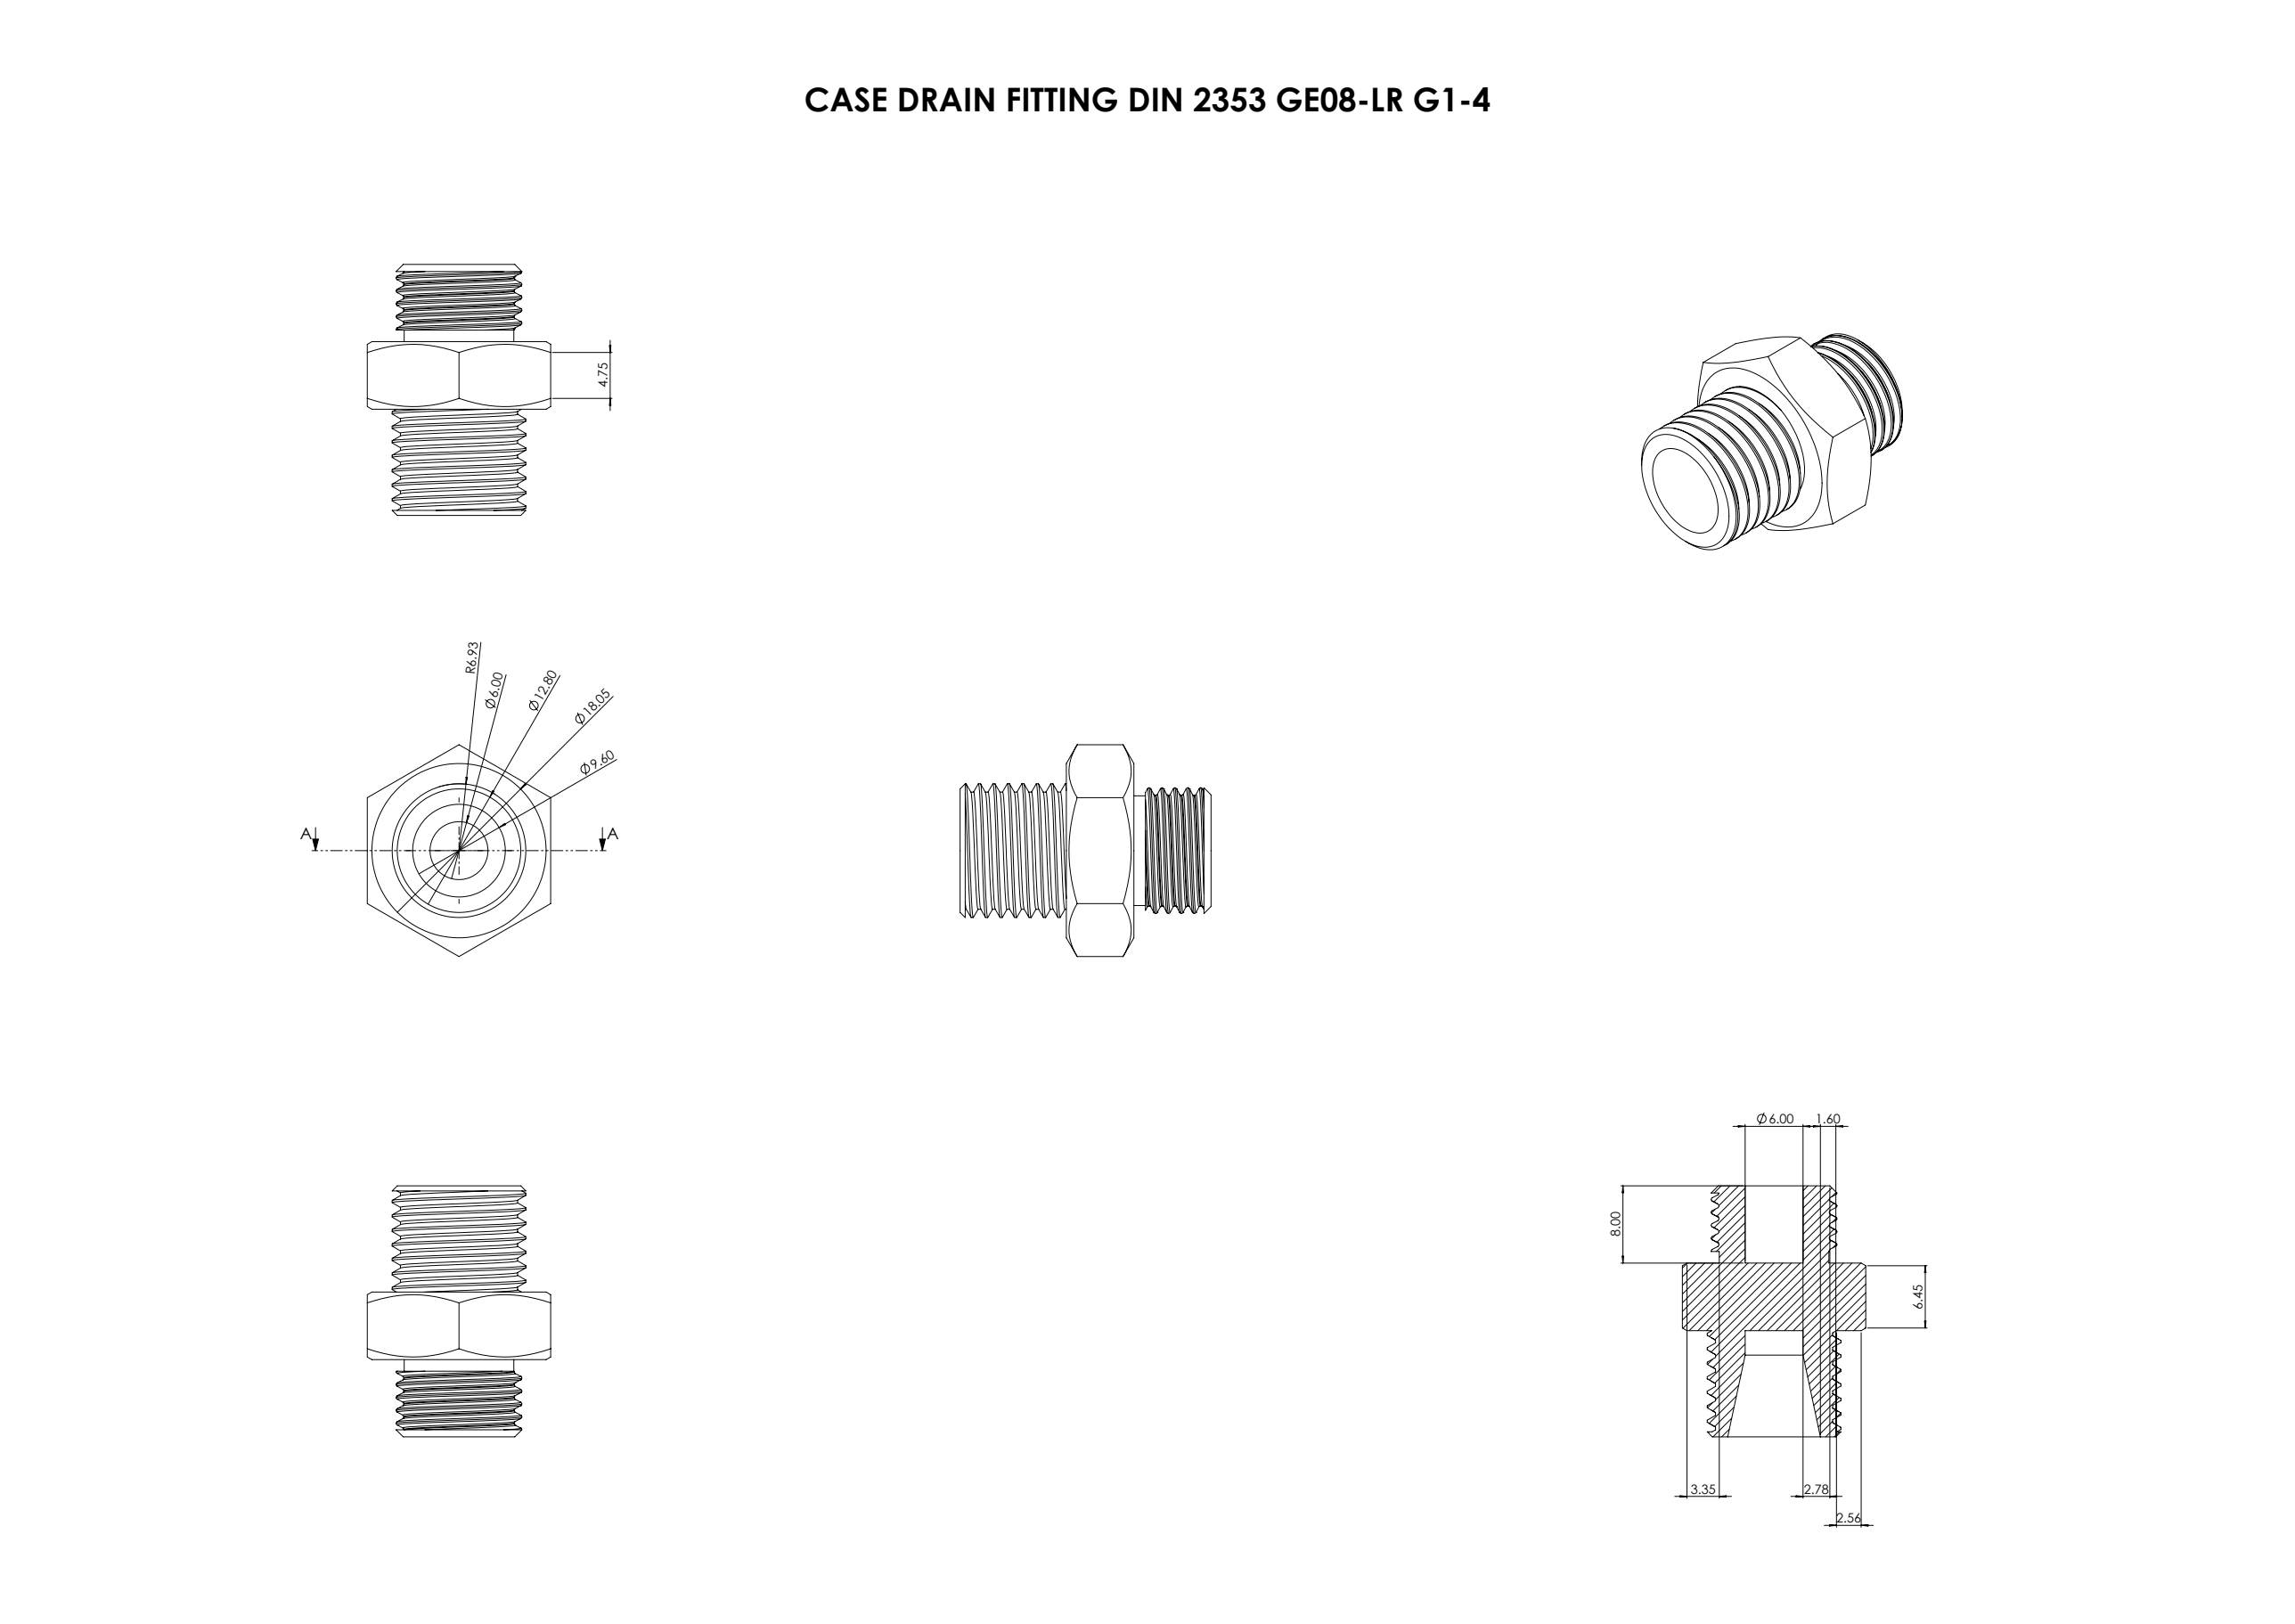
ISO-10303-21;
HEADER;
/* Generated by software containing ST-Developer
 * from STEP Tools, Inc. (www.steptools.com) 
 */

FILE_DESCRIPTION(
/* description */ (''),
/* implementation_level */ '2;1');

FILE_NAME(
/* name */ '19_Case_Drain_Fitting_DIN_2353_GE08-LR_G1-4.step',
/* time_stamp */ '2026-10-23T00:52:27+05:00',
/* author */ (''),
/* organization */ (''),
/* preprocessor_version */ 'ST-DEVELOPER v20.2',
/* originating_system */ 'Autodesk Translation Framework v15.15.0.0',
/* authorisation */ '');

FILE_SCHEMA (('AUTOMOTIVE_DESIGN { 1 0 10303 214 3 1 1 }'));
ENDSEC;

DATA;
#10=MECHANICAL_DESIGN_GEOMETRIC_PRESENTATION_REPRESENTATION('',(#1555),#59204);
#324=B_SPLINE_SURFACE_WITH_KNOTS('',3,3,((#38272,#38273,#38274,#38275,#38276,
#38277,#38278,#38279,#38280,#38281,#38282,#38283,#38284,#38285,#38286,#38287,
#38288,#38289,#38290,#38291,#38292,#38293,#38294,#38295,#38296,#38297,#38298,
#38299,#38300,#38301,#38302,#38303,#38304,#38305,#38306,#38307,#38308,#38309,
#38310,#38311,#38312,#38313,#38314,#38315,#38316,#38317,#38318,#38319,#38320,
#38321,#38322,#38323,#38324,#38325,#38326,#38327,#38328,#38329,#38330,#38331,
#38332,#38333,#38334,#38335,#38336,#38337,#38338,#38339,#38340,#38341,#38342,
#38343,#38344,#38345,#38346,#38347,#38348,#38349,#38350,#38351,#38352,#38353,
#38354,#38355,#38356,#38357,#38358,#38359,#38360,#38361,#38362,#38363,#38364,
#38365,#38366),(#38367,#38368,#38369,#38370,#38371,#38372,#38373,#38374,
#38375,#38376,#38377,#38378,#38379,#38380,#38381,#38382,#38383,#38384,#38385,
#38386,#38387,#38388,#38389,#38390,#38391,#38392,#38393,#38394,#38395,#38396,
#38397,#38398,#38399,#38400,#38401,#38402,#38403,#38404,#38405,#38406,#38407,
#38408,#38409,#38410,#38411,#38412,#38413,#38414,#38415,#38416,#38417,#38418,
#38419,#38420,#38421,#38422,#38423,#38424,#38425,#38426,#38427,#38428,#38429,
#38430,#38431,#38432,#38433,#38434,#38435,#38436,#38437,#38438,#38439,#38440,
#38441,#38442,#38443,#38444,#38445,#38446,#38447,#38448,#38449,#38450,#38451,
#38452,#38453,#38454,#38455,#38456,#38457,#38458,#38459,#38460,#38461),
(#38462,#38463,#38464,#38465,#38466,#38467,#38468,#38469,#38470,#38471,
#38472,#38473,#38474,#38475,#38476,#38477,#38478,#38479,#38480,#38481,#38482,
#38483,#38484,#38485,#38486,#38487,#38488,#38489,#38490,#38491,#38492,#38493,
#38494,#38495,#38496,#38497,#38498,#38499,#38500,#38501,#38502,#38503,#38504,
#38505,#38506,#38507,#38508,#38509,#38510,#38511,#38512,#38513,#38514,#38515,
#38516,#38517,#38518,#38519,#38520,#38521,#38522,#38523,#38524,#38525,#38526,
#38527,#38528,#38529,#38530,#38531,#38532,#38533,#38534,#38535,#38536,#38537,
#38538,#38539,#38540,#38541,#38542,#38543,#38544,#38545,#38546,#38547,#38548,
#38549,#38550,#38551,#38552,#38553,#38554,#38555,#38556),(#38557,#38558,
#38559,#38560,#38561,#38562,#38563,#38564,#38565,#38566,#38567,#38568,#38569,
#38570,#38571,#38572,#38573,#38574,#38575,#38576,#38577,#38578,#38579,#38580,
#38581,#38582,#38583,#38584,#38585,#38586,#38587,#38588,#38589,#38590,#38591,
#38592,#38593,#38594,#38595,#38596,#38597,#38598,#38599,#38600,#38601,#38602,
#38603,#38604,#38605,#38606,#38607,#38608,#38609,#38610,#38611,#38612,#38613,
#38614,#38615,#38616,#38617,#38618,#38619,#38620,#38621,#38622,#38623,#38624,
#38625,#38626,#38627,#38628,#38629,#38630,#38631,#38632,#38633,#38634,#38635,
#38636,#38637,#38638,#38639,#38640,#38641,#38642,#38643,#38644,#38645,#38646,
#38647,#38648,#38649,#38650,#38651)),.UNSPECIFIED.,.F.,.F.,.F.,(4,4),(4,
1,1,1,1,1,1,1,1,1,1,1,1,1,1,1,1,1,1,1,1,1,1,1,1,1,1,1,1,1,1,1,1,1,1,1,1,
1,1,1,1,1,1,1,1,1,1,1,1,1,1,1,1,1,1,1,1,1,1,1,1,1,1,1,1,1,1,1,1,1,1,1,1,
1,1,1,1,1,1,1,1,1,1,1,1,1,1,1,1,1,1,1,4),(0.,0.0989001011121828),(8.30505915324877,
8.80450411269543,9.30394907214209,9.80339403158876,10.3028389910354,10.8022839504821,
11.3017289099287,11.8011738693754,12.3006188288221,12.8000637882687,13.2995087477154,
13.7989537071621,14.2983986666087,14.7978436260554,15.297288585502,15.7967335449487,
16.2961785043954,16.795623463842,17.2950684232887,17.7945133827353,18.293958342182,
18.7934033016287,19.2928482610753,19.792293220522,20.2917381799687,20.7911831394153,
21.290628098862,21.7900730583086,22.2895180177553,22.788962977202,23.2884079366486,
23.7878528960953,24.287297855542,24.7867428149886,25.2861877744353,25.7856327338819,
26.2850776933286,26.7845226527753,27.2839676122219,27.7834125716686,28.2828575311152,
28.7823024905619,29.2817474500086,29.7811924094552,30.2806373689019,30.7800823283486,
31.2795272877952,31.7789722472419,32.2784172066885,32.7778621661352,33.2773071255819,
33.7767520850285,34.2761970444752,34.7756420039219,35.2750869633685,35.7745319228152,
36.2739768822618,36.7734218417085,37.2728668011552,37.7723117606018,38.2717567200485,
38.7712016794951,39.2706466389418,39.7700915983885,40.2695365578351,40.7689815172818,
41.2684264767285,41.7678714361751,42.2673163956218,42.7667613550684,43.2662063145151,
43.7656512739618,44.2650962334084,44.7645411928551,45.2639861523018,45.7634311117484,
46.2628760711951,46.7623210306417,47.2617659900884,47.7612109495351,48.2606559089817,
48.7601008684284,49.2595458278751,49.7589907873217,50.2584357467684,50.757880706215,
51.2573256656617,51.7567706251084,52.256215584555,52.7556605440017,53.2551055034483,
53.754550462895,54.2539954223417),.UNSPECIFIED.);
#325=B_SPLINE_SURFACE_WITH_KNOTS('',3,3,((#38789,#38790,#38791,#38792,#38793,
#38794,#38795,#38796,#38797,#38798,#38799,#38800,#38801,#38802,#38803,#38804,
#38805,#38806,#38807,#38808,#38809,#38810,#38811,#38812,#38813,#38814,#38815,
#38816,#38817,#38818,#38819,#38820,#38821,#38822,#38823,#38824,#38825,#38826,
#38827,#38828,#38829,#38830,#38831,#38832,#38833,#38834,#38835,#38836,#38837,
#38838,#38839,#38840,#38841,#38842,#38843,#38844,#38845,#38846,#38847,#38848,
#38849,#38850,#38851,#38852,#38853,#38854,#38855,#38856,#38857,#38858,#38859,
#38860,#38861,#38862,#38863,#38864,#38865,#38866,#38867,#38868,#38869,#38870,
#38871,#38872,#38873,#38874,#38875,#38876,#38877,#38878,#38879,#38880,#38881,
#38882,#38883),(#38884,#38885,#38886,#38887,#38888,#38889,#38890,#38891,
#38892,#38893,#38894,#38895,#38896,#38897,#38898,#38899,#38900,#38901,#38902,
#38903,#38904,#38905,#38906,#38907,#38908,#38909,#38910,#38911,#38912,#38913,
#38914,#38915,#38916,#38917,#38918,#38919,#38920,#38921,#38922,#38923,#38924,
#38925,#38926,#38927,#38928,#38929,#38930,#38931,#38932,#38933,#38934,#38935,
#38936,#38937,#38938,#38939,#38940,#38941,#38942,#38943,#38944,#38945,#38946,
#38947,#38948,#38949,#38950,#38951,#38952,#38953,#38954,#38955,#38956,#38957,
#38958,#38959,#38960,#38961,#38962,#38963,#38964,#38965,#38966,#38967,#38968,
#38969,#38970,#38971,#38972,#38973,#38974,#38975,#38976,#38977,#38978),
(#38979,#38980,#38981,#38982,#38983,#38984,#38985,#38986,#38987,#38988,
#38989,#38990,#38991,#38992,#38993,#38994,#38995,#38996,#38997,#38998,#38999,
#39000,#39001,#39002,#39003,#39004,#39005,#39006,#39007,#39008,#39009,#39010,
#39011,#39012,#39013,#39014,#39015,#39016,#39017,#39018,#39019,#39020,#39021,
#39022,#39023,#39024,#39025,#39026,#39027,#39028,#39029,#39030,#39031,#39032,
#39033,#39034,#39035,#39036,#39037,#39038,#39039,#39040,#39041,#39042,#39043,
#39044,#39045,#39046,#39047,#39048,#39049,#39050,#39051,#39052,#39053,#39054,
#39055,#39056,#39057,#39058,#39059,#39060,#39061,#39062,#39063,#39064,#39065,
#39066,#39067,#39068,#39069,#39070,#39071,#39072,#39073),(#39074,#39075,
#39076,#39077,#39078,#39079,#39080,#39081,#39082,#39083,#39084,#39085,#39086,
#39087,#39088,#39089,#39090,#39091,#39092,#39093,#39094,#39095,#39096,#39097,
#39098,#39099,#39100,#39101,#39102,#39103,#39104,#39105,#39106,#39107,#39108,
#39109,#39110,#39111,#39112,#39113,#39114,#39115,#39116,#39117,#39118,#39119,
#39120,#39121,#39122,#39123,#39124,#39125,#39126,#39127,#39128,#39129,#39130,
#39131,#39132,#39133,#39134,#39135,#39136,#39137,#39138,#39139,#39140,#39141,
#39142,#39143,#39144,#39145,#39146,#39147,#39148,#39149,#39150,#39151,#39152,
#39153,#39154,#39155,#39156,#39157,#39158,#39159,#39160,#39161,#39162,#39163,
#39164,#39165,#39166,#39167,#39168)),.UNSPECIFIED.,.F.,.F.,.F.,(4,4),(4,
1,1,1,1,1,1,1,1,1,1,1,1,1,1,1,1,1,1,1,1,1,1,1,1,1,1,1,1,1,1,1,1,1,1,1,1,
1,1,1,1,1,1,1,1,1,1,1,1,1,1,1,1,1,1,1,1,1,1,1,1,1,1,1,1,1,1,1,1,1,1,1,1,
1,1,1,1,1,1,1,1,1,1,1,1,1,1,1,1,1,1,1,4),(0.,0.0989001011121828),(11.6147305479243,
12.1141755073709,12.6136204668176,13.1130654262643,13.6125103857109,14.1119553451576,
14.6114003046042,15.1108452640509,15.6102902234976,16.1097351829442,16.6091801423909,
17.1086251018376,17.6080700612842,18.1075150207309,18.6069599801775,19.1064049396242,
19.6058498990709,20.1052948585175,20.6047398179642,21.1041847774109,21.6036297368575,
22.1030746963042,22.6025196557508,23.1019646151975,23.6014095746442,24.1008545340908,
24.6002994935375,25.0997444529841,25.5991894124308,26.0986343718775,26.5980793313241,
27.0975242907708,27.5969692502175,28.0964142096641,28.5958591691108,29.0953041285574,
29.5947490880041,30.0941940474508,30.5936390068974,31.0930839663441,31.5925289257907,
32.0919738852374,32.5914188446841,33.0908638041307,33.5903087635774,34.0897537230241,
34.5891986824707,35.0886436419174,35.588088601364,36.0875335608107,36.5869785202574,
37.086423479704,37.5858684391507,38.0853133985973,38.584758358044,39.0842033174907,
39.5836482769373,40.083093236384,40.5825381958307,41.0819831552773,41.581428114724,
42.0808730741707,42.5803180336173,43.079762993064,43.5792079525106,44.0786529119573,
44.578097871404,45.0775428308506,45.5769877902973,46.0764327497439,46.5758777091906,
47.0753226686373,47.5747676280839,48.0742125875306,48.5736575469773,49.0731025064239,
49.5725474658706,50.0719924253172,50.5714373847639,51.0708823442106,51.5703273036572,
52.0697722631039,52.5692172225505,53.0686621819972,53.5681071414439,54.0675521008905,
54.5669970603372,55.0664420197839,55.5658869792305,56.0653319386772,56.5647768981239,
57.0642218575705,57.5636668170172),.UNSPECIFIED.);
#326=B_SPLINE_SURFACE_WITH_KNOTS('',3,3,((#39272,#39273,#39274,#39275,#39276,
#39277,#39278,#39279,#39280,#39281,#39282,#39283,#39284,#39285,#39286,#39287,
#39288,#39289,#39290,#39291,#39292,#39293,#39294,#39295,#39296,#39297,#39298,
#39299,#39300,#39301,#39302,#39303,#39304,#39305,#39306,#39307,#39308,#39309,
#39310,#39311,#39312,#39313,#39314,#39315,#39316,#39317,#39318,#39319,#39320,
#39321,#39322,#39323,#39324,#39325,#39326,#39327,#39328,#39329,#39330,#39331,
#39332,#39333,#39334),(#39335,#39336,#39337,#39338,#39339,#39340,#39341,
#39342,#39343,#39344,#39345,#39346,#39347,#39348,#39349,#39350,#39351,#39352,
#39353,#39354,#39355,#39356,#39357,#39358,#39359,#39360,#39361,#39362,#39363,
#39364,#39365,#39366,#39367,#39368,#39369,#39370,#39371,#39372,#39373,#39374,
#39375,#39376,#39377,#39378,#39379,#39380,#39381,#39382,#39383,#39384,#39385,
#39386,#39387,#39388,#39389,#39390,#39391,#39392,#39393,#39394,#39395,#39396,
#39397),(#39398,#39399,#39400,#39401,#39402,#39403,#39404,#39405,#39406,
#39407,#39408,#39409,#39410,#39411,#39412,#39413,#39414,#39415,#39416,#39417,
#39418,#39419,#39420,#39421,#39422,#39423,#39424,#39425,#39426,#39427,#39428,
#39429,#39430,#39431,#39432,#39433,#39434,#39435,#39436,#39437,#39438,#39439,
#39440,#39441,#39442,#39443,#39444,#39445,#39446,#39447,#39448,#39449,#39450,
#39451,#39452,#39453,#39454,#39455,#39456,#39457,#39458,#39459,#39460),
(#39461,#39462,#39463,#39464,#39465,#39466,#39467,#39468,#39469,#39470,
#39471,#39472,#39473,#39474,#39475,#39476,#39477,#39478,#39479,#39480,#39481,
#39482,#39483,#39484,#39485,#39486,#39487,#39488,#39489,#39490,#39491,#39492,
#39493,#39494,#39495,#39496,#39497,#39498,#39499,#39500,#39501,#39502,#39503,
#39504,#39505,#39506,#39507,#39508,#39509,#39510,#39511,#39512,#39513,#39514,
#39515,#39516,#39517,#39518,#39519,#39520,#39521,#39522,#39523),(#39524,
#39525,#39526,#39527,#39528,#39529,#39530,#39531,#39532,#39533,#39534,#39535,
#39536,#39537,#39538,#39539,#39540,#39541,#39542,#39543,#39544,#39545,#39546,
#39547,#39548,#39549,#39550,#39551,#39552,#39553,#39554,#39555,#39556,#39557,
#39558,#39559,#39560,#39561,#39562,#39563,#39564,#39565,#39566,#39567,#39568,
#39569,#39570,#39571,#39572,#39573,#39574,#39575,#39576,#39577,#39578,#39579,
#39580,#39581,#39582,#39583,#39584,#39585,#39586)),.UNSPECIFIED.,.F.,.F.,
 .F.,(4,1,4),(4,1,1,1,1,1,1,1,1,1,1,1,1,1,1,1,1,1,1,1,1,1,1,1,1,1,1,1,1,
1,1,1,1,1,1,1,1,1,1,1,1,1,1,1,1,1,1,1,1,1,1,1,1,1,1,1,1,1,1,1,4),(0.,0.467498906784196,
1.09083078249646),(6.2831853071796,6.77083463049239,7.25848395380519,7.74613327711798,
8.23378260043077,8.72143192374356,9.20908124705636,9.69673057036915,10.1843798936819,
10.6720292169947,11.1596785403075,11.6473278636203,12.1349771869331,12.6226265102459,
13.1102758335587,13.5979251568715,14.0855744801843,14.5732238034971,15.0608731268099,
15.5485224501227,16.0361717734355,16.5238210967483,17.011470420061,17.4991197433738,
17.9867690666866,18.4744183899994,18.9620677133122,19.449717036625,19.9373663599378,
20.4250156832506,20.9126650065634,21.4003143298762,21.887963653189,22.3756129765018,
22.8632622998146,23.3509116231274,23.8385609464401,24.3262102697529,24.8138595930657,
25.3015089163785,25.7891582396913,26.2768075630041,26.7644568863169,27.2521062096297,
27.7397555329425,28.2274048562553,28.7150541795681,29.2027035028809,29.6903528261937,
30.1780021495065,30.6656514728192,31.153300796132,31.6409501194448,32.1285994427576,
32.6162487660704,33.1038980893832,33.591547412696,34.0791967360088,34.5668460593216,
35.0544953826344,35.5421447059472),.UNSPECIFIED.);
#327=B_SPLINE_SURFACE_WITH_KNOTS('',3,3,((#39847,#39848,#39849,#39850,#39851,
#39852,#39853,#39854,#39855,#39856,#39857,#39858,#39859,#39860,#39861,#39862,
#39863,#39864,#39865,#39866,#39867,#39868,#39869,#39870,#39871,#39872,#39873,
#39874,#39875,#39876,#39877,#39878,#39879,#39880,#39881,#39882,#39883,#39884,
#39885,#39886,#39887,#39888,#39889,#39890,#39891,#39892,#39893,#39894,#39895,
#39896,#39897,#39898,#39899,#39900,#39901,#39902,#39903,#39904,#39905,#39906,
#39907,#39908,#39909),(#39910,#39911,#39912,#39913,#39914,#39915,#39916,
#39917,#39918,#39919,#39920,#39921,#39922,#39923,#39924,#39925,#39926,#39927,
#39928,#39929,#39930,#39931,#39932,#39933,#39934,#39935,#39936,#39937,#39938,
#39939,#39940,#39941,#39942,#39943,#39944,#39945,#39946,#39947,#39948,#39949,
#39950,#39951,#39952,#39953,#39954,#39955,#39956,#39957,#39958,#39959,#39960,
#39961,#39962,#39963,#39964,#39965,#39966,#39967,#39968,#39969,#39970,#39971,
#39972),(#39973,#39974,#39975,#39976,#39977,#39978,#39979,#39980,#39981,
#39982,#39983,#39984,#39985,#39986,#39987,#39988,#39989,#39990,#39991,#39992,
#39993,#39994,#39995,#39996,#39997,#39998,#39999,#40000,#40001,#40002,#40003,
#40004,#40005,#40006,#40007,#40008,#40009,#40010,#40011,#40012,#40013,#40014,
#40015,#40016,#40017,#40018,#40019,#40020,#40021,#40022,#40023,#40024,#40025,
#40026,#40027,#40028,#40029,#40030,#40031,#40032,#40033,#40034,#40035),
(#40036,#40037,#40038,#40039,#40040,#40041,#40042,#40043,#40044,#40045,
#40046,#40047,#40048,#40049,#40050,#40051,#40052,#40053,#40054,#40055,#40056,
#40057,#40058,#40059,#40060,#40061,#40062,#40063,#40064,#40065,#40066,#40067,
#40068,#40069,#40070,#40071,#40072,#40073,#40074,#40075,#40076,#40077,#40078,
#40079,#40080,#40081,#40082,#40083,#40084,#40085,#40086,#40087,#40088,#40089,
#40090,#40091,#40092,#40093,#40094,#40095,#40096,#40097,#40098)),
 .UNSPECIFIED.,.F.,.F.,.F.,(4,4),(4,1,1,1,1,1,1,1,1,1,1,1,1,1,1,1,1,1,1,
1,1,1,1,1,1,1,1,1,1,1,1,1,1,1,1,1,1,1,1,1,1,1,1,1,1,1,1,1,1,1,1,1,1,1,1,
1,1,1,1,1,4),(0.,0.0671853436149874),(7.04827039213817,7.54746954913154,
8.0466687061249,8.54586786311827,9.04506702011163,9.54426617710499,10.0434653340984,
10.5426644910917,11.0418636480851,11.5410628050784,12.0402619620718,12.5394611190652,
13.0386602760585,13.5378594330519,14.0370585900453,14.5362577470386,15.035456904032,
15.5346560610254,16.0338552180187,16.5330543750121,17.0322535320054,17.5314526889988,
18.0306518459922,18.5298510029855,19.0290501599789,19.5282493169723,20.0274484739656,
20.526647630959,21.0258467879524,21.5250459449457,22.0242451019391,22.5234442589325,
23.0226434159258,23.5218425729192,24.0210417299125,24.5202408869059,25.0194400438993,
25.5186392008926,26.017838357886,26.5170375148794,27.0162366718727,27.5154358288661,
28.0146349858595,28.5138341428528,29.0130332998462,29.5122324568395,30.0114316138329,
30.5106307708263,31.0098299278196,31.509029084813,32.0082282418064,32.5074273987997,
33.0066265557931,33.5058257127865,34.0050248697798,34.5042240267732,35.0034231837665,
35.5026223407599,36.0018214977533,36.5010206547466,37.00021981174),
 .UNSPECIFIED.);
#328=B_SPLINE_SURFACE_WITH_KNOTS('',3,3,((#40257,#40258,#40259,#40260,#40261,
#40262,#40263,#40264,#40265,#40266,#40267,#40268,#40269,#40270,#40271,#40272,
#40273,#40274,#40275,#40276,#40277,#40278,#40279,#40280,#40281,#40282,#40283,
#40284,#40285,#40286,#40287,#40288,#40289,#40290,#40291,#40292,#40293,#40294,
#40295,#40296,#40297,#40298,#40299,#40300,#40301,#40302,#40303,#40304,#40305,
#40306,#40307,#40308,#40309,#40310,#40311,#40312,#40313,#40314,#40315,#40316,
#40317,#40318,#40319),(#40320,#40321,#40322,#40323,#40324,#40325,#40326,
#40327,#40328,#40329,#40330,#40331,#40332,#40333,#40334,#40335,#40336,#40337,
#40338,#40339,#40340,#40341,#40342,#40343,#40344,#40345,#40346,#40347,#40348,
#40349,#40350,#40351,#40352,#40353,#40354,#40355,#40356,#40357,#40358,#40359,
#40360,#40361,#40362,#40363,#40364,#40365,#40366,#40367,#40368,#40369,#40370,
#40371,#40372,#40373,#40374,#40375,#40376,#40377,#40378,#40379,#40380,#40381,
#40382),(#40383,#40384,#40385,#40386,#40387,#40388,#40389,#40390,#40391,
#40392,#40393,#40394,#40395,#40396,#40397,#40398,#40399,#40400,#40401,#40402,
#40403,#40404,#40405,#40406,#40407,#40408,#40409,#40410,#40411,#40412,#40413,
#40414,#40415,#40416,#40417,#40418,#40419,#40420,#40421,#40422,#40423,#40424,
#40425,#40426,#40427,#40428,#40429,#40430,#40431,#40432,#40433,#40434,#40435,
#40436,#40437,#40438,#40439,#40440,#40441,#40442,#40443,#40444,#40445),
(#40446,#40447,#40448,#40449,#40450,#40451,#40452,#40453,#40454,#40455,
#40456,#40457,#40458,#40459,#40460,#40461,#40462,#40463,#40464,#40465,#40466,
#40467,#40468,#40469,#40470,#40471,#40472,#40473,#40474,#40475,#40476,#40477,
#40478,#40479,#40480,#40481,#40482,#40483,#40484,#40485,#40486,#40487,#40488,
#40489,#40490,#40491,#40492,#40493,#40494,#40495,#40496,#40497,#40498,#40499,
#40500,#40501,#40502,#40503,#40504,#40505,#40506,#40507,#40508),(#40509,
#40510,#40511,#40512,#40513,#40514,#40515,#40516,#40517,#40518,#40519,#40520,
#40521,#40522,#40523,#40524,#40525,#40526,#40527,#40528,#40529,#40530,#40531,
#40532,#40533,#40534,#40535,#40536,#40537,#40538,#40539,#40540,#40541,#40542,
#40543,#40544,#40545,#40546,#40547,#40548,#40549,#40550,#40551,#40552,#40553,
#40554,#40555,#40556,#40557,#40558,#40559,#40560,#40561,#40562,#40563,#40564,
#40565,#40566,#40567,#40568,#40569,#40570,#40571)),.UNSPECIFIED.,.F.,.F.,
 .F.,(4,1,4),(4,1,1,1,1,1,1,1,1,1,1,1,1,1,1,1,1,1,1,1,1,1,1,1,1,1,1,1,1,
1,1,1,1,1,1,1,1,1,1,1,1,1,1,1,1,1,1,1,1,1,1,1,1,1,1,1,1,1,1,1,4),(0.,0.467498906784196,
1.09083078249646),(8.50634549793098,8.99399482124377,9.48164414455657,9.96929346786936,
10.4569427911822,10.9445921144949,11.4322414378077,11.9198907611205,12.4075400844333,
12.8951894077461,13.3828387310589,13.8704880543717,14.3581373776845,14.8457867009973,
15.3334360243101,15.8210853476229,16.3087346709357,16.7963839942485,17.2840333175613,
17.771682640874,18.2593319641868,18.7469812874996,19.2346306108124,19.7222799341252,
20.209929257438,20.6975785807508,21.1852279040636,21.6728772273764,22.1605265506892,
22.648175874002,23.1358251973148,23.6234745206276,24.1111238439404,24.5987731672532,
25.0864224905659,25.5740718138787,26.0617211371915,26.5493704605043,27.0370197838171,
27.5246691071299,28.0123184304427,28.4999677537555,28.9876170770683,29.4752664003811,
29.9629157236939,30.4505650470067,30.9382143703195,31.4258636936323,31.913513016945,
32.4011623402578,32.8888116635706,33.3764609868834,33.8641103101962,34.351759633509,
34.8394089568218,35.3270582801346,35.8147076034474,36.3023569267602,36.790006250073,
37.2776555733858,37.7653048966986),.UNSPECIFIED.);
#329=B_SPLINE_SURFACE_WITH_KNOTS('',3,3,((#40664,#40665,#40666,#40667,#40668,
#40669,#40670,#40671,#40672,#40673,#40674,#40675,#40676,#40677,#40678,#40679,
#40680,#40681,#40682,#40683,#40684,#40685,#40686,#40687,#40688,#40689,#40690,
#40691,#40692,#40693,#40694,#40695,#40696,#40697,#40698,#40699,#40700,#40701,
#40702,#40703,#40704,#40705,#40706,#40707,#40708,#40709,#40710,#40711,#40712,
#40713,#40714,#40715,#40716,#40717,#40718,#40719,#40720,#40721,#40722,#40723,
#40724,#40725,#40726),(#40727,#40728,#40729,#40730,#40731,#40732,#40733,
#40734,#40735,#40736,#40737,#40738,#40739,#40740,#40741,#40742,#40743,#40744,
#40745,#40746,#40747,#40748,#40749,#40750,#40751,#40752,#40753,#40754,#40755,
#40756,#40757,#40758,#40759,#40760,#40761,#40762,#40763,#40764,#40765,#40766,
#40767,#40768,#40769,#40770,#40771,#40772,#40773,#40774,#40775,#40776,#40777,
#40778,#40779,#40780,#40781,#40782,#40783,#40784,#40785,#40786,#40787,#40788,
#40789),(#40790,#40791,#40792,#40793,#40794,#40795,#40796,#40797,#40798,
#40799,#40800,#40801,#40802,#40803,#40804,#40805,#40806,#40807,#40808,#40809,
#40810,#40811,#40812,#40813,#40814,#40815,#40816,#40817,#40818,#40819,#40820,
#40821,#40822,#40823,#40824,#40825,#40826,#40827,#40828,#40829,#40830,#40831,
#40832,#40833,#40834,#40835,#40836,#40837,#40838,#40839,#40840,#40841,#40842,
#40843,#40844,#40845,#40846,#40847,#40848,#40849,#40850,#40851,#40852),
(#40853,#40854,#40855,#40856,#40857,#40858,#40859,#40860,#40861,#40862,
#40863,#40864,#40865,#40866,#40867,#40868,#40869,#40870,#40871,#40872,#40873,
#40874,#40875,#40876,#40877,#40878,#40879,#40880,#40881,#40882,#40883,#40884,
#40885,#40886,#40887,#40888,#40889,#40890,#40891,#40892,#40893,#40894,#40895,
#40896,#40897,#40898,#40899,#40900,#40901,#40902,#40903,#40904,#40905,#40906,
#40907,#40908,#40909,#40910,#40911,#40912,#40913,#40914,#40915),(#40916,
#40917,#40918,#40919,#40920,#40921,#40922,#40923,#40924,#40925,#40926,#40927,
#40928,#40929,#40930,#40931,#40932,#40933,#40934,#40935,#40936,#40937,#40938,
#40939,#40940,#40941,#40942,#40943,#40944,#40945,#40946,#40947,#40948,#40949,
#40950,#40951,#40952,#40953,#40954,#40955,#40956,#40957,#40958,#40959,#40960,
#40961,#40962,#40963,#40964,#40965,#40966,#40967,#40968,#40969,#40970,#40971,
#40972,#40973,#40974,#40975,#40976,#40977,#40978)),.UNSPECIFIED.,.F.,.F.,
 .F.,(4,1,4),(4,1,1,1,1,1,1,1,1,1,1,1,1,1,1,1,1,1,1,1,1,1,1,1,1,1,1,1,1,
1,1,1,1,1,1,1,1,1,1,1,1,1,1,1,1,1,1,1,1,1,1,1,1,1,1,1,1,1,1,1,4),(-1.09083078249646,
-0.623331875712262,0.),(9.57812533864923,10.065774661962,10.5534239852748,
11.0410733085876,11.5287226319004,12.0163719552132,12.504021278526,12.9916706018388,
13.4793199251516,13.9669692484644,14.4546185717772,14.94226789509,15.4299172184027,
15.9175665417155,16.4052158650283,16.8928651883411,17.3805145116539,17.8681638349667,
18.3558131582795,18.8434624815923,19.3311118049051,19.8187611282179,20.3064104515307,
20.7940597748435,21.2817090981563,21.7693584214691,22.2570077447818,22.7446570680946,
23.2323063914074,23.7199557147202,24.207605038033,24.6952543613458,25.1829036846586,
25.6705530079714,26.1582023312842,26.645851654597,27.1335009779098,27.6211503012226,
28.1087996245354,28.5964489478482,29.0840982711609,29.5717475944737,30.0593969177865,
30.5470462410993,31.0346955644121,31.5223448877249,32.0099942110377,32.4976435343505,
32.9852928576633,33.4729421809761,33.9605915042889,34.4482408276017,34.9358901509145,
35.4235394742273,35.91118879754,36.3988381208528,36.8864874441656,37.3741367674784,
37.8617860907912,38.349435414104,38.8370847374168),.UNSPECIFIED.);
#330=B_SPLINE_SURFACE_WITH_KNOTS('',3,3,((#41048,#41049,#41050,#41051,#41052,
#41053,#41054,#41055,#41056,#41057,#41058,#41059,#41060,#41061,#41062,#41063,
#41064,#41065,#41066,#41067,#41068,#41069,#41070,#41071,#41072,#41073,#41074,
#41075,#41076,#41077,#41078,#41079,#41080,#41081,#41082,#41083,#41084,#41085,
#41086,#41087,#41088,#41089,#41090,#41091,#41092,#41093,#41094,#41095,#41096,
#41097,#41098,#41099,#41100,#41101,#41102,#41103,#41104,#41105,#41106,#41107,
#41108,#41109,#41110),(#41111,#41112,#41113,#41114,#41115,#41116,#41117,
#41118,#41119,#41120,#41121,#41122,#41123,#41124,#41125,#41126,#41127,#41128,
#41129,#41130,#41131,#41132,#41133,#41134,#41135,#41136,#41137,#41138,#41139,
#41140,#41141,#41142,#41143,#41144,#41145,#41146,#41147,#41148,#41149,#41150,
#41151,#41152,#41153,#41154,#41155,#41156,#41157,#41158,#41159,#41160,#41161,
#41162,#41163,#41164,#41165,#41166,#41167,#41168,#41169,#41170,#41171,#41172,
#41173),(#41174,#41175,#41176,#41177,#41178,#41179,#41180,#41181,#41182,
#41183,#41184,#41185,#41186,#41187,#41188,#41189,#41190,#41191,#41192,#41193,
#41194,#41195,#41196,#41197,#41198,#41199,#41200,#41201,#41202,#41203,#41204,
#41205,#41206,#41207,#41208,#41209,#41210,#41211,#41212,#41213,#41214,#41215,
#41216,#41217,#41218,#41219,#41220,#41221,#41222,#41223,#41224,#41225,#41226,
#41227,#41228,#41229,#41230,#41231,#41232,#41233,#41234,#41235,#41236),
(#41237,#41238,#41239,#41240,#41241,#41242,#41243,#41244,#41245,#41246,
#41247,#41248,#41249,#41250,#41251,#41252,#41253,#41254,#41255,#41256,#41257,
#41258,#41259,#41260,#41261,#41262,#41263,#41264,#41265,#41266,#41267,#41268,
#41269,#41270,#41271,#41272,#41273,#41274,#41275,#41276,#41277,#41278,#41279,
#41280,#41281,#41282,#41283,#41284,#41285,#41286,#41287,#41288,#41289,#41290,
#41291,#41292,#41293,#41294,#41295,#41296,#41297,#41298,#41299)),
 .UNSPECIFIED.,.F.,.F.,.F.,(4,4),(4,1,1,1,1,1,1,1,1,1,1,1,1,1,1,1,1,1,1,
1,1,1,1,1,1,1,1,1,1,1,1,1,1,1,1,1,1,1,1,1,1,1,1,1,1,1,1,1,1,1,1,1,1,1,1,
1,1,1,1,1,4),(0.,0.0671853436149874),(10.3432104236078,10.8424095806012,
11.3416087375945,11.8408078945879,12.3400070515813,12.8392062085746,13.338405365568,
13.8376045225613,14.3368036795547,14.8360028365481,15.3352019935414,15.8344011505348,
16.3336003075282,16.8327994645215,17.3319986215149,17.8311977785083,18.3303969355016,
18.829596092495,19.3287952494883,19.8279944064817,20.3271935634751,20.8263927204684,
21.3255918774618,21.8247910344552,22.3239901914485,22.8231893484419,23.3223885054353,
23.8215876624286,24.320786819422,24.8199859764153,25.3191851334087,25.8183842904021,
26.3175834473954,26.8167826043888,27.3159817613822,27.8151809183755,28.3143800753689,
28.8135792323623,29.3127783893556,29.811977546349,30.3111767033423,30.8103758603357,
31.3095750173291,31.8087741743224,32.3079733313158,32.8071724883092,33.3063716453025,
33.8055708022959,34.3047699592893,34.8039691162826,35.303168273276,35.8023674302693,
36.3015665872627,36.8007657442561,37.2999649012494,37.7991640582428,38.2983632152362,
38.7975623722295,39.2967615292229,39.7959606862163,40.2951598432096),
 .UNSPECIFIED.);
#331=B_SPLINE_SURFACE_WITH_KNOTS('',3,3,((#41411,#41412,#41413,#41414,#41415,
#41416,#41417,#41418,#41419,#41420,#41421,#41422,#41423,#41424,#41425,#41426,
#41427,#41428,#41429,#41430,#41431,#41432,#41433,#41434,#41435,#41436,#41437,
#41438,#41439,#41440,#41441,#41442,#41443,#41444,#41445,#41446,#41447,#41448,
#41449,#41450,#41451,#41452,#41453,#41454,#41455,#41456,#41457,#41458,#41459,
#41460,#41461,#41462,#41463,#41464,#41465,#41466,#41467,#41468,#41469,#41470,
#41471,#41472,#41473),(#41474,#41475,#41476,#41477,#41478,#41479,#41480,
#41481,#41482,#41483,#41484,#41485,#41486,#41487,#41488,#41489,#41490,#41491,
#41492,#41493,#41494,#41495,#41496,#41497,#41498,#41499,#41500,#41501,#41502,
#41503,#41504,#41505,#41506,#41507,#41508,#41509,#41510,#41511,#41512,#41513,
#41514,#41515,#41516,#41517,#41518,#41519,#41520,#41521,#41522,#41523,#41524,
#41525,#41526,#41527,#41528,#41529,#41530,#41531,#41532,#41533,#41534,#41535,
#41536),(#41537,#41538,#41539,#41540,#41541,#41542,#41543,#41544,#41545,
#41546,#41547,#41548,#41549,#41550,#41551,#41552,#41553,#41554,#41555,#41556,
#41557,#41558,#41559,#41560,#41561,#41562,#41563,#41564,#41565,#41566,#41567,
#41568,#41569,#41570,#41571,#41572,#41573,#41574,#41575,#41576,#41577,#41578,
#41579,#41580,#41581,#41582,#41583,#41584,#41585,#41586,#41587,#41588,#41589,
#41590,#41591,#41592,#41593,#41594,#41595,#41596,#41597,#41598,#41599),
(#41600,#41601,#41602,#41603,#41604,#41605,#41606,#41607,#41608,#41609,
#41610,#41611,#41612,#41613,#41614,#41615,#41616,#41617,#41618,#41619,#41620,
#41621,#41622,#41623,#41624,#41625,#41626,#41627,#41628,#41629,#41630,#41631,
#41632,#41633,#41634,#41635,#41636,#41637,#41638,#41639,#41640,#41641,#41642,
#41643,#41644,#41645,#41646,#41647,#41648,#41649,#41650,#41651,#41652,#41653,
#41654,#41655,#41656,#41657,#41658,#41659,#41660,#41661,#41662),(#41663,
#41664,#41665,#41666,#41667,#41668,#41669,#41670,#41671,#41672,#41673,#41674,
#41675,#41676,#41677,#41678,#41679,#41680,#41681,#41682,#41683,#41684,#41685,
#41686,#41687,#41688,#41689,#41690,#41691,#41692,#41693,#41694,#41695,#41696,
#41697,#41698,#41699,#41700,#41701,#41702,#41703,#41704,#41705,#41706,#41707,
#41708,#41709,#41710,#41711,#41712,#41713,#41714,#41715,#41716,#41717,#41718,
#41719,#41720,#41721,#41722,#41723,#41724,#41725)),.UNSPECIFIED.,.F.,.F.,
 .F.,(4,1,4),(4,1,1,1,1,1,1,1,1,1,1,1,1,1,1,1,1,1,1,1,1,1,1,1,1,1,1,1,1,
1,1,1,1,1,1,1,1,1,1,1,1,1,1,1,1,1,1,1,1,1,1,1,1,1,1,1,1,1,1,1,4),(-1.09083078249646,
-0.623331875712262,0.),(11.8012855294006,12.2889348527134,12.7765841760262,
13.264233499339,13.7518828226518,14.2395321459646,14.7271814692774,15.2148307925902,
15.702480115903,16.1901294392157,16.6777787625285,17.1654280858413,17.6530774091541,
18.1407267324669,18.6283760557797,19.1160253790925,19.6036747024053,20.0913240257181,
20.5789733490309,21.0666226723437,21.5542719956565,22.0419213189693,22.5295706422821,
23.0172199655949,23.5048692889076,23.9925186122204,24.4801679355332,24.967817258846,
25.4554665821588,25.9431159054716,26.4307652287844,26.9184145520972,27.40606387541,
27.8937131987228,28.3813625220356,28.8690118453484,29.3566611686612,29.844310491974,
30.3319598152868,30.8196091385995,31.3072584619123,31.7949077852251,32.2825571085379,
32.7702064318507,33.2578557551635,33.7455050784763,34.2331544017891,34.7208037251019,
35.2084530484147,35.6961023717275,36.1837516950403,36.6714010183531,37.1590503416659,
37.6466996649787,38.1343489882914,38.6219983116042,39.109647634917,39.5972969582298,
40.0849462815426,40.5725956048554,41.0602449281682),.UNSPECIFIED.);
#615=B_SPLINE_CURVE_WITH_KNOTS('',3,(#37146,#37147,#37148,#37149,#37150,
#37151,#37152,#37153,#37154,#37155,#37156),.UNSPECIFIED.,.F.,.F.,(4,1,1,
1,1,1,1,1,4),(34.5575191894877,34.9358901509145,35.4235394742273,35.91118879754,
36.3988381208528,36.8864874441656,37.3741367674784,37.8617860907912,38.0719996524582),
 .UNSPECIFIED.);
#616=B_SPLINE_CURVE_WITH_KNOTS('',3,(#37159,#37160,#37161,#37162,#37163,
#37164,#37165,#37166,#37167,#37168),.UNSPECIFIED.,.F.,.F.,(4,1,1,1,1,1,
1,4),(34.5575191894877,34.8394089568218,35.3270582801346,35.8147076034474,
36.3023569267602,36.790006250073,37.2776555733858,37.7653048966986),
 .UNSPECIFIED.);
#617=B_SPLINE_CURVE_WITH_KNOTS('',3,(#37173,#37174,#37175,#37176,#37177,
#37178,#37179,#37180,#37181,#37182,#37183,#37184,#37185,#37186,#37187,#37188,
#37189),.UNSPECIFIED.,.F.,.F.,(4,1,1,1,1,1,1,1,1,1,1,1,1,1,4),(28.2743338823081,
28.5964489478482,29.0840982711609,29.5717475944737,30.0593969177865,30.5470462410993,
31.0346955644121,31.5223448877249,32.0099942110377,32.4976435343505,32.9852928576633,
33.4729421809761,33.9605915042889,34.4482408276017,34.5575191894877),
 .UNSPECIFIED.);
#618=B_SPLINE_CURVE_WITH_KNOTS('',3,(#37190,#37191,#37192,#37193,#37194,
#37195,#37196,#37197,#37198,#37199,#37200,#37201,#37202,#37203,#37204,#37205,
#37206),.UNSPECIFIED.,.F.,.F.,(4,1,1,1,1,1,1,1,1,1,1,1,1,1,4),(28.2743338823081,
28.4999677537555,28.9876170770683,29.4752664003811,29.9629157236939,30.4505650470067,
30.9382143703195,31.4258636936323,31.913513016945,32.4011623402578,32.8888116635706,
33.3764609868834,33.8641103101962,34.351759633509,34.5575191894877),
 .UNSPECIFIED.);
#619=B_SPLINE_CURVE_WITH_KNOTS('',3,(#37211,#37212,#37213,#37214,#37215,
#37216,#37217,#37218,#37219,#37220,#37221,#37222,#37223,#37224,#37225,#37226,
#37227),.UNSPECIFIED.,.F.,.F.,(4,1,1,1,1,1,1,1,1,1,1,1,1,1,4),(21.9911485751285,
22.2570077447818,22.7446570680946,23.2323063914074,23.7199557147202,24.207605038033,
24.6952543613458,25.1829036846586,25.6705530079714,26.1582023312842,26.645851654597,
27.1335009779098,27.6211503012226,28.1087996245354,28.2743338823081),
 .UNSPECIFIED.);
#620=B_SPLINE_CURVE_WITH_KNOTS('',3,(#37228,#37229,#37230,#37231,#37232,
#37233,#37234,#37235,#37236,#37237,#37238,#37239,#37240,#37241,#37242,#37243,
#37244),.UNSPECIFIED.,.F.,.F.,(4,1,1,1,1,1,1,1,1,1,1,1,1,1,4),(21.9911485751285,
22.1605265506892,22.648175874002,23.1358251973148,23.6234745206276,24.1111238439404,
24.5987731672532,25.0864224905659,25.5740718138787,26.0617211371915,26.5493704605043,
27.0370197838171,27.5246691071299,28.0123184304427,28.2743338823081),
 .UNSPECIFIED.);
#621=B_SPLINE_CURVE_WITH_KNOTS('',3,(#37249,#37250,#37251,#37252,#37253,
#37254,#37255,#37256,#37257,#37258,#37259,#37260,#37261,#37262,#37263,#37264,
#37265),.UNSPECIFIED.,.F.,.F.,(4,1,1,1,1,1,1,1,1,1,1,1,1,1,4),(15.707963267949,
15.9175665417155,16.4052158650283,16.8928651883411,17.3805145116539,17.8681638349667,
18.3558131582795,18.8434624815923,19.3311118049051,19.8187611282179,20.3064104515307,
20.7940597748435,21.2817090981563,21.7693584214691,21.9911485751285),
 .UNSPECIFIED.);
#622=B_SPLINE_CURVE_WITH_KNOTS('',3,(#37266,#37267,#37268,#37269,#37270,
#37271,#37272,#37273,#37274,#37275,#37276,#37277,#37278,#37279,#37280,#37281,
#37282),.UNSPECIFIED.,.F.,.F.,(4,1,1,1,1,1,1,1,1,1,1,1,1,1,4),(15.707963267949,
15.8210853476229,16.3087346709357,16.7963839942485,17.2840333175613,17.771682640874,
18.2593319641868,18.7469812874996,19.2346306108124,19.7222799341252,20.209929257438,
20.6975785807508,21.1852279040636,21.6728772273764,21.9911485751285),
 .UNSPECIFIED.);
#623=B_SPLINE_CURVE_WITH_KNOTS('',3,(#37289,#37290,#37291,#37292,#37293,
#37294,#37295,#37296,#37297,#37298,#37299,#37300,#37301,#37302,#37303,#37304),
 .UNSPECIFIED.,.F.,.F.,(4,1,1,1,1,1,1,1,1,1,1,1,1,4),(9.57812533864923,
10.065774661962,10.5534239852748,11.0410733085876,11.5287226319004,12.0163719552132,
12.504021278526,12.9916706018388,13.4793199251516,13.9669692484644,14.4546185717772,
14.94226789509,15.4299172184027,15.707963267949),.UNSPECIFIED.);
#624=B_SPLINE_CURVE_WITH_KNOTS('',3,(#37305,#37306,#37307,#37308,#37309,
#37310,#37311,#37312,#37313,#37314,#37315,#37316,#37317,#37318,#37319,#37320,
#37321),.UNSPECIFIED.,.F.,.F.,(4,1,1,1,1,1,1,1,1,1,1,1,1,1,4),(9.42477796076937,
9.48164414455657,9.96929346786936,10.4569427911822,10.9445921144949,11.4322414378077,
11.9198907611205,12.4075400844333,12.8951894077461,13.3828387310589,13.8704880543717,
14.3581373776845,14.8457867009973,15.3334360243101,15.707963267949),
 .UNSPECIFIED.);
#625=B_SPLINE_CURVE_WITH_KNOTS('',3,(#37327,#37328,#37329,#37330,#37331,
#37332,#37333,#37334,#37335,#37336,#37337,#37338,#37339,#37340,#37341,#37342),
 .UNSPECIFIED.,.F.,.F.,(4,3,3,3,3,4),(-4.09323272002467,-3.9955596755733,
-3.49611471612663,-2.99666975667997,-2.49722479723331,-2.07135887395548),
 .UNSPECIFIED.);
#626=B_SPLINE_CURVE_WITH_KNOTS('',3,(#37345,#37346,#37347,#37348,#37349,
#37350,#37351,#37352,#37353,#37354),.UNSPECIFIED.,.F.,.F.,(4,3,3,4),(0.,
0.499444959446661,0.998889918893321,1.11971880752059),.UNSPECIFIED.);
#627=B_SPLINE_CURVE_WITH_KNOTS('',3,(#37359,#37360,#37361,#37362,#37363,
#37364,#37365,#37366,#37367,#37368,#37369,#37370,#37371,#37372,#37373,#37374,
#37375,#37376,#37377,#37378,#37379,#37380,#37381,#37382,#37383,#37384,#37385,
#37386,#37387,#37388,#37389,#37390,#37391,#37392,#37393,#37394,#37395,#37396,
#37397,#37398),.UNSPECIFIED.,.F.,.F.,(4,3,3,3,3,3,3,3,3,3,3,3,3,4),(-10.3764180272043,
-9.98889918893324,-9.48945422948658,-8.99000927003992,-8.49056431059325,
-7.99111935114659,-7.49167439169993,-6.99222943225327,-6.49278447280661,
-5.99333951335995,-5.49389455391328,-4.99444959446662,-4.49500463501996,
-4.09323272002467),.UNSPECIFIED.);
#628=B_SPLINE_CURVE_WITH_KNOTS('',3,(#37399,#37400,#37401,#37402,#37403,
#37404,#37405,#37406,#37407,#37408,#37409,#37410,#37411,#37412,#37413,#37414,
#37415,#37416,#37417,#37418,#37419,#37420,#37421,#37422,#37423,#37424,#37425,
#37426,#37427,#37428,#37429,#37430,#37431,#37432,#37433,#37434,#37435,#37436,
#37437,#37438),.UNSPECIFIED.,.F.,.F.,(4,3,3,3,3,3,3,3,3,3,3,3,3,4),(1.11971880752059,
1.49833487833998,1.99777983778665,2.4972247972333,2.99666975667997,3.49611471612663,
3.99555967557329,4.49500463501995,4.99444959446662,5.49389455391328,5.99333951335994,
6.4927844728066,6.99222943225326,7.40290411470018),.UNSPECIFIED.);
#629=B_SPLINE_CURVE_WITH_KNOTS('',3,(#37443,#37444,#37445,#37446,#37447,
#37448,#37449,#37450,#37451,#37452,#37453,#37454,#37455,#37456,#37457,#37458,
#37459,#37460,#37461,#37462,#37463,#37464,#37465,#37466,#37467,#37468,#37469,
#37470,#37471,#37472,#37473,#37474,#37475,#37476,#37477,#37478,#37479,#37480,
#37481,#37482,#37483,#37484,#37485),.UNSPECIFIED.,.F.,.F.,(4,3,3,3,3,3,
3,3,3,3,3,3,3,3,4),(-16.6596033343838,-16.4816836617398,-15.9822387022932,
-15.4827937428465,-14.9833487833999,-14.4839038239532,-13.9844588645065,
-13.4850139050599,-12.9855689456132,-12.4861239861666,-11.9866790267199,
-11.4872340672732,-10.9877891078266,-10.4883441483799,-10.3764180272043),
 .UNSPECIFIED.);
#630=B_SPLINE_CURVE_WITH_KNOTS('',3,(#37486,#37487,#37488,#37489,#37490,
#37491,#37492,#37493,#37494,#37495,#37496,#37497,#37498,#37499,#37500,#37501,
#37502,#37503,#37504,#37505,#37506,#37507,#37508,#37509,#37510,#37511,#37512,
#37513,#37514,#37515,#37516,#37517,#37518,#37519,#37520,#37521,#37522,#37523,
#37524,#37525,#37526,#37527,#37528),.UNSPECIFIED.,.F.,.F.,(4,3,3,3,3,3,
3,3,3,3,3,3,3,3,4),(7.40290411470018,7.49167439169993,7.99111935114659,
8.49056431059325,8.99000927003991,9.48945422948658,9.98889918893324,10.4883441483799,
10.9877891078266,11.4872340672732,11.9866790267199,12.4861239861666,12.9855689456132,
13.4850139050599,13.6860894218798),.UNSPECIFIED.);
#631=B_SPLINE_CURVE_WITH_KNOTS('',3,(#37533,#37534,#37535,#37536,#37537,
#37538,#37539,#37540,#37541,#37542,#37543,#37544,#37545,#37546,#37547,#37548,
#37549,#37550,#37551,#37552,#37553,#37554,#37555,#37556,#37557,#37558,#37559,
#37560,#37561,#37562,#37563,#37564,#37565,#37566,#37567,#37568,#37569,#37570,
#37571,#37572),.UNSPECIFIED.,.F.,.F.,(4,3,3,3,3,3,3,3,3,3,3,3,3,4),(-22.9427886415634,
-22.4750231750998,-21.9755782156531,-21.4761332562065,-20.9766882967598,
-20.4772433373131,-19.9777983778665,-19.4783534184198,-18.9789084589732,
-18.4794634995265,-17.9800185400798,-17.4805735806332,-16.9811286211865,
-16.6596033343838),.UNSPECIFIED.);
#632=B_SPLINE_CURVE_WITH_KNOTS('',3,(#37573,#37574,#37575,#37576,#37577,
#37578,#37579,#37580,#37581,#37582,#37583,#37584,#37585,#37586,#37587,#37588,
#37589,#37590,#37591,#37592,#37593,#37594,#37595,#37596,#37597,#37598,#37599,
#37600,#37601,#37602,#37603,#37604,#37605,#37606,#37607,#37608,#37609,#37610,
#37611,#37612),.UNSPECIFIED.,.F.,.F.,(4,3,3,3,3,3,3,3,3,3,3,3,3,4),(13.6860894218798,
13.9844588645065,14.4839038239532,14.9833487833999,15.4827937428465,15.9822387022932,
16.4816836617398,16.9811286211865,17.4805735806332,17.9800185400798,18.4794634995265,
18.9789084589732,19.4783534184198,19.9692747290593),.UNSPECIFIED.);
#633=B_SPLINE_CURVE_WITH_KNOTS('',3,(#37617,#37618,#37619,#37620,#37621,
#37622,#37623,#37624,#37625,#37626,#37627,#37628,#37629,#37630,#37631,#37632,
#37633,#37634,#37635,#37636,#37637,#37638,#37639,#37640,#37641,#37642,#37643,
#37644,#37645,#37646,#37647,#37648,#37649,#37650,#37651,#37652,#37653,#37654,
#37655,#37656,#37657,#37658,#37659),.UNSPECIFIED.,.F.,.F.,(4,3,3,3,3,3,
3,3,3,3,3,3,3,3,4),(-29.225973948743,-28.9678076479064,-28.4683626884597,
-27.9689177290131,-27.4694727695664,-26.9700278101197,-26.4705828506731,
-25.9711378912264,-25.4716929317798,-24.9722479723331,-24.4728030128864,
-23.9733580534398,-23.4739130939931,-22.9744681345465,-22.9427886415634),
 .UNSPECIFIED.);
#634=B_SPLINE_CURVE_WITH_KNOTS('',3,(#37660,#37661,#37662,#37663,#37664,
#37665,#37666,#37667,#37668,#37669,#37670,#37671,#37672,#37673,#37674,#37675,
#37676,#37677,#37678,#37679,#37680,#37681,#37682,#37683,#37684,#37685,#37686,
#37687,#37688,#37689,#37690,#37691,#37692,#37693,#37694,#37695,#37696,#37697,
#37698,#37699,#37700,#37701,#37702),.UNSPECIFIED.,.F.,.F.,(4,3,3,3,3,3,
3,3,3,3,3,3,3,3,4),(19.9692747290593,19.9777983778665,20.4772433373131,
20.9766882967598,21.4761332562065,21.9755782156531,22.4750231750998,22.9744681345464,
23.4739130939931,23.9733580534398,24.4728030128864,24.9722479723331,25.4716929317798,
25.9711378912264,26.2524600362389),.UNSPECIFIED.);
#635=B_SPLINE_CURVE_WITH_KNOTS('',3,(#37707,#37708,#37709,#37710,#37711,
#37712,#37713,#37714,#37715,#37716,#37717,#37718,#37719,#37720,#37721,#37722,
#37723,#37724,#37725,#37726,#37727,#37728,#37729,#37730,#37731,#37732,#37733,
#37734,#37735,#37736,#37737,#37738,#37739,#37740,#37741,#37742,#37743,#37744,
#37745,#37746,#37747,#37748,#37749),.UNSPECIFIED.,.F.,.F.,(4,3,3,3,3,3,
3,3,3,3,3,3,3,3,4),(-35.5091592559226,-35.460592120713,-34.9611471612663,
-34.4617022018197,-33.962257242373,-33.4628122829264,-32.9633673234797,
-32.463922364033,-31.9644774045864,-31.4650324451397,-30.965587485693,-30.4661425262464,
-29.9666975667997,-29.4672526073531,-29.225973948743),.UNSPECIFIED.);
#636=B_SPLINE_CURVE_WITH_KNOTS('',3,(#37750,#37751,#37752,#37753,#37754,
#37755,#37756,#37757,#37758,#37759,#37760,#37761,#37762,#37763,#37764,#37765,
#37766,#37767,#37768,#37769,#37770,#37771,#37772,#37773,#37774,#37775,#37776,
#37777,#37778,#37779,#37780,#37781,#37782,#37783,#37784,#37785,#37786,#37787,
#37788,#37789,#37790,#37791,#37792),.UNSPECIFIED.,.F.,.F.,(4,3,3,3,3,3,
3,3,3,3,3,3,3,3,4),(26.2524600362389,26.4705828506731,26.9700278101197,
27.4694727695664,27.9689177290131,28.4683626884597,28.9678076479064,29.467252607353,
29.9666975667997,30.4661425262464,30.965587485693,31.4650324451397,31.9644774045864,
32.463922364033,32.5356453434185),.UNSPECIFIED.);
#637=B_SPLINE_CURVE_WITH_KNOTS('',3,(#37797,#37798,#37799,#37800,#37801,
#37802,#37803,#37804,#37805,#37806,#37807,#37808,#37809,#37810,#37811,#37812,
#37813,#37814,#37815,#37816,#37817,#37818,#37819,#37820,#37821,#37822,#37823,
#37824,#37825,#37826,#37827,#37828,#37829,#37830,#37831,#37832,#37833,#37834,
#37835,#37836),.UNSPECIFIED.,.F.,.F.,(4,3,3,3,3,3,3,3,3,3,3,3,3,4),(-41.7923445631022,
-41.453931634073,-40.9544866746263,-40.4550417151796,-39.955596755733,-39.4561517962863,
-38.9567068368396,-38.457261877393,-37.9578169179463,-37.4583719584997,
-36.958926999053,-36.4594820396063,-35.9600370801597,-35.5091592559226),
 .UNSPECIFIED.);
#638=B_SPLINE_CURVE_WITH_KNOTS('',3,(#37837,#37838,#37839,#37840,#37841,
#37842,#37843,#37844,#37845,#37846,#37847,#37848,#37849,#37850,#37851,#37852,
#37853,#37854,#37855,#37856,#37857,#37858,#37859,#37860,#37861,#37862,#37863,
#37864,#37865,#37866,#37867,#37868,#37869,#37870,#37871,#37872,#37873,#37874,
#37875,#37876),.UNSPECIFIED.,.F.,.F.,(4,3,3,3,3,3,3,3,3,3,3,3,3,4),(32.5356453434185,
32.9633673234797,33.4628122829263,33.962257242373,34.4617022018197,34.9611471612663,
35.460592120713,35.9600370801597,36.4594820396063,36.958926999053,37.4583719584996,
37.9578169179463,38.457261877393,38.8188306505981),.UNSPECIFIED.);
#639=B_SPLINE_CURVE_WITH_KNOTS('',3,(#37882,#37883,#37884,#37885,#37886,
#37887,#37888,#37889),.UNSPECIFIED.,.F.,.F.,(4,1,1,1,1,4),(53.4070751110265,
53.5681071414439,54.0675521008905,54.5669970603372,55.0664420197839,55.4923079430617),
 .UNSPECIFIED.);
#640=B_SPLINE_CURVE_WITH_KNOTS('',3,(#37892,#37893,#37894,#37895,#37896),
 .UNSPECIFIED.,.F.,.F.,(4,1,4),(53.4070751110265,53.754550462895,54.2539954223417),
 .UNSPECIFIED.);
#641=B_SPLINE_CURVE_WITH_KNOTS('',3,(#37901,#37902,#37903,#37904,#37905,
#37906,#37907,#37908,#37909,#37910,#37911,#37912,#37913,#37914,#37915,#37916),
 .UNSPECIFIED.,.F.,.F.,(4,1,1,1,1,1,1,1,1,1,1,1,1,4),(47.1238898038469,
47.5747676280839,48.0742125875306,48.5736575469773,49.0731025064239,49.5725474658706,
50.0719924253172,50.5714373847639,51.0708823442106,51.5703273036572,52.0697722631039,
52.5692172225505,53.0686621819972,53.4070751110265),.UNSPECIFIED.);
#642=B_SPLINE_CURVE_WITH_KNOTS('',3,(#37917,#37918,#37919,#37920,#37921,
#37922,#37923,#37924,#37925,#37926,#37927,#37928,#37929,#37930,#37931,#37932,
#37933),.UNSPECIFIED.,.F.,.F.,(4,1,1,1,1,1,1,1,1,1,1,1,1,1,4),(47.1238898038469,
47.2617659900884,47.7612109495351,48.2606559089817,48.7601008684284,49.2595458278751,
49.7589907873217,50.2584357467684,50.757880706215,51.2573256656617,51.7567706251084,
52.256215584555,52.7556605440017,53.2551055034483,53.4070751110265),
 .UNSPECIFIED.);
#643=B_SPLINE_CURVE_WITH_KNOTS('',3,(#37938,#37939,#37940,#37941,#37942,
#37943,#37944,#37945,#37946,#37947,#37948,#37949,#37950,#37951,#37952,#37953,
#37954),.UNSPECIFIED.,.F.,.F.,(4,1,1,1,1,1,1,1,1,1,1,1,1,1,4),(40.8407044966673,
41.0819831552773,41.581428114724,42.0808730741707,42.5803180336173,43.079762993064,
43.5792079525106,44.0786529119573,44.578097871404,45.0775428308506,45.5769877902973,
46.0764327497439,46.5758777091906,47.0753226686373,47.1238898038469),
 .UNSPECIFIED.);
#644=B_SPLINE_CURVE_WITH_KNOTS('',3,(#37955,#37956,#37957,#37958,#37959,
#37960,#37961,#37962,#37963,#37964,#37965,#37966,#37967,#37968,#37969,#37970),
 .UNSPECIFIED.,.F.,.F.,(4,1,1,1,1,1,1,1,1,1,1,1,1,4),(40.8407044966673,
41.2684264767285,41.7678714361751,42.2673163956218,42.7667613550684,43.2662063145151,
43.7656512739618,44.2650962334084,44.7645411928551,45.2639861523018,45.7634311117484,
46.2628760711951,46.7623210306417,47.1238898038469),.UNSPECIFIED.);
#645=B_SPLINE_CURVE_WITH_KNOTS('',3,(#37975,#37976,#37977,#37978,#37979,
#37980,#37981,#37982,#37983,#37984,#37985,#37986,#37987,#37988,#37989,#37990,
#37991),.UNSPECIFIED.,.F.,.F.,(4,1,1,1,1,1,1,1,1,1,1,1,1,1,4),(34.5575191894877,
34.5891986824707,35.0886436419174,35.588088601364,36.0875335608107,36.5869785202574,
37.086423479704,37.5858684391507,38.0853133985973,38.584758358044,39.0842033174907,
39.5836482769373,40.083093236384,40.5825381958307,40.8407044966673),
 .UNSPECIFIED.);
#646=B_SPLINE_CURVE_WITH_KNOTS('',3,(#37992,#37993,#37994,#37995,#37996,
#37997,#37998,#37999,#38000,#38001,#38002,#38003,#38004,#38005,#38006,#38007,
#38008),.UNSPECIFIED.,.F.,.F.,(4,1,1,1,1,1,1,1,1,1,1,1,1,1,4),(34.5575191894877,
34.7756420039219,35.2750869633685,35.7745319228152,36.2739768822618,36.7734218417085,
37.2728668011552,37.7723117606018,38.2717567200485,38.7712016794951,39.2706466389418,
39.7700915983885,40.2695365578351,40.7689815172818,40.8407044966673),
 .UNSPECIFIED.);
#647=B_SPLINE_CURVE_WITH_KNOTS('',3,(#38013,#38014,#38015,#38016,#38017,
#38018,#38019,#38020,#38021,#38022,#38023,#38024,#38025,#38026,#38027,#38028),
 .UNSPECIFIED.,.F.,.F.,(4,1,1,1,1,1,1,1,1,1,1,1,1,4),(28.2743338823081,
28.5958591691108,29.0953041285574,29.5947490880041,30.0941940474508,30.5936390068974,
31.0930839663441,31.5925289257907,32.0919738852374,32.5914188446841,33.0908638041307,
33.5903087635774,34.0897537230241,34.5575191894877),.UNSPECIFIED.);
#648=B_SPLINE_CURVE_WITH_KNOTS('',3,(#38029,#38030,#38031,#38032,#38033,
#38034,#38035,#38036,#38037,#38038,#38039,#38040,#38041,#38042,#38043,#38044,
#38045),.UNSPECIFIED.,.F.,.F.,(4,1,1,1,1,1,1,1,1,1,1,1,1,1,4),(28.2743338823081,
28.2828575311152,28.7823024905619,29.2817474500086,29.7811924094552,30.2806373689019,
30.7800823283486,31.2795272877952,31.7789722472419,32.2784172066885,32.7778621661352,
33.2773071255819,33.7767520850285,34.2761970444752,34.5575191894877),
 .UNSPECIFIED.);
#649=B_SPLINE_CURVE_WITH_KNOTS('',3,(#38050,#38051,#38052,#38053,#38054,
#38055,#38056,#38057,#38058,#38059,#38060,#38061,#38062,#38063,#38064,#38065,
#38066),.UNSPECIFIED.,.F.,.F.,(4,1,1,1,1,1,1,1,1,1,1,1,1,1,4),(21.9911485751285,
22.1030746963042,22.6025196557508,23.1019646151975,23.6014095746442,24.1008545340908,
24.6002994935375,25.0997444529841,25.5991894124308,26.0986343718775,26.5980793313241,
27.0975242907708,27.5969692502175,28.0964142096641,28.2743338823081),
 .UNSPECIFIED.);
#650=B_SPLINE_CURVE_WITH_KNOTS('',3,(#38067,#38068,#38069,#38070,#38071,
#38072,#38073,#38074,#38075,#38076,#38077,#38078,#38079,#38080,#38081,#38082),
 .UNSPECIFIED.,.F.,.F.,(4,1,1,1,1,1,1,1,1,1,1,1,1,4),(21.9911485751285,
22.2895180177553,22.788962977202,23.2884079366486,23.7878528960953,24.287297855542,
24.7867428149886,25.2861877744353,25.7856327338819,26.2850776933286,26.7845226527753,
27.2839676122219,27.7834125716686,28.2743338823081),.UNSPECIFIED.);
#651=B_SPLINE_CURVE_WITH_KNOTS('',3,(#38087,#38088,#38089,#38090,#38091,
#38092,#38093,#38094,#38095,#38096,#38097,#38098,#38099,#38100,#38101,#38102),
 .UNSPECIFIED.,.F.,.F.,(4,1,1,1,1,1,1,1,1,1,1,1,1,4),(15.7079632679489,
16.1097351829442,16.6091801423909,17.1086251018376,17.6080700612842,18.1075150207309,
18.6069599801775,19.1064049396242,19.6058498990709,20.1052948585175,20.6047398179642,
21.1041847774109,21.6036297368575,21.9911485751285),.UNSPECIFIED.);
#652=B_SPLINE_CURVE_WITH_KNOTS('',3,(#38103,#38104,#38105,#38106,#38107,
#38108,#38109,#38110,#38111,#38112,#38113,#38114,#38115,#38116,#38117,#38118,
#38119),.UNSPECIFIED.,.F.,.F.,(4,1,1,1,1,1,1,1,1,1,1,1,1,1,4),(15.7079632679489,
15.7967335449487,16.2961785043954,16.795623463842,17.2950684232887,17.7945133827353,
18.293958342182,18.7934033016287,19.2928482610753,19.792293220522,20.2917381799687,
20.7911831394153,21.290628098862,21.7900730583086,21.9911485751285),
 .UNSPECIFIED.);
#653=B_SPLINE_CURVE_WITH_KNOTS('',3,(#38122,#38123,#38124,#38125,#38126,
#38127,#38128,#38129,#38130,#38131,#38132,#38133,#38134,#38135,#38136,#38137,
#38138,#38139,#38140,#38141,#38142,#38143,#38144,#38145,#38146,#38147,#38148,
#38149,#38150,#38151,#38152,#38153,#38154,#38155,#38156,#38157,#38158,#38159,
#38160,#38161,#38162,#38163,#38164,#38165,#38166,#38167,#38168,#38169,#38170,
#38171,#38172,#38173,#38174,#38175,#38176,#38177,#38178,#38179,#38180,#38181,
#38182,#38183,#38184,#38185,#38186,#38187,#38188,#38189,#38190,#38191,#38192,
#38193,#38194),.UNSPECIFIED.,.F.,.F.,(4,3,3,3,3,3,3,3,3,3,3,3,3,3,3,3,3,
3,3,3,3,3,3,3,4),(-1.35394557174001,-1.30892768444359,-1.23102926805986,
-1.19688794819057,-1.17004272714157,-1.08368837302513,-1.04606736794041,
-1.01553569614099,-0.997334018908685,-0.903275013057271,-0.840846396492717,
-0.792075238959429,-0.767723825473952,-0.674993002634861,-0.591861111789504,
-0.541890483864056,-0.513413628060138,-0.415103168314629,-0.342465439253432,
-0.295139204862908,-0.267683354098771,-0.246657321726534,-0.147343803841858,
-0.0476021900320448,0.),.UNSPECIFIED.);
#654=B_SPLINE_CURVE_WITH_KNOTS('',3,(#38199,#38200,#38201,#38202,#38203,
#38204,#38205,#38206,#38207,#38208,#38209,#38210,#38211,#38212,#38213,#38214,
#38215,#38216,#38217,#38218,#38219,#38220,#38221,#38222,#38223,#38224,#38225,
#38226,#38227,#38228,#38229,#38230,#38231,#38232,#38233,#38234,#38235,#38236,
#38237,#38238,#38239,#38240,#38241,#38242,#38243,#38244,#38245,#38246,#38247,
#38248,#38249,#38250,#38251,#38252,#38253,#38254,#38255,#38256,#38257,#38258,
#38259,#38260,#38261,#38262,#38263,#38264,#38265,#38266,#38267,#38268,#38269,
#38270,#38271),.UNSPECIFIED.,.F.,.F.,(4,3,3,3,3,3,3,3,3,3,3,3,3,3,3,3,3,
3,3,3,3,3,3,3,4),(-1.3501974997237,-1.29933842216202,-1.21445175298089,
-1.17996490551909,-1.15395803466285,-1.05687489005017,-0.995259379032231,
-0.973262385119946,-0.959791745437487,-0.862294128942176,-0.765592015437111,
-0.740849630173425,-0.722135556856507,-0.62974877054122,-0.549747247506987,
-0.504760312423779,-0.483247297343189,-0.389544187887911,-0.30974267840429,
-0.263847143486886,-0.242838513083088,-0.223579745215157,-0.131366862398016,
-0.0408081318941806,0.),.UNSPECIFIED.);
#655=B_SPLINE_CURVE_WITH_KNOTS('',3,(#38652,#38653,#38654,#38655,#38656,
#38657,#38658,#38659,#38660,#38661,#38662,#38663,#38664,#38665,#38666,#38667,
#38668,#38669,#38670,#38671,#38672,#38673,#38674,#38675,#38676,#38677,#38678,
#38679,#38680,#38681,#38682,#38683,#38684,#38685),.UNSPECIFIED.,.F.,.F.,
(4,3,3,3,3,3,3,3,3,3,3,4),(38.8188306505981,38.9567068368396,39.4561517962863,
39.955596755733,40.4550417151796,40.9544866746263,41.4539316340729,41.9533765935196,
42.4528215529663,42.9522665124129,43.4517114718596,43.8775773951374),
 .UNSPECIFIED.);
#656=B_SPLINE_CURVE_WITH_KNOTS('',3,(#38687,#38688,#38689,#38690,#38691,
#38692,#38693,#38694,#38695,#38696,#38697,#38698,#38699,#38700,#38701,#38702,
#38703,#38704,#38705,#38706,#38707,#38708,#38709,#38710,#38711,#38712,#38713,
#38714,#38715,#38716,#38717,#38718,#38719,#38720,#38721,#38722,#38723,#38724,
#38725,#38726,#38727,#38728,#38729,#38730,#38731,#38732,#38733,#38734,#38735,
#38736,#38737,#38738,#38739,#38740,#38741,#38742,#38743,#38744,#38745,#38746,
#38747,#38748,#38749,#38750,#38751,#38752,#38753,#38754,#38755,#38756,#38757,
#38758,#38759),.UNSPECIFIED.,.F.,.F.,(4,3,3,3,3,3,3,3,3,3,3,3,3,3,3,3,3,
3,3,3,3,3,3,3,4),(-1.35394557173993,-1.3089276844435,-1.23102926805979,
-1.19688793436548,-1.17004272418587,-1.08368837154726,-1.04606737005723,
-1.01553569577731,-0.997334018908637,-0.903275019134099,-0.840846379666836,
-0.792075216486473,-0.767723818900745,-0.674993002634844,-0.591861111789487,
-0.5418904765301,-0.513413625146155,-0.415103169643614,-0.342465439253416,
-0.295139212184705,-0.267683438959337,-0.246657340266153,-0.14734376022256,
-0.0476021992245664,0.),.UNSPECIFIED.);
#657=B_SPLINE_CURVE_WITH_KNOTS('',3,(#38760,#38761,#38762,#38763,#38764,
#38765,#38766,#38767,#38768,#38769,#38770,#38771,#38772,#38773),
 .UNSPECIFIED.,.F.,.F.,(4,1,1,1,1,1,1,1,1,1,1,4),(10.3764180272042,10.8022839504821,
11.3017289099287,11.8011738693754,12.3006188288221,12.8000637882687,13.2995087477154,
13.7989537071621,14.2983986666087,14.7978436260554,15.297288585502,15.7079632679489),
 .UNSPECIFIED.);
#658=B_SPLINE_CURVE_WITH_KNOTS('',3,(#38777,#38778,#38779,#38780,#38781,
#38782,#38783,#38784,#38785,#38786,#38787,#38788),.UNSPECIFIED.,.F.,.F.,
(4,1,1,1,1,1,1,1,1,4),(11.6147305479243,12.1141755073709,12.6136204668176,
13.1130654262643,13.6125103857109,14.1119553451576,14.6114003046042,15.1108452640509,
15.6102902234976,15.7079632679489),.UNSPECIFIED.);
#659=B_SPLINE_CURVE_WITH_KNOTS('',3,(#39169,#39170,#39171,#39172,#39173,
#39174,#39175,#39176,#39177,#39178,#39179,#39180,#39181,#39182,#39183,#39184,
#39185,#39186,#39187,#39188,#39189,#39190,#39191,#39192,#39193,#39194,#39195,
#39196,#39197,#39198,#39199,#39200,#39201,#39202,#39203,#39204,#39205,#39206,
#39207,#39208,#39209,#39210,#39211,#39212,#39213,#39214,#39215,#39216,#39217,
#39218,#39219,#39220,#39221,#39222,#39223,#39224,#39225,#39226,#39227,#39228,
#39229,#39230,#39231,#39232,#39233,#39234,#39235,#39236,#39237,#39238,#39239,
#39240,#39241),.UNSPECIFIED.,.F.,.F.,(4,3,3,3,3,3,3,3,3,3,3,3,3,3,3,3,3,
3,3,3,3,3,3,3,4),(-1.35019749972372,-1.29933842216204,-1.2144517529809,
-1.1799649098461,-1.15395803765335,-1.05687489154542,-0.995259377759728,
-0.973262384530162,-0.959791745437486,-0.862294124972048,-0.765591977626827,
-0.740849464395243,-0.722135242327674,-0.629748770541223,-0.549747247506988,
-0.5047603153859,-0.483247294935022,-0.389544230430759,-0.309742678404285,
-0.263847165242411,-0.242838634274085,-0.223579987122219,-0.131367108976752,
-0.0408082650079221,0.),.UNSPECIFIED.);
#660=B_SPLINE_CURVE_WITH_KNOTS('',3,(#39242,#39243,#39244,#39245,#39246,
#39247,#39248,#39249,#39250,#39251,#39252,#39253,#39254,#39255,#39256,#39257,
#39258,#39259,#39260,#39261,#39262,#39263,#39264,#39265,#39266,#39267,#39268,
#39269),.UNSPECIFIED.,.F.,.F.,(4,3,3,3,3,3,3,3,3,4),(-45.9489362690929,
-45.4494913096462,-44.9500463501996,-44.4506013907529,-43.9511564313063,
-43.4517114718596,-42.9522665124129,-42.4528215529663,-41.9533765935196,
-41.7923445631022),.UNSPECIFIED.);
#661=B_SPLINE_CURVE_WITH_KNOTS('',3,(#39589,#39590,#39591,#39592,#39593,
#39594,#39595,#39596),.UNSPECIFIED.,.F.,.F.,(4,2,2,4),(0.,0.237315706087857,
0.388427486543153,0.517252919461271),.UNSPECIFIED.);
#662=B_SPLINE_CURVE_WITH_KNOTS('',3,(#39598,#39599,#39600,#39601,#39602,
#39603,#39604,#39605,#39606,#39607,#39608,#39609,#39610,#39611,#39612,#39613,
#39614,#39615,#39616,#39617,#39618,#39619,#39620,#39621,#39622,#39623,#39624,
#39625,#39626,#39627,#39628,#39629,#39630,#39631,#39632,#39633,#39634,#39635,
#39636,#39637,#39638,#39639,#39640,#39641,#39642,#39643,#39644,#39645,#39646,
#39647,#39648,#39649,#39650,#39651,#39652,#39653,#39654,#39655,#39656,#39657,
#39658,#39659,#39660,#39661,#39662,#39663,#39664,#39665,#39666,#39667,#39668,
#39669,#39670,#39671,#39672,#39673,#39674,#39675,#39676,#39677,#39678,#39679,
#39680,#39681,#39682,#39683,#39684,#39685,#39686,#39687,#39688,#39689,#39690,
#39691,#39692,#39693,#39694,#39695,#39696,#39697,#39698,#39699,#39700,#39701,
#39702,#39703,#39704,#39705,#39706,#39707,#39708,#39709,#39710,#39711,#39712,
#39713,#39714,#39715,#39716,#39717,#39718,#39719,#39720,#39721,#39722,#39723,
#39724,#39725,#39726,#39727,#39728,#39729,#39730,#39731,#39732,#39733,#39734,
#39735,#39736,#39737,#39738,#39739,#39740,#39741,#39742,#39743,#39744,#39745,
#39746,#39747,#39748,#39749,#39750,#39751,#39752,#39753,#39754,#39755,#39756,
#39757,#39758,#39759,#39760,#39761,#39762,#39763,#39764,#39765,#39766,#39767,
#39768,#39769,#39770,#39771,#39772,#39773,#39774,#39775),.UNSPECIFIED.,
 .F.,.F.,(4,3,3,3,3,3,3,3,3,3,3,3,3,3,3,3,3,3,3,3,3,3,3,3,3,3,3,3,3,3,3,
3,3,3,3,3,3,3,3,3,3,3,3,3,3,3,3,3,3,3,3,3,3,3,3,3,3,3,3,4),(0.,0.487649323312794,
0.975298646625587,1.46294796993838,1.95059729325117,2.43824661656396,2.92589593987676,
3.41354526318955,3.90119458650234,4.38884390981513,4.87649323312793,5.36414255644072,
5.85179187975351,6.33944120306631,6.8270905263791,7.31473984969189,7.80238917300469,
8.29003849631748,8.77768781963027,9.26533714294306,9.75298646625586,10.2406357895687,
10.7282851128814,11.2159344361942,11.703583759507,12.1912330828198,12.6788824061326,
13.1665317294454,13.6541810527582,14.141830376071,14.6294796993838,15.1171290226966,
15.6047783460094,16.0924276693222,16.580076992635,17.0677263159478,17.5553756392605,
18.0430249625733,18.5306742858861,19.0183236091989,19.5059729325117,19.9936222558245,
20.4812715791373,20.9689209024501,21.4565702257629,21.9442195490757,22.4318688723885,
22.9195181957013,23.4071675190141,23.8948168423269,24.3824661656396,24.8701154889524,
25.3577648122652,25.845414135578,26.3330634588908,26.8207127822036,27.3083621055164,
27.7960114288292,28.283660752142,28.493874313809),.UNSPECIFIED.);
#663=B_SPLINE_CURVE_WITH_KNOTS('',3,(#39777,#39778,#39779,#39780,#39781,
#39782,#39783,#39784),.UNSPECIFIED.,.F.,.F.,(4,2,2,4),(-0.517251340629339,
-0.388433724430474,-0.237311387866167,0.),.UNSPECIFIED.);
#664=B_SPLINE_CURVE_WITH_KNOTS('',3,(#39785,#39786,#39787,#39788,#39789,
#39790,#39791,#39792,#39793,#39794,#39795,#39796,#39797,#39798,#39799,#39800,
#39801,#39802,#39803,#39804,#39805,#39806,#39807,#39808,#39809,#39810,#39811,
#39812,#39813,#39814,#39815,#39816,#39817,#39818,#39819,#39820,#39821,#39822,
#39823,#39824,#39825,#39826,#39827,#39828,#39829,#39830,#39831,#39832,#39833,
#39834,#39835,#39836,#39837,#39838,#39839,#39840,#39841,#39842,#39843,#39844,
#39845,#39846),.UNSPECIFIED.,.F.,.F.,(4,1,1,1,1,1,1,1,1,1,1,1,1,1,1,1,1,
1,1,1,1,1,1,1,1,1,1,1,1,1,1,1,1,1,1,1,1,1,1,1,1,1,1,1,1,1,1,1,1,1,1,1,1,
1,1,1,1,1,1,4),(7.04827039213818,7.25848395380519,7.74613327711798,8.23378260043077,
8.72143192374356,9.20908124705636,9.69673057036915,10.1843798936819,10.6720292169947,
11.1596785403075,11.6473278636203,12.1349771869331,12.6226265102459,13.1102758335587,
13.5979251568715,14.0855744801843,14.5732238034971,15.0608731268099,15.5485224501227,
16.0361717734355,16.5238210967483,17.011470420061,17.4991197433738,17.9867690666866,
18.4744183899994,18.9620677133122,19.449717036625,19.9373663599378,20.4250156832506,
20.9126650065634,21.4003143298762,21.887963653189,22.3756129765018,22.8632622998146,
23.3509116231274,23.8385609464401,24.3262102697529,24.8138595930657,25.3015089163785,
25.7891582396913,26.2768075630041,26.7644568863169,27.2521062096297,27.7397555329425,
28.2274048562553,28.7150541795681,29.2027035028809,29.6903528261937,30.1780021495065,
30.6656514728192,31.153300796132,31.6409501194448,32.1285994427576,32.6162487660704,
33.1038980893832,33.591547412696,34.0791967360088,34.5668460593216,35.0544953826344,
35.5421447059472),.UNSPECIFIED.);
#665=B_SPLINE_CURVE_WITH_KNOTS('',3,(#40100,#40101,#40102,#40103,#40104,
#40105,#40106,#40107,#40108,#40109,#40110,#40111,#40112,#40113,#40114,#40115,
#40116,#40117,#40118,#40119,#40120,#40121,#40122,#40123,#40124,#40125,#40126,
#40127,#40128,#40129,#40130,#40131,#40132,#40133,#40134,#40135,#40136,#40137,
#40138,#40139,#40140,#40141,#40142,#40143,#40144,#40145),.UNSPECIFIED.,
 .F.,.F.,(4,3,3,3,3,3,3,3,3,3,3,3,3,3,3,4),(0.,0.0942991010737542,0.193262215210111,
0.237548070776078,0.261597840086782,0.292225329346469,0.384931640470592,
0.454115017893606,0.485075070504274,0.504919783104731,0.600066451276272,
0.674462382718296,0.696928463272835,0.786359577028978,0.874195006668787,
0.897650177044366),.UNSPECIFIED.);
#666=B_SPLINE_CURVE_WITH_KNOTS('',3,(#40147,#40148,#40149,#40150,#40151,
#40152,#40153,#40154,#40155,#40156,#40157,#40158,#40159,#40160,#40161,#40162,
#40163,#40164,#40165,#40166,#40167,#40168,#40169,#40170,#40171,#40172,#40173,
#40174,#40175,#40176,#40177,#40178,#40179,#40180,#40181,#40182,#40183,#40184,
#40185,#40186,#40187,#40188,#40189,#40190,#40191,#40192,#40193,#40194,#40195),
 .UNSPECIFIED.,.F.,.F.,(4,3,3,3,3,3,3,3,3,3,3,3,3,3,3,3,4),(-0.897650177044365,
-0.809221996292059,-0.716620361820245,-0.696324645029017,-0.674917979597778,
-0.624018727348431,-0.547256284732747,-0.495744435273601,-0.47451926273118,
-0.381889608747681,-0.316968956885692,-0.2713446547458,-0.249438014013973,
-0.22789468603582,-0.134228551311836,-0.0401158448815296,0.),
 .UNSPECIFIED.);
#667=B_SPLINE_CURVE_WITH_KNOTS('',3,(#40196,#40197,#40198,#40199,#40200,
#40201,#40202,#40203,#40204,#40205,#40206,#40207,#40208,#40209,#40210,#40211,
#40212,#40213,#40214,#40215,#40216,#40217,#40218,#40219,#40220,#40221,#40222,
#40223,#40224,#40225,#40226,#40227,#40228,#40229,#40230,#40231,#40232,#40233,
#40234,#40235,#40236,#40237,#40238,#40239,#40240,#40241,#40242,#40243,#40244,
#40245,#40246,#40247,#40248,#40249,#40250,#40251,#40252,#40253,#40254,#40255,
#40256),.UNSPECIFIED.,.F.,.F.,(4,1,1,1,1,1,1,1,1,1,1,1,1,1,1,1,1,1,1,1,
1,1,1,1,1,1,1,1,1,1,1,1,1,1,1,1,1,1,1,1,1,1,1,1,1,1,1,1,1,1,1,1,1,1,1,1,
1,1,4),(8.50634549793098,8.54586786311827,9.04506702011163,9.54426617710499,
10.0434653340984,10.5426644910917,11.0418636480851,11.5410628050784,12.0402619620718,
12.5394611190652,13.0386602760585,13.5378594330519,14.0370585900453,14.5362577470386,
15.035456904032,15.5346560610254,16.0338552180187,16.5330543750121,17.0322535320054,
17.5314526889988,18.0306518459922,18.5298510029855,19.0290501599789,19.5282493169723,
20.0274484739656,20.526647630959,21.0258467879524,21.5250459449457,22.0242451019391,
22.5234442589325,23.0226434159258,23.5218425729192,24.0210417299125,24.5202408869059,
25.0194400438993,25.5186392008926,26.017838357886,26.5170375148794,27.0162366718727,
27.5154358288661,28.0146349858595,28.5138341428528,29.0130332998462,29.5122324568395,
30.0114316138329,30.5106307708263,31.0098299278196,31.509029084813,32.0082282418064,
32.5074273987997,33.0066265557931,33.5058257127865,34.0050248697798,34.5042240267732,
35.0034231837665,35.5026223407599,36.0018214977533,36.5010206547466,37.00021981174),
 .UNSPECIFIED.);
#668=B_SPLINE_CURVE_WITH_KNOTS('',3,(#40572,#40573,#40574,#40575,#40576,
#40577,#40578,#40579),.UNSPECIFIED.,.F.,.F.,(4,2,2,4),(0.,0.129325009251138,
0.19845452791459,0.272929378090483),.UNSPECIFIED.);
#669=B_SPLINE_CURVE_WITH_KNOTS('',3,(#40581,#40582,#40583,#40584,#40585,
#40586,#40587,#40588),.UNSPECIFIED.,.F.,.F.,(4,2,2,4),(-0.272903900599443,
-0.198454240786918,-0.129349013127501,0.),.UNSPECIFIED.);
#670=B_SPLINE_CURVE_WITH_KNOTS('',3,(#40589,#40590,#40591,#40592),
 .UNSPECIFIED.,.F.,.F.,(4,4),(9.27143058288956,9.42477796076937),
 .UNSPECIFIED.);
#671=B_SPLINE_CURVE_WITH_KNOTS('',3,(#40598,#40599,#40600,#40601,#40602,
#40603,#40604,#40605),.UNSPECIFIED.,.F.,.F.,(4,2,2,4),(-0.322073238962409,
-0.232715827739448,-0.150125558909819,0.),.UNSPECIFIED.);
#672=B_SPLINE_CURVE_WITH_KNOTS('',3,(#40607,#40608,#40609,#40610,#40611,
#40612,#40613,#40614,#40615,#40616,#40617,#40618,#40619,#40620,#40621,#40622,
#40623,#40624,#40625,#40626,#40627,#40628,#40629,#40630,#40631,#40632,#40633,
#40634,#40635,#40636,#40637,#40638,#40639,#40640,#40641,#40642,#40643,#40644,
#40645,#40646,#40647,#40648,#40649,#40650,#40651,#40652,#40653,#40654,#40655),
 .UNSPECIFIED.,.F.,.F.,(4,3,3,3,3,3,3,3,3,3,3,3,3,3,3,3,4),(-0.89585384003955,
-0.801561846631882,-0.702966153173172,-0.678976633753644,-0.657477299216225,
-0.604370459714462,-0.527568764985274,-0.481321993461353,-0.451377108901128,
-0.36059738503407,-0.297163680797711,-0.25214599148876,-0.230319865611295,
-0.210822177973724,-0.121429520577694,-0.0337496836487225,0.),
 .UNSPECIFIED.);
#673=B_SPLINE_CURVE_WITH_KNOTS('',3,(#40656,#40657,#40658,#40659,#40660,
#40661),.UNSPECIFIED.,.F.,.F.,(4,2,4),(-0.500559801427663,-0.225408038500461,
0.),.UNSPECIFIED.);
#674=B_SPLINE_CURVE_WITH_KNOTS('',3,(#40980,#40981,#40982,#40983,#40984,
#40985),.UNSPECIFIED.,.F.,.F.,(4,2,4),(0.,0.225412734088363,0.500557798157366),
 .UNSPECIFIED.);
#675=B_SPLINE_CURVE_WITH_KNOTS('',3,(#40986,#40987,#40988,#40989,#40990,
#40991,#40992,#40993,#40994,#40995,#40996,#40997,#40998,#40999,#41000,#41001,
#41002,#41003,#41004,#41005,#41006,#41007,#41008,#41009,#41010,#41011,#41012,
#41013,#41014,#41015,#41016,#41017,#41018,#41019,#41020,#41021,#41022,#41023,
#41024,#41025,#41026,#41027,#41028,#41029,#41030,#41031,#41032,#41033,#41034,
#41035,#41036,#41037,#41038,#41039,#41040,#41041,#41042,#41043,#41044,#41045,
#41046,#41047),.UNSPECIFIED.,.F.,.F.,(4,1,1,1,1,1,1,1,1,1,1,1,1,1,1,1,1,
1,1,1,1,1,1,1,1,1,1,1,1,1,1,1,1,1,1,1,1,1,1,1,1,1,1,1,1,1,1,1,1,1,1,1,1,
1,1,1,1,1,1,4),(10.3432104236078,10.5534239852748,11.0410733085876,11.5287226319004,
12.0163719552132,12.504021278526,12.9916706018388,13.4793199251516,13.9669692484644,
14.4546185717772,14.94226789509,15.4299172184027,15.9175665417155,16.4052158650283,
16.8928651883411,17.3805145116539,17.8681638349667,18.3558131582795,18.8434624815923,
19.3311118049051,19.8187611282179,20.3064104515307,20.7940597748435,21.2817090981563,
21.7693584214691,22.2570077447818,22.7446570680946,23.2323063914074,23.7199557147202,
24.207605038033,24.6952543613458,25.1829036846586,25.6705530079714,26.1582023312842,
26.645851654597,27.1335009779098,27.6211503012226,28.1087996245354,28.5964489478482,
29.0840982711609,29.5717475944737,30.0593969177865,30.5470462410993,31.0346955644121,
31.5223448877249,32.0099942110377,32.4976435343505,32.9852928576633,33.4729421809761,
33.9605915042889,34.4482408276017,34.9358901509145,35.4235394742273,35.91118879754,
36.3988381208528,36.8864874441656,37.3741367674784,37.8617860907912,38.349435414104,
38.8370847374168),.UNSPECIFIED.);
#676=B_SPLINE_CURVE_WITH_KNOTS('',3,(#41301,#41302,#41303,#41304,#41305,
#41306,#41307,#41308,#41309,#41310,#41311,#41312,#41313,#41314,#41315,#41316,
#41317,#41318,#41319,#41320,#41321,#41322,#41323,#41324,#41325,#41326,#41327,
#41328,#41329,#41330,#41331,#41332,#41333,#41334,#41335,#41336,#41337,#41338,
#41339,#41340,#41341,#41342,#41343,#41344,#41345,#41346,#41347,#41348,#41349),
 .UNSPECIFIED.,.F.,.F.,(4,3,3,3,3,3,3,3,3,3,3,3,3,3,3,3,4),(0.,0.0881387442926152,
0.180700997921297,0.22591832279636,0.243527785554388,0.27326325154998,0.36378372577003,
0.424829269926009,0.460795635173694,0.480982236187546,0.57372100351339,
0.579674857270561,0.658719602962808,0.681251247199192,0.774812612388552,
0.868884434159813,0.895853840039549),.UNSPECIFIED.);
#677=B_SPLINE_CURVE_WITH_KNOTS('',3,(#41350,#41351,#41352,#41353,#41354,
#41355,#41356,#41357,#41358,#41359,#41360,#41361,#41362,#41363,#41364,#41365,
#41366,#41367,#41368,#41369,#41370,#41371,#41372,#41373,#41374,#41375,#41376,
#41377,#41378,#41379,#41380,#41381,#41382,#41383,#41384,#41385,#41386,#41387,
#41388,#41389,#41390,#41391,#41392,#41393,#41394,#41395,#41396,#41397,#41398,
#41399,#41400,#41401,#41402,#41403,#41404,#41405,#41406,#41407,#41408,#41409,
#41410),.UNSPECIFIED.,.F.,.F.,(4,1,1,1,1,1,1,1,1,1,1,1,1,1,1,1,1,1,1,1,
1,1,1,1,1,1,1,1,1,1,1,1,1,1,1,1,1,1,1,1,1,1,1,1,1,1,1,1,1,1,1,1,1,1,1,1,
1,1,4),(11.8012855294006,11.8408078945879,12.3400070515813,12.8392062085746,
13.338405365568,13.8376045225613,14.3368036795547,14.8360028365481,15.3352019935414,
15.8344011505348,16.3336003075282,16.8327994645215,17.3319986215149,17.8311977785083,
18.3303969355016,18.829596092495,19.3287952494883,19.8279944064817,20.3271935634751,
20.8263927204684,21.3255918774618,21.8247910344552,22.3239901914485,22.8231893484419,
23.3223885054353,23.8215876624286,24.320786819422,24.8199859764153,25.3191851334087,
25.8183842904021,26.3175834473954,26.8167826043888,27.3159817613822,27.8151809183755,
28.3143800753689,28.8135792323623,29.3127783893556,29.811977546349,30.3111767033423,
30.8103758603357,31.3095750173291,31.8087741743224,32.3079733313158,32.8071724883092,
33.3063716453025,33.8055708022959,34.3047699592893,34.8039691162826,35.303168273276,
35.8023674302693,36.3015665872627,36.8007657442561,37.2999649012494,37.7991640582428,
38.2983632152362,38.7975623722295,39.2967615292229,39.7959606862163,40.2951598432096),
 .UNSPECIFIED.);
#678=B_SPLINE_CURVE_WITH_KNOTS('',3,(#41726,#41727,#41728,#41729,#41730,
#41731,#41732,#41733),.UNSPECIFIED.,.F.,.F.,(4,2,2,4),(0.,0.150083807667359,
0.232692116568135,0.322068030175859),.UNSPECIFIED.);
#1468=(
BOUNDED_CURVE()
B_SPLINE_CURVE(2,(#41740,#41741,#41742),.UNSPECIFIED.,.F.,.F.)
B_SPLINE_CURVE_WITH_KNOTS((3,3),(0.0820488586119731,0.652657405316371),
 .UNSPECIFIED.)
CURVE()
GEOMETRIC_REPRESENTATION_ITEM()
RATIONAL_B_SPLINE_CURVE((1.02442640079672,1.10366605866331,1.10366605866331))
REPRESENTATION_ITEM('')
);
#1469=(
BOUNDED_CURVE()
B_SPLINE_CURVE(2,(#41744,#41745,#41746),.UNSPECIFIED.,.F.,.F.)
B_SPLINE_CURVE_WITH_KNOTS((3,3),(0.0820488586119737,1.22326595202077),
 .UNSPECIFIED.)
CURVE()
GEOMETRIC_REPRESENTATION_ITEM()
RATIONAL_B_SPLINE_CURVE((1.02442640079672,1.18290571652989,1.02442640079672))
REPRESENTATION_ITEM('')
);
#1470=(
BOUNDED_CURVE()
B_SPLINE_CURVE(2,(#41748,#41749,#41750),.UNSPECIFIED.,.F.,.F.)
B_SPLINE_CURVE_WITH_KNOTS((3,3),(0.0820488586119732,1.22326595202077),
 .UNSPECIFIED.)
CURVE()
GEOMETRIC_REPRESENTATION_ITEM()
RATIONAL_B_SPLINE_CURVE((1.02442640079672,1.1829057165299,1.02442640079672))
REPRESENTATION_ITEM('')
);
#1471=(
BOUNDED_CURVE()
B_SPLINE_CURVE(2,(#41752,#41753,#41754),.UNSPECIFIED.,.F.,.F.)
B_SPLINE_CURVE_WITH_KNOTS((3,3),(0.082048858611974,1.22326595202077),
 .UNSPECIFIED.)
CURVE()
GEOMETRIC_REPRESENTATION_ITEM()
RATIONAL_B_SPLINE_CURVE((1.02442640079672,1.1829057165299,1.02442640079672))
REPRESENTATION_ITEM('')
);
#1472=(
BOUNDED_CURVE()
B_SPLINE_CURVE(2,(#41756,#41757,#41758),.UNSPECIFIED.,.F.,.F.)
B_SPLINE_CURVE_WITH_KNOTS((3,3),(0.0820488586119736,1.22326595202077),
 .UNSPECIFIED.)
CURVE()
GEOMETRIC_REPRESENTATION_ITEM()
RATIONAL_B_SPLINE_CURVE((1.02442640079672,1.1829057165299,1.02442640079672))
REPRESENTATION_ITEM('')
);
#1473=(
BOUNDED_CURVE()
B_SPLINE_CURVE(2,(#41760,#41761,#41762),.UNSPECIFIED.,.F.,.F.)
B_SPLINE_CURVE_WITH_KNOTS((3,3),(0.0820488586119736,1.22326595202077),
 .UNSPECIFIED.)
CURVE()
GEOMETRIC_REPRESENTATION_ITEM()
RATIONAL_B_SPLINE_CURVE((1.02442640079672,1.1829057165299,1.02442640079672))
REPRESENTATION_ITEM('')
);
#1474=(
BOUNDED_CURVE()
B_SPLINE_CURVE(2,(#41763,#41764,#41765),.UNSPECIFIED.,.F.,.F.)
B_SPLINE_CURVE_WITH_KNOTS((3,3),(0.652657405316371,1.22326595202077),
 .UNSPECIFIED.)
CURVE()
GEOMETRIC_REPRESENTATION_ITEM()
RATIONAL_B_SPLINE_CURVE((1.10366605866331,1.10366605866331,1.02442640079672))
REPRESENTATION_ITEM('')
);
#1475=(
BOUNDED_CURVE()
B_SPLINE_CURVE(2,(#41770,#41771,#41772),.UNSPECIFIED.,.F.,.F.)
B_SPLINE_CURVE_WITH_KNOTS((3,3),(0.0820488586119733,1.22326595202077),
 .UNSPECIFIED.)
CURVE()
GEOMETRIC_REPRESENTATION_ITEM()
RATIONAL_B_SPLINE_CURVE((1.02442640079672,1.1829057165299,1.02442640079672))
REPRESENTATION_ITEM('')
);
#1476=(
BOUNDED_CURVE()
B_SPLINE_CURVE(2,(#41777,#41778,#41779),.UNSPECIFIED.,.F.,.F.)
B_SPLINE_CURVE_WITH_KNOTS((3,3),(0.0820488586119739,1.22326595202077),
 .UNSPECIFIED.)
CURVE()
GEOMETRIC_REPRESENTATION_ITEM()
RATIONAL_B_SPLINE_CURVE((1.02442640079672,1.1829057165299,1.02442640079672))
REPRESENTATION_ITEM('')
);
#1477=(
BOUNDED_CURVE()
B_SPLINE_CURVE(2,(#41783,#41784,#41785),.UNSPECIFIED.,.F.,.F.)
B_SPLINE_CURVE_WITH_KNOTS((3,3),(0.0820488586119737,1.22326595202077),
 .UNSPECIFIED.)
CURVE()
GEOMETRIC_REPRESENTATION_ITEM()
RATIONAL_B_SPLINE_CURVE((1.02442640079672,1.1829057165299,1.02442640079672))
REPRESENTATION_ITEM('')
);
#1478=(
BOUNDED_CURVE()
B_SPLINE_CURVE(2,(#41788,#41789,#41790),.UNSPECIFIED.,.F.,.F.)
B_SPLINE_CURVE_WITH_KNOTS((3,3),(0.0820488586119733,1.22326595202077),
 .UNSPECIFIED.)
CURVE()
GEOMETRIC_REPRESENTATION_ITEM()
RATIONAL_B_SPLINE_CURVE((1.02442640079672,1.1829057165299,1.02442640079672))
REPRESENTATION_ITEM('')
);
#1479=(
BOUNDED_CURVE()
B_SPLINE_CURVE(2,(#41792,#41793,#41794),.UNSPECIFIED.,.F.,.F.)
B_SPLINE_CURVE_WITH_KNOTS((3,3),(0.652657405316372,1.22326595202077),
 .UNSPECIFIED.)
CURVE()
GEOMETRIC_REPRESENTATION_ITEM()
RATIONAL_B_SPLINE_CURVE((1.10366605866331,1.10366605866331,1.02442640079672))
REPRESENTATION_ITEM('')
);
#1480=(
BOUNDED_CURVE()
B_SPLINE_CURVE(2,(#41799,#41800,#41801),.UNSPECIFIED.,.F.,.F.)
B_SPLINE_CURVE_WITH_KNOTS((3,3),(0.0820488586119738,0.652657405316372),
 .UNSPECIFIED.)
CURVE()
GEOMETRIC_REPRESENTATION_ITEM()
RATIONAL_B_SPLINE_CURVE((1.02442640079672,1.10366605866331,1.10366605866331))
REPRESENTATION_ITEM('')
);
#1481=(
BOUNDED_CURVE()
B_SPLINE_CURVE(2,(#41802,#41803,#41804),.UNSPECIFIED.,.F.,.F.)
B_SPLINE_CURVE_WITH_KNOTS((3,3),(0.0820488586119739,1.22326595202077),
 .UNSPECIFIED.)
CURVE()
GEOMETRIC_REPRESENTATION_ITEM()
RATIONAL_B_SPLINE_CURVE((1.02442640079672,1.1829057165299,1.02442640079672))
REPRESENTATION_ITEM('')
);
#1515=SHAPE_REPRESENTATION_RELATIONSHIP('SRR','None',#59304,#1535);
#1535=ADVANCED_BREP_SHAPE_REPRESENTATION('',(#1582),#59191);
#1555=STYLED_ITEM('',(#59572),#1582);
#1582=MANIFOLD_SOLID_BREP('Stud body',#22811);
#1634=FACE_BOUND('',#4300,.T.);
#1635=FACE_BOUND('',#4303,.T.);
#1636=FACE_BOUND('',#4310,.T.);
#1637=FACE_BOUND('',#4313,.T.);
#1638=FACE_BOUND('',#4317,.T.);
#1975=PLANE('',#23515);
#1976=PLANE('',#23522);
#1977=PLANE('',#23529);
#1978=PLANE('',#23530);
#1979=PLANE('',#23531);
#1980=PLANE('',#23534);
#1981=PLANE('',#23535);
#1982=PLANE('',#23536);
#1983=PLANE('',#23538);
#1984=PLANE('',#23540);
#1985=PLANE('',#23542);
#1986=PLANE('',#23543);
#1987=PLANE('',#23548);
#1988=PLANE('',#23551);
#1989=PLANE('',#23556);
#2446=CYLINDRICAL_SURFACE('',#23492,0.57225);
#2447=CYLINDRICAL_SURFACE('',#23494,0.57225);
#2448=CYLINDRICAL_SURFACE('',#23495,0.57225);
#2449=CYLINDRICAL_SURFACE('',#23496,0.57225);
#2450=CYLINDRICAL_SURFACE('',#23497,0.57225);
#2451=CYLINDRICAL_SURFACE('',#23499,0.6925);
#2452=CYLINDRICAL_SURFACE('',#23501,0.6925);
#2453=CYLINDRICAL_SURFACE('',#23502,0.6925);
#2454=CYLINDRICAL_SURFACE('',#23503,0.6925);
#2455=CYLINDRICAL_SURFACE('',#23504,0.6925);
#2456=CYLINDRICAL_SURFACE('',#23505,0.6925);
#2457=CYLINDRICAL_SURFACE('',#23506,0.6925);
#2458=CYLINDRICAL_SURFACE('',#23507,0.60685);
#2459=CYLINDRICAL_SURFACE('',#23509,0.60685);
#2460=CYLINDRICAL_SURFACE('',#23510,0.60685);
#2461=CYLINDRICAL_SURFACE('',#23511,0.60685);
#2462=CYLINDRICAL_SURFACE('',#23512,0.60685);
#2463=CYLINDRICAL_SURFACE('',#23513,0.60685);
#2464=CYLINDRICAL_SURFACE('',#23514,0.60685);
#2465=CYLINDRICAL_SURFACE('',#23518,0.60685);
#2466=CYLINDRICAL_SURFACE('',#23520,0.6925);
#2467=CYLINDRICAL_SURFACE('',#23526,0.57225);
#2468=CYLINDRICAL_SURFACE('',#23544,0.3);
#2469=CYLINDRICAL_SURFACE('',#23546,0.3);
#2470=CYLINDRICAL_SURFACE('',#23553,0.56785);
#2921=FACE_OUTER_BOUND('',#4261,.T.);
#2922=FACE_OUTER_BOUND('',#4262,.T.);
#2923=FACE_OUTER_BOUND('',#4263,.T.);
#2924=FACE_OUTER_BOUND('',#4264,.T.);
#2925=FACE_OUTER_BOUND('',#4265,.T.);
#2926=FACE_OUTER_BOUND('',#4266,.T.);
#2927=FACE_OUTER_BOUND('',#4267,.T.);
#2928=FACE_OUTER_BOUND('',#4268,.T.);
#2929=FACE_OUTER_BOUND('',#4269,.T.);
#2930=FACE_OUTER_BOUND('',#4270,.T.);
#2931=FACE_OUTER_BOUND('',#4271,.T.);
#2932=FACE_OUTER_BOUND('',#4272,.T.);
#2933=FACE_OUTER_BOUND('',#4273,.T.);
#2934=FACE_OUTER_BOUND('',#4274,.T.);
#2935=FACE_OUTER_BOUND('',#4275,.T.);
#2936=FACE_OUTER_BOUND('',#4276,.T.);
#2937=FACE_OUTER_BOUND('',#4277,.T.);
#2938=FACE_OUTER_BOUND('',#4278,.T.);
#2939=FACE_OUTER_BOUND('',#4279,.T.);
#2940=FACE_OUTER_BOUND('',#4280,.T.);
#2941=FACE_OUTER_BOUND('',#4281,.T.);
#2942=FACE_OUTER_BOUND('',#4282,.T.);
#2943=FACE_OUTER_BOUND('',#4283,.T.);
#2944=FACE_OUTER_BOUND('',#4284,.T.);
#2945=FACE_OUTER_BOUND('',#4285,.T.);
#2946=FACE_OUTER_BOUND('',#4286,.T.);
#2947=FACE_OUTER_BOUND('',#4287,.T.);
#2948=FACE_OUTER_BOUND('',#4288,.T.);
#2949=FACE_OUTER_BOUND('',#4289,.T.);
#2950=FACE_OUTER_BOUND('',#4290,.T.);
#2951=FACE_OUTER_BOUND('',#4291,.T.);
#2952=FACE_OUTER_BOUND('',#4292,.T.);
#2953=FACE_OUTER_BOUND('',#4293,.T.);
#2954=FACE_OUTER_BOUND('',#4294,.T.);
#2955=FACE_OUTER_BOUND('',#4295,.T.);
#2956=FACE_OUTER_BOUND('',#4296,.T.);
#2957=FACE_OUTER_BOUND('',#4297,.T.);
#2958=FACE_OUTER_BOUND('',#4298,.T.);
#2959=FACE_OUTER_BOUND('',#4299,.T.);
#2960=FACE_OUTER_BOUND('',#4301,.T.);
#2961=FACE_OUTER_BOUND('',#4302,.T.);
#2962=FACE_OUTER_BOUND('',#4304,.T.);
#2963=FACE_OUTER_BOUND('',#4305,.T.);
#2964=FACE_OUTER_BOUND('',#4306,.T.);
#2965=FACE_OUTER_BOUND('',#4307,.T.);
#2966=FACE_OUTER_BOUND('',#4308,.T.);
#2967=FACE_OUTER_BOUND('',#4309,.T.);
#2968=FACE_OUTER_BOUND('',#4311,.T.);
#2969=FACE_OUTER_BOUND('',#4312,.T.);
#2970=FACE_OUTER_BOUND('',#4314,.T.);
#2971=FACE_OUTER_BOUND('',#4315,.T.);
#2972=FACE_OUTER_BOUND('',#4316,.T.);
#2973=FACE_OUTER_BOUND('',#4318,.T.);
#4261=EDGE_LOOP('',(#15846,#15847,#15848,#15849));
#4262=EDGE_LOOP('',(#15850,#15851,#15852,#15853));
#4263=EDGE_LOOP('',(#15854,#15855,#15856,#15857));
#4264=EDGE_LOOP('',(#15858,#15859,#15860,#15861));
#4265=EDGE_LOOP('',(#15862,#15863,#15864,#15865,#15866));
#4266=EDGE_LOOP('',(#15867,#15868,#15869,#15870));
#4267=EDGE_LOOP('',(#15871,#15872,#15873,#15874));
#4268=EDGE_LOOP('',(#15875,#15876,#15877,#15878));
#4269=EDGE_LOOP('',(#15879,#15880,#15881,#15882));
#4270=EDGE_LOOP('',(#15883,#15884,#15885,#15886));
#4271=EDGE_LOOP('',(#15887,#15888,#15889,#15890));
#4272=EDGE_LOOP('',(#15891,#15892,#15893,#15894));
#4273=EDGE_LOOP('',(#15895,#15896,#15897,#15898));
#4274=EDGE_LOOP('',(#15899,#15900,#15901,#15902));
#4275=EDGE_LOOP('',(#15903,#15904,#15905,#15906));
#4276=EDGE_LOOP('',(#15907,#15908,#15909,#15910));
#4277=EDGE_LOOP('',(#15911,#15912,#15913,#15914));
#4278=EDGE_LOOP('',(#15915,#15916,#15917,#15918));
#4279=EDGE_LOOP('',(#15919,#15920,#15921,#15922));
#4280=EDGE_LOOP('',(#15923,#15924,#15925,#15926,#15927));
#4281=EDGE_LOOP('',(#15928,#15929,#15930,#15931,#15932,#15933,#15934,#15935,
#15936,#15937,#15938,#15939,#15940,#15941,#15942,#15943,#15944,#15945));
#4282=EDGE_LOOP('',(#15946,#15947,#15948,#15949));
#4283=EDGE_LOOP('',(#15950,#15951,#15952,#15953,#15954,#15955,#15956,#15957,
#15958,#15959,#15960,#15961,#15962,#15963,#15964,#15965,#15966,#15967));
#4284=EDGE_LOOP('',(#15968,#15969,#15970,#15971));
#4285=EDGE_LOOP('',(#15972,#15973,#15974,#15975));
#4286=EDGE_LOOP('',(#15976,#15977,#15978,#15979));
#4287=EDGE_LOOP('',(#15980,#15981,#15982,#15983,#15984,#15985,#15986,#15987,
#15988));
#4288=EDGE_LOOP('',(#15989,#15990,#15991,#15992,#15993,#15994,#15995,#15996,
#15997,#15998));
#4289=EDGE_LOOP('',(#15999,#16000,#16001));
#4290=EDGE_LOOP('',(#16002,#16003,#16004,#16005,#16006,#16007,#16008,#16009));
#4291=EDGE_LOOP('',(#16010,#16011,#16012,#16013));
#4292=EDGE_LOOP('',(#16014,#16015,#16016,#16017));
#4293=EDGE_LOOP('',(#16018,#16019,#16020,#16021,#16022,#16023,#16024,#16025,
#16026,#16027));
#4294=EDGE_LOOP('',(#16028,#16029,#16030,#16031));
#4295=EDGE_LOOP('',(#16032,#16033,#16034,#16035));
#4296=EDGE_LOOP('',(#16036,#16037,#16038,#16039));
#4297=EDGE_LOOP('',(#16040,#16041,#16042,#16043,#16044,#16045,#16046,#16047,
#16048,#16049));
#4298=EDGE_LOOP('',(#16050,#16051,#16052,#16053));
#4299=EDGE_LOOP('',(#16054));
#4300=EDGE_LOOP('',(#16055,#16056,#16057,#16058));
#4301=EDGE_LOOP('',(#16059));
#4302=EDGE_LOOP('',(#16060));
#4303=EDGE_LOOP('',(#16061));
#4304=EDGE_LOOP('',(#16062));
#4305=EDGE_LOOP('',(#16063,#16064,#16065,#16066));
#4306=EDGE_LOOP('',(#16067,#16068,#16069,#16070,#16071,#16072));
#4307=EDGE_LOOP('',(#16073,#16074,#16075,#16076));
#4308=EDGE_LOOP('',(#16077,#16078,#16079,#16080));
#4309=EDGE_LOOP('',(#16081));
#4310=EDGE_LOOP('',(#16082));
#4311=EDGE_LOOP('',(#16083,#16084,#16085,#16086,#16087));
#4312=EDGE_LOOP('',(#16088,#16089,#16090,#16091,#16092,#16093,#16094));
#4313=EDGE_LOOP('',(#16095));
#4314=EDGE_LOOP('',(#16096,#16097,#16098,#16099));
#4315=EDGE_LOOP('',(#16100,#16101,#16102,#16103,#16104,#16105));
#4316=EDGE_LOOP('',(#16106));
#4317=EDGE_LOOP('',(#16107));
#4318=EDGE_LOOP('',(#16108,#16109,#16110,#16111));
#5824=LINE('',#37144,#7257);
#5825=LINE('',#37172,#7258);
#5826=LINE('',#37210,#7259);
#5827=LINE('',#37248,#7260);
#5828=LINE('',#37286,#7261);
#5829=LINE('',#37325,#7262);
#5830=LINE('',#37358,#7263);
#5831=LINE('',#37442,#7264);
#5832=LINE('',#37532,#7265);
#5833=LINE('',#37616,#7266);
#5834=LINE('',#37706,#7267);
#5835=LINE('',#37796,#7268);
#5836=LINE('',#37880,#7269);
#5837=LINE('',#37900,#7270);
#5838=LINE('',#37937,#7271);
#5839=LINE('',#37974,#7272);
#5840=LINE('',#38012,#7273);
#5841=LINE('',#38049,#7274);
#5842=LINE('',#38086,#7275);
#5843=LINE('',#41738,#7276);
#5844=LINE('',#41768,#7277);
#5845=LINE('',#41773,#7278);
#5846=LINE('',#41776,#7279);
#5847=LINE('',#41782,#7280);
#5848=LINE('',#41796,#7281);
#5849=LINE('',#41806,#7282);
#5850=LINE('',#41818,#7283);
#5851=LINE('',#41822,#7284);
#5852=LINE('',#41827,#7285);
#5853=LINE('',#41832,#7286);
#5854=LINE('',#41837,#7287);
#5855=LINE('',#41841,#7288);
#5856=LINE('',#41846,#7289);
#7257=VECTOR('',#26346,0.57225);
#7258=VECTOR('',#26351,0.57225);
#7259=VECTOR('',#26354,0.57225);
#7260=VECTOR('',#26357,0.57225);
#7261=VECTOR('',#26360,0.57225);
#7262=VECTOR('',#26365,0.7);
#7263=VECTOR('',#26370,0.7);
#7264=VECTOR('',#26373,0.7);
#7265=VECTOR('',#26376,0.7);
#7266=VECTOR('',#26379,0.7);
#7267=VECTOR('',#26382,0.7);
#7268=VECTOR('',#26385,0.7);
#7269=VECTOR('',#26388,0.60685);
#7270=VECTOR('',#26393,0.60685);
#7271=VECTOR('',#26396,0.60685);
#7272=VECTOR('',#26399,0.60685);
#7273=VECTOR('',#26402,0.60685);
#7274=VECTOR('',#26405,0.60685);
#7275=VECTOR('',#26408,0.60685);
#7276=VECTOR('',#26437,1.02473275573014);
#7277=VECTOR('',#26440,1.);
#7278=VECTOR('',#26441,1.);
#7279=VECTOR('',#26444,1.);
#7280=VECTOR('',#26447,1.);
#7281=VECTOR('',#26450,1.02473275573014);
#7282=VECTOR('',#26455,1.);
#7283=VECTOR('',#26472,1.);
#7284=VECTOR('',#26477,0.3);
#7285=VECTOR('',#26484,0.3);
#7286=VECTOR('',#26491,0.61785);
#7287=VECTOR('',#26498,0.56785);
#7288=VECTOR('',#26503,0.67);
#7289=VECTOR('',#26510,0.39);
#8552=CIRCLE('',#23493,0.57225);
#8553=CIRCLE('',#23498,0.57225);
#8554=CIRCLE('',#23500,0.6925);
#8555=CIRCLE('',#23508,0.60685);
#8556=CIRCLE('',#23516,0.6925);
#8557=CIRCLE('',#23517,0.6925);
#8558=CIRCLE('',#23519,0.60685);
#8559=CIRCLE('',#23521,0.6925);
#8560=CIRCLE('',#23523,0.6516);
#8561=CIRCLE('',#23524,0.6516);
#8562=CIRCLE('',#23525,0.57225);
#8563=CIRCLE('',#23528,0.9025);
#8564=CIRCLE('',#23533,0.9025);
#8565=CIRCLE('',#23537,0.3);
#8566=CIRCLE('',#23539,0.56785);
#8567=CIRCLE('',#23541,0.3);
#8568=CIRCLE('',#23545,0.3);
#8569=CIRCLE('',#23547,0.3);
#8570=CIRCLE('',#23549,0.57785);
#8571=CIRCLE('',#23552,0.56785);
#8572=CIRCLE('',#23555,0.64);
#8573=CIRCLE('',#23557,0.48);
#9555=VERTEX_POINT('',#37142);
#9556=VERTEX_POINT('',#37143);
#9557=VERTEX_POINT('',#37145);
#9558=VERTEX_POINT('',#37157);
#9559=VERTEX_POINT('',#37170);
#9560=VERTEX_POINT('',#37171);
#9561=VERTEX_POINT('',#37208);
#9562=VERTEX_POINT('',#37209);
#9563=VERTEX_POINT('',#37246);
#9564=VERTEX_POINT('',#37247);
#9565=VERTEX_POINT('',#37284);
#9566=VERTEX_POINT('',#37285);
#9567=VERTEX_POINT('',#37287);
#9568=VERTEX_POINT('',#37323);
#9569=VERTEX_POINT('',#37324);
#9570=VERTEX_POINT('',#37326);
#9571=VERTEX_POINT('',#37343);
#9572=VERTEX_POINT('',#37356);
#9573=VERTEX_POINT('',#37357);
#9574=VERTEX_POINT('',#37440);
#9575=VERTEX_POINT('',#37441);
#9576=VERTEX_POINT('',#37530);
#9577=VERTEX_POINT('',#37531);
#9578=VERTEX_POINT('',#37614);
#9579=VERTEX_POINT('',#37615);
#9580=VERTEX_POINT('',#37704);
#9581=VERTEX_POINT('',#37705);
#9582=VERTEX_POINT('',#37794);
#9583=VERTEX_POINT('',#37795);
#9584=VERTEX_POINT('',#37878);
#9585=VERTEX_POINT('',#37879);
#9586=VERTEX_POINT('',#37881);
#9587=VERTEX_POINT('',#37890);
#9588=VERTEX_POINT('',#37898);
#9589=VERTEX_POINT('',#37899);
#9590=VERTEX_POINT('',#37935);
#9591=VERTEX_POINT('',#37936);
#9592=VERTEX_POINT('',#37972);
#9593=VERTEX_POINT('',#37973);
#9594=VERTEX_POINT('',#38010);
#9595=VERTEX_POINT('',#38011);
#9596=VERTEX_POINT('',#38047);
#9597=VERTEX_POINT('',#38048);
#9598=VERTEX_POINT('',#38084);
#9599=VERTEX_POINT('',#38085);
#9600=VERTEX_POINT('',#38121);
#9601=VERTEX_POINT('',#38195);
#9602=VERTEX_POINT('',#38197);
#9603=VERTEX_POINT('',#38686);
#9604=VERTEX_POINT('',#38775);
#9605=VERTEX_POINT('',#39587);
#9606=VERTEX_POINT('',#39588);
#9607=VERTEX_POINT('',#39597);
#9608=VERTEX_POINT('',#39776);
#9609=VERTEX_POINT('',#40099);
#9610=VERTEX_POINT('',#40146);
#9611=VERTEX_POINT('',#40580);
#9612=VERTEX_POINT('',#40594);
#9613=VERTEX_POINT('',#40597);
#9614=VERTEX_POINT('',#40606);
#9615=VERTEX_POINT('',#40979);
#9616=VERTEX_POINT('',#41300);
#9617=VERTEX_POINT('',#41735);
#9618=VERTEX_POINT('',#41737);
#9619=VERTEX_POINT('',#41739);
#9620=VERTEX_POINT('',#41743);
#9621=VERTEX_POINT('',#41747);
#9622=VERTEX_POINT('',#41751);
#9623=VERTEX_POINT('',#41755);
#9624=VERTEX_POINT('',#41759);
#9625=VERTEX_POINT('',#41767);
#9626=VERTEX_POINT('',#41769);
#9627=VERTEX_POINT('',#41775);
#9628=VERTEX_POINT('',#41781);
#9629=VERTEX_POINT('',#41787);
#9630=VERTEX_POINT('',#41791);
#9631=VERTEX_POINT('',#41795);
#9632=VERTEX_POINT('',#41798);
#9633=VERTEX_POINT('',#41809);
#9634=VERTEX_POINT('',#41812);
#9635=VERTEX_POINT('',#41815);
#9636=VERTEX_POINT('',#41821);
#9637=VERTEX_POINT('',#41825);
#9638=VERTEX_POINT('',#41829);
#9639=VERTEX_POINT('',#41834);
#9640=VERTEX_POINT('',#41839);
#9641=VERTEX_POINT('',#41843);
#11927=EDGE_CURVE('',#9555,#9556,#5824,.T.);
#11928=EDGE_CURVE('',#9555,#9557,#615,.T.);
#11929=EDGE_CURVE('',#9558,#9557,#8552,.T.);
#11930=EDGE_CURVE('',#9556,#9558,#616,.T.);
#11931=EDGE_CURVE('',#9559,#9560,#5825,.T.);
#11932=EDGE_CURVE('',#9559,#9555,#617,.T.);
#11933=EDGE_CURVE('',#9560,#9556,#618,.T.);
#11934=EDGE_CURVE('',#9561,#9562,#5826,.T.);
#11935=EDGE_CURVE('',#9561,#9559,#619,.T.);
#11936=EDGE_CURVE('',#9562,#9560,#620,.T.);
#11937=EDGE_CURVE('',#9563,#9564,#5827,.T.);
#11938=EDGE_CURVE('',#9563,#9561,#621,.T.);
#11939=EDGE_CURVE('',#9564,#9562,#622,.T.);
#11940=EDGE_CURVE('',#9565,#9566,#5828,.T.);
#11941=EDGE_CURVE('',#9567,#9565,#8553,.T.);
#11942=EDGE_CURVE('',#9567,#9563,#623,.T.);
#11943=EDGE_CURVE('',#9566,#9564,#624,.T.);
#11944=EDGE_CURVE('',#9568,#9569,#5829,.T.);
#11945=EDGE_CURVE('',#9568,#9570,#625,.T.);
#11946=EDGE_CURVE('',#9570,#9571,#8554,.F.);
#11947=EDGE_CURVE('',#9571,#9569,#626,.T.);
#11948=EDGE_CURVE('',#9572,#9573,#5830,.T.);
#11949=EDGE_CURVE('',#9572,#9568,#627,.T.);
#11950=EDGE_CURVE('',#9569,#9573,#628,.T.);
#11951=EDGE_CURVE('',#9574,#9575,#5831,.T.);
#11952=EDGE_CURVE('',#9574,#9572,#629,.T.);
#11953=EDGE_CURVE('',#9573,#9575,#630,.T.);
#11954=EDGE_CURVE('',#9576,#9577,#5832,.T.);
#11955=EDGE_CURVE('',#9576,#9574,#631,.T.);
#11956=EDGE_CURVE('',#9575,#9577,#632,.T.);
#11957=EDGE_CURVE('',#9578,#9579,#5833,.T.);
#11958=EDGE_CURVE('',#9578,#9576,#633,.T.);
#11959=EDGE_CURVE('',#9577,#9579,#634,.T.);
#11960=EDGE_CURVE('',#9580,#9581,#5834,.T.);
#11961=EDGE_CURVE('',#9580,#9578,#635,.T.);
#11962=EDGE_CURVE('',#9579,#9581,#636,.T.);
#11963=EDGE_CURVE('',#9582,#9583,#5835,.T.);
#11964=EDGE_CURVE('',#9582,#9580,#637,.T.);
#11965=EDGE_CURVE('',#9581,#9583,#638,.T.);
#11966=EDGE_CURVE('',#9584,#9585,#5836,.T.);
#11967=EDGE_CURVE('',#9584,#9586,#639,.T.);
#11968=EDGE_CURVE('',#9587,#9586,#8555,.T.);
#11969=EDGE_CURVE('',#9585,#9587,#640,.T.);
#11970=EDGE_CURVE('',#9588,#9589,#5837,.T.);
#11971=EDGE_CURVE('',#9588,#9584,#641,.T.);
#11972=EDGE_CURVE('',#9589,#9585,#642,.T.);
#11973=EDGE_CURVE('',#9590,#9591,#5838,.T.);
#11974=EDGE_CURVE('',#9590,#9588,#643,.T.);
#11975=EDGE_CURVE('',#9591,#9589,#644,.T.);
#11976=EDGE_CURVE('',#9592,#9593,#5839,.T.);
#11977=EDGE_CURVE('',#9592,#9590,#645,.T.);
#11978=EDGE_CURVE('',#9593,#9591,#646,.T.);
#11979=EDGE_CURVE('',#9594,#9595,#5840,.T.);
#11980=EDGE_CURVE('',#9594,#9592,#647,.T.);
#11981=EDGE_CURVE('',#9595,#9593,#648,.T.);
#11982=EDGE_CURVE('',#9596,#9597,#5841,.T.);
#11983=EDGE_CURVE('',#9596,#9594,#649,.T.);
#11984=EDGE_CURVE('',#9597,#9595,#650,.T.);
#11985=EDGE_CURVE('',#9598,#9599,#5842,.T.);
#11986=EDGE_CURVE('',#9598,#9596,#651,.T.);
#11987=EDGE_CURVE('',#9599,#9597,#652,.T.);
#11988=EDGE_CURVE('',#9586,#9600,#653,.T.);
#11989=EDGE_CURVE('',#9601,#9600,#8556,.F.);
#11990=EDGE_CURVE('',#9602,#9601,#8557,.F.);
#11991=EDGE_CURVE('',#9602,#9587,#654,.T.);
#11992=EDGE_CURVE('',#9583,#9602,#655,.T.);
#11993=EDGE_CURVE('',#9603,#9571,#656,.T.);
#11994=EDGE_CURVE('',#9603,#9599,#657,.T.);
#11995=EDGE_CURVE('',#9604,#9603,#8558,.T.);
#11996=EDGE_CURVE('',#9604,#9598,#658,.T.);
#11997=EDGE_CURVE('',#9570,#9604,#659,.T.);
#11998=EDGE_CURVE('',#9600,#9582,#660,.T.);
#11999=EDGE_CURVE('',#9600,#9602,#8559,.F.);
#12000=EDGE_CURVE('',#9605,#9606,#661,.T.);
#12001=EDGE_CURVE('',#9607,#9605,#662,.T.);
#12002=EDGE_CURVE('',#9608,#9607,#663,.T.);
#12003=EDGE_CURVE('',#9608,#9606,#664,.T.);
#12004=EDGE_CURVE('',#9606,#9609,#665,.T.);
#12005=EDGE_CURVE('',#9610,#9608,#666,.T.);
#12006=EDGE_CURVE('',#9610,#9609,#667,.T.);
#12007=EDGE_CURVE('',#9609,#9558,#668,.T.);
#12008=EDGE_CURVE('',#9611,#9610,#669,.T.);
#12009=EDGE_CURVE('',#9611,#9566,#670,.T.);
#12010=EDGE_CURVE('',#9607,#9612,#8560,.T.);
#12011=EDGE_CURVE('',#9612,#9607,#8561,.T.);
#12012=EDGE_CURVE('',#9607,#9613,#671,.T.);
#12013=EDGE_CURVE('',#9613,#9614,#672,.T.);
#12014=EDGE_CURVE('',#9614,#9567,#673,.T.);
#12015=EDGE_CURVE('',#9565,#9611,#8562,.T.);
#12016=EDGE_CURVE('',#9557,#9615,#674,.T.);
#12017=EDGE_CURVE('',#9614,#9615,#675,.T.);
#12018=EDGE_CURVE('',#9615,#9616,#676,.T.);
#12019=EDGE_CURVE('',#9613,#9616,#677,.T.);
#12020=EDGE_CURVE('',#9616,#9605,#678,.T.);
#12021=EDGE_CURVE('',#9617,#9617,#8563,.T.);
#12022=EDGE_CURVE('',#9617,#9618,#5843,.T.);
#12023=EDGE_CURVE('',#9619,#9618,#1468,.T.);
#12024=EDGE_CURVE('',#9620,#9619,#1469,.T.);
#12025=EDGE_CURVE('',#9621,#9620,#1470,.T.);
#12026=EDGE_CURVE('',#9622,#9621,#1471,.T.);
#12027=EDGE_CURVE('',#9623,#9622,#1472,.T.);
#12028=EDGE_CURVE('',#9624,#9623,#1473,.T.);
#12029=EDGE_CURVE('',#9618,#9624,#1474,.T.);
#12030=EDGE_CURVE('',#9622,#9625,#5844,.T.);
#12031=EDGE_CURVE('',#9625,#9626,#1475,.T.);
#12032=EDGE_CURVE('',#9623,#9626,#5845,.T.);
#12033=EDGE_CURVE('',#9621,#9627,#5846,.T.);
#12034=EDGE_CURVE('',#9627,#9625,#1476,.T.);
#12035=EDGE_CURVE('',#9620,#9628,#5847,.T.);
#12036=EDGE_CURVE('',#9628,#9627,#1477,.T.);
#12037=EDGE_CURVE('',#9629,#9628,#1478,.T.);
#12038=EDGE_CURVE('',#9630,#9629,#1479,.T.);
#12039=EDGE_CURVE('',#9630,#9631,#5848,.T.);
#12040=EDGE_CURVE('',#9631,#9631,#8564,.T.);
#12041=EDGE_CURVE('',#9632,#9630,#1480,.T.);
#12042=EDGE_CURVE('',#9626,#9632,#1481,.T.);
#12043=EDGE_CURVE('',#9619,#9629,#5849,.T.);
#12044=EDGE_CURVE('',#9633,#9633,#8565,.T.);
#12045=EDGE_CURVE('',#9634,#9634,#8566,.T.);
#12046=EDGE_CURVE('',#9635,#9635,#8567,.T.);
#12047=EDGE_CURVE('',#9624,#9632,#5850,.T.);
#12048=EDGE_CURVE('',#9635,#9636,#5851,.T.);
#12049=EDGE_CURVE('',#9636,#9636,#8568,.T.);
#12050=EDGE_CURVE('',#9637,#9637,#8569,.T.);
#12051=EDGE_CURVE('',#9637,#9633,#5852,.T.);
#12052=EDGE_CURVE('',#9638,#9638,#8570,.T.);
#12053=EDGE_CURVE('',#9612,#9638,#5853,.T.);
#12054=EDGE_CURVE('',#9639,#9639,#8571,.T.);
#12055=EDGE_CURVE('',#9634,#9639,#5854,.T.);
#12056=EDGE_CURVE('',#9640,#9640,#8572,.T.);
#12057=EDGE_CURVE('',#9640,#9601,#5855,.T.);
#12058=EDGE_CURVE('',#9641,#9641,#8573,.T.);
#12059=EDGE_CURVE('',#9641,#9637,#5856,.T.);
#15846=ORIENTED_EDGE('',*,*,#11927,.F.);
#15847=ORIENTED_EDGE('',*,*,#11928,.T.);
#15848=ORIENTED_EDGE('',*,*,#11929,.F.);
#15849=ORIENTED_EDGE('',*,*,#11930,.F.);
#15850=ORIENTED_EDGE('',*,*,#11931,.F.);
#15851=ORIENTED_EDGE('',*,*,#11932,.T.);
#15852=ORIENTED_EDGE('',*,*,#11927,.T.);
#15853=ORIENTED_EDGE('',*,*,#11933,.F.);
#15854=ORIENTED_EDGE('',*,*,#11934,.F.);
#15855=ORIENTED_EDGE('',*,*,#11935,.T.);
#15856=ORIENTED_EDGE('',*,*,#11931,.T.);
#15857=ORIENTED_EDGE('',*,*,#11936,.F.);
#15858=ORIENTED_EDGE('',*,*,#11937,.F.);
#15859=ORIENTED_EDGE('',*,*,#11938,.T.);
#15860=ORIENTED_EDGE('',*,*,#11934,.T.);
#15861=ORIENTED_EDGE('',*,*,#11939,.F.);
#15862=ORIENTED_EDGE('',*,*,#11940,.F.);
#15863=ORIENTED_EDGE('',*,*,#11941,.F.);
#15864=ORIENTED_EDGE('',*,*,#11942,.T.);
#15865=ORIENTED_EDGE('',*,*,#11937,.T.);
#15866=ORIENTED_EDGE('',*,*,#11943,.F.);
#15867=ORIENTED_EDGE('',*,*,#11944,.F.);
#15868=ORIENTED_EDGE('',*,*,#11945,.T.);
#15869=ORIENTED_EDGE('',*,*,#11946,.T.);
#15870=ORIENTED_EDGE('',*,*,#11947,.T.);
#15871=ORIENTED_EDGE('',*,*,#11948,.F.);
#15872=ORIENTED_EDGE('',*,*,#11949,.T.);
#15873=ORIENTED_EDGE('',*,*,#11944,.T.);
#15874=ORIENTED_EDGE('',*,*,#11950,.T.);
#15875=ORIENTED_EDGE('',*,*,#11951,.F.);
#15876=ORIENTED_EDGE('',*,*,#11952,.T.);
#15877=ORIENTED_EDGE('',*,*,#11948,.T.);
#15878=ORIENTED_EDGE('',*,*,#11953,.T.);
#15879=ORIENTED_EDGE('',*,*,#11954,.F.);
#15880=ORIENTED_EDGE('',*,*,#11955,.T.);
#15881=ORIENTED_EDGE('',*,*,#11951,.T.);
#15882=ORIENTED_EDGE('',*,*,#11956,.T.);
#15883=ORIENTED_EDGE('',*,*,#11957,.F.);
#15884=ORIENTED_EDGE('',*,*,#11958,.T.);
#15885=ORIENTED_EDGE('',*,*,#11954,.T.);
#15886=ORIENTED_EDGE('',*,*,#11959,.T.);
#15887=ORIENTED_EDGE('',*,*,#11960,.F.);
#15888=ORIENTED_EDGE('',*,*,#11961,.T.);
#15889=ORIENTED_EDGE('',*,*,#11957,.T.);
#15890=ORIENTED_EDGE('',*,*,#11962,.T.);
#15891=ORIENTED_EDGE('',*,*,#11963,.F.);
#15892=ORIENTED_EDGE('',*,*,#11964,.T.);
#15893=ORIENTED_EDGE('',*,*,#11960,.T.);
#15894=ORIENTED_EDGE('',*,*,#11965,.T.);
#15895=ORIENTED_EDGE('',*,*,#11966,.F.);
#15896=ORIENTED_EDGE('',*,*,#11967,.T.);
#15897=ORIENTED_EDGE('',*,*,#11968,.F.);
#15898=ORIENTED_EDGE('',*,*,#11969,.F.);
#15899=ORIENTED_EDGE('',*,*,#11970,.F.);
#15900=ORIENTED_EDGE('',*,*,#11971,.T.);
#15901=ORIENTED_EDGE('',*,*,#11966,.T.);
#15902=ORIENTED_EDGE('',*,*,#11972,.F.);
#15903=ORIENTED_EDGE('',*,*,#11973,.F.);
#15904=ORIENTED_EDGE('',*,*,#11974,.T.);
#15905=ORIENTED_EDGE('',*,*,#11970,.T.);
#15906=ORIENTED_EDGE('',*,*,#11975,.F.);
#15907=ORIENTED_EDGE('',*,*,#11976,.F.);
#15908=ORIENTED_EDGE('',*,*,#11977,.T.);
#15909=ORIENTED_EDGE('',*,*,#11973,.T.);
#15910=ORIENTED_EDGE('',*,*,#11978,.F.);
#15911=ORIENTED_EDGE('',*,*,#11979,.F.);
#15912=ORIENTED_EDGE('',*,*,#11980,.T.);
#15913=ORIENTED_EDGE('',*,*,#11976,.T.);
#15914=ORIENTED_EDGE('',*,*,#11981,.F.);
#15915=ORIENTED_EDGE('',*,*,#11982,.F.);
#15916=ORIENTED_EDGE('',*,*,#11983,.T.);
#15917=ORIENTED_EDGE('',*,*,#11979,.T.);
#15918=ORIENTED_EDGE('',*,*,#11984,.F.);
#15919=ORIENTED_EDGE('',*,*,#11985,.F.);
#15920=ORIENTED_EDGE('',*,*,#11986,.T.);
#15921=ORIENTED_EDGE('',*,*,#11982,.T.);
#15922=ORIENTED_EDGE('',*,*,#11987,.F.);
#15923=ORIENTED_EDGE('',*,*,#11968,.T.);
#15924=ORIENTED_EDGE('',*,*,#11988,.T.);
#15925=ORIENTED_EDGE('',*,*,#11989,.F.);
#15926=ORIENTED_EDGE('',*,*,#11990,.F.);
#15927=ORIENTED_EDGE('',*,*,#11991,.T.);
#15928=ORIENTED_EDGE('',*,*,#11991,.F.);
#15929=ORIENTED_EDGE('',*,*,#11992,.F.);
#15930=ORIENTED_EDGE('',*,*,#11965,.F.);
#15931=ORIENTED_EDGE('',*,*,#11962,.F.);
#15932=ORIENTED_EDGE('',*,*,#11959,.F.);
#15933=ORIENTED_EDGE('',*,*,#11956,.F.);
#15934=ORIENTED_EDGE('',*,*,#11953,.F.);
#15935=ORIENTED_EDGE('',*,*,#11950,.F.);
#15936=ORIENTED_EDGE('',*,*,#11947,.F.);
#15937=ORIENTED_EDGE('',*,*,#11993,.F.);
#15938=ORIENTED_EDGE('',*,*,#11994,.T.);
#15939=ORIENTED_EDGE('',*,*,#11987,.T.);
#15940=ORIENTED_EDGE('',*,*,#11984,.T.);
#15941=ORIENTED_EDGE('',*,*,#11981,.T.);
#15942=ORIENTED_EDGE('',*,*,#11978,.T.);
#15943=ORIENTED_EDGE('',*,*,#11975,.T.);
#15944=ORIENTED_EDGE('',*,*,#11972,.T.);
#15945=ORIENTED_EDGE('',*,*,#11969,.T.);
#15946=ORIENTED_EDGE('',*,*,#11985,.T.);
#15947=ORIENTED_EDGE('',*,*,#11994,.F.);
#15948=ORIENTED_EDGE('',*,*,#11995,.F.);
#15949=ORIENTED_EDGE('',*,*,#11996,.T.);
#15950=ORIENTED_EDGE('',*,*,#11988,.F.);
#15951=ORIENTED_EDGE('',*,*,#11967,.F.);
#15952=ORIENTED_EDGE('',*,*,#11971,.F.);
#15953=ORIENTED_EDGE('',*,*,#11974,.F.);
#15954=ORIENTED_EDGE('',*,*,#11977,.F.);
#15955=ORIENTED_EDGE('',*,*,#11980,.F.);
#15956=ORIENTED_EDGE('',*,*,#11983,.F.);
#15957=ORIENTED_EDGE('',*,*,#11986,.F.);
#15958=ORIENTED_EDGE('',*,*,#11996,.F.);
#15959=ORIENTED_EDGE('',*,*,#11997,.F.);
#15960=ORIENTED_EDGE('',*,*,#11945,.F.);
#15961=ORIENTED_EDGE('',*,*,#11949,.F.);
#15962=ORIENTED_EDGE('',*,*,#11952,.F.);
#15963=ORIENTED_EDGE('',*,*,#11955,.F.);
#15964=ORIENTED_EDGE('',*,*,#11958,.F.);
#15965=ORIENTED_EDGE('',*,*,#11961,.F.);
#15966=ORIENTED_EDGE('',*,*,#11964,.F.);
#15967=ORIENTED_EDGE('',*,*,#11998,.F.);
#15968=ORIENTED_EDGE('',*,*,#11963,.T.);
#15969=ORIENTED_EDGE('',*,*,#11992,.T.);
#15970=ORIENTED_EDGE('',*,*,#11999,.F.);
#15971=ORIENTED_EDGE('',*,*,#11998,.T.);
#15972=ORIENTED_EDGE('',*,*,#12000,.F.);
#15973=ORIENTED_EDGE('',*,*,#12001,.F.);
#15974=ORIENTED_EDGE('',*,*,#12002,.F.);
#15975=ORIENTED_EDGE('',*,*,#12003,.T.);
#15976=ORIENTED_EDGE('',*,*,#12004,.F.);
#15977=ORIENTED_EDGE('',*,*,#12003,.F.);
#15978=ORIENTED_EDGE('',*,*,#12005,.F.);
#15979=ORIENTED_EDGE('',*,*,#12006,.T.);
#15980=ORIENTED_EDGE('',*,*,#12007,.F.);
#15981=ORIENTED_EDGE('',*,*,#12006,.F.);
#15982=ORIENTED_EDGE('',*,*,#12008,.F.);
#15983=ORIENTED_EDGE('',*,*,#12009,.T.);
#15984=ORIENTED_EDGE('',*,*,#11943,.T.);
#15985=ORIENTED_EDGE('',*,*,#11939,.T.);
#15986=ORIENTED_EDGE('',*,*,#11936,.T.);
#15987=ORIENTED_EDGE('',*,*,#11933,.T.);
#15988=ORIENTED_EDGE('',*,*,#11930,.T.);
#15989=ORIENTED_EDGE('',*,*,#12010,.T.);
#15990=ORIENTED_EDGE('',*,*,#12011,.T.);
#15991=ORIENTED_EDGE('',*,*,#12012,.T.);
#15992=ORIENTED_EDGE('',*,*,#12013,.T.);
#15993=ORIENTED_EDGE('',*,*,#12014,.T.);
#15994=ORIENTED_EDGE('',*,*,#11941,.T.);
#15995=ORIENTED_EDGE('',*,*,#12015,.T.);
#15996=ORIENTED_EDGE('',*,*,#12008,.T.);
#15997=ORIENTED_EDGE('',*,*,#12005,.T.);
#15998=ORIENTED_EDGE('',*,*,#12002,.T.);
#15999=ORIENTED_EDGE('',*,*,#11940,.T.);
#16000=ORIENTED_EDGE('',*,*,#12009,.F.);
#16001=ORIENTED_EDGE('',*,*,#12015,.F.);
#16002=ORIENTED_EDGE('',*,*,#12016,.F.);
#16003=ORIENTED_EDGE('',*,*,#11928,.F.);
#16004=ORIENTED_EDGE('',*,*,#11932,.F.);
#16005=ORIENTED_EDGE('',*,*,#11935,.F.);
#16006=ORIENTED_EDGE('',*,*,#11938,.F.);
#16007=ORIENTED_EDGE('',*,*,#11942,.F.);
#16008=ORIENTED_EDGE('',*,*,#12014,.F.);
#16009=ORIENTED_EDGE('',*,*,#12017,.T.);
#16010=ORIENTED_EDGE('',*,*,#12018,.F.);
#16011=ORIENTED_EDGE('',*,*,#12017,.F.);
#16012=ORIENTED_EDGE('',*,*,#12013,.F.);
#16013=ORIENTED_EDGE('',*,*,#12019,.T.);
#16014=ORIENTED_EDGE('',*,*,#12020,.F.);
#16015=ORIENTED_EDGE('',*,*,#12019,.F.);
#16016=ORIENTED_EDGE('',*,*,#12012,.F.);
#16017=ORIENTED_EDGE('',*,*,#12001,.T.);
#16018=ORIENTED_EDGE('',*,*,#12021,.F.);
#16019=ORIENTED_EDGE('',*,*,#12022,.T.);
#16020=ORIENTED_EDGE('',*,*,#12023,.F.);
#16021=ORIENTED_EDGE('',*,*,#12024,.F.);
#16022=ORIENTED_EDGE('',*,*,#12025,.F.);
#16023=ORIENTED_EDGE('',*,*,#12026,.F.);
#16024=ORIENTED_EDGE('',*,*,#12027,.F.);
#16025=ORIENTED_EDGE('',*,*,#12028,.F.);
#16026=ORIENTED_EDGE('',*,*,#12029,.F.);
#16027=ORIENTED_EDGE('',*,*,#12022,.F.);
#16028=ORIENTED_EDGE('',*,*,#12027,.T.);
#16029=ORIENTED_EDGE('',*,*,#12030,.T.);
#16030=ORIENTED_EDGE('',*,*,#12031,.T.);
#16031=ORIENTED_EDGE('',*,*,#12032,.F.);
#16032=ORIENTED_EDGE('',*,*,#12026,.T.);
#16033=ORIENTED_EDGE('',*,*,#12033,.T.);
#16034=ORIENTED_EDGE('',*,*,#12034,.T.);
#16035=ORIENTED_EDGE('',*,*,#12030,.F.);
#16036=ORIENTED_EDGE('',*,*,#12025,.T.);
#16037=ORIENTED_EDGE('',*,*,#12035,.T.);
#16038=ORIENTED_EDGE('',*,*,#12036,.T.);
#16039=ORIENTED_EDGE('',*,*,#12033,.F.);
#16040=ORIENTED_EDGE('',*,*,#12031,.F.);
#16041=ORIENTED_EDGE('',*,*,#12034,.F.);
#16042=ORIENTED_EDGE('',*,*,#12036,.F.);
#16043=ORIENTED_EDGE('',*,*,#12037,.F.);
#16044=ORIENTED_EDGE('',*,*,#12038,.F.);
#16045=ORIENTED_EDGE('',*,*,#12039,.T.);
#16046=ORIENTED_EDGE('',*,*,#12040,.F.);
#16047=ORIENTED_EDGE('',*,*,#12039,.F.);
#16048=ORIENTED_EDGE('',*,*,#12041,.F.);
#16049=ORIENTED_EDGE('',*,*,#12042,.F.);
#16050=ORIENTED_EDGE('',*,*,#12024,.T.);
#16051=ORIENTED_EDGE('',*,*,#12043,.T.);
#16052=ORIENTED_EDGE('',*,*,#12037,.T.);
#16053=ORIENTED_EDGE('',*,*,#12035,.F.);
#16054=ORIENTED_EDGE('',*,*,#12040,.T.);
#16055=ORIENTED_EDGE('',*,*,#11997,.T.);
#16056=ORIENTED_EDGE('',*,*,#11995,.T.);
#16057=ORIENTED_EDGE('',*,*,#11993,.T.);
#16058=ORIENTED_EDGE('',*,*,#11946,.F.);
#16059=ORIENTED_EDGE('',*,*,#12044,.F.);
#16060=ORIENTED_EDGE('',*,*,#12021,.T.);
#16061=ORIENTED_EDGE('',*,*,#12045,.F.);
#16062=ORIENTED_EDGE('',*,*,#12046,.F.);
#16063=ORIENTED_EDGE('',*,*,#12028,.T.);
#16064=ORIENTED_EDGE('',*,*,#12032,.T.);
#16065=ORIENTED_EDGE('',*,*,#12042,.T.);
#16066=ORIENTED_EDGE('',*,*,#12047,.F.);
#16067=ORIENTED_EDGE('',*,*,#12023,.T.);
#16068=ORIENTED_EDGE('',*,*,#12029,.T.);
#16069=ORIENTED_EDGE('',*,*,#12047,.T.);
#16070=ORIENTED_EDGE('',*,*,#12041,.T.);
#16071=ORIENTED_EDGE('',*,*,#12038,.T.);
#16072=ORIENTED_EDGE('',*,*,#12043,.F.);
#16073=ORIENTED_EDGE('',*,*,#12046,.T.);
#16074=ORIENTED_EDGE('',*,*,#12048,.T.);
#16075=ORIENTED_EDGE('',*,*,#12049,.F.);
#16076=ORIENTED_EDGE('',*,*,#12048,.F.);
#16077=ORIENTED_EDGE('',*,*,#12050,.T.);
#16078=ORIENTED_EDGE('',*,*,#12051,.T.);
#16079=ORIENTED_EDGE('',*,*,#12044,.T.);
#16080=ORIENTED_EDGE('',*,*,#12051,.F.);
#16081=ORIENTED_EDGE('',*,*,#12052,.F.);
#16082=ORIENTED_EDGE('',*,*,#12049,.T.);
#16083=ORIENTED_EDGE('',*,*,#12010,.F.);
#16084=ORIENTED_EDGE('',*,*,#12011,.F.);
#16085=ORIENTED_EDGE('',*,*,#12053,.T.);
#16086=ORIENTED_EDGE('',*,*,#12052,.T.);
#16087=ORIENTED_EDGE('',*,*,#12053,.F.);
#16088=ORIENTED_EDGE('',*,*,#12000,.T.);
#16089=ORIENTED_EDGE('',*,*,#12004,.T.);
#16090=ORIENTED_EDGE('',*,*,#12007,.T.);
#16091=ORIENTED_EDGE('',*,*,#11929,.T.);
#16092=ORIENTED_EDGE('',*,*,#12016,.T.);
#16093=ORIENTED_EDGE('',*,*,#12018,.T.);
#16094=ORIENTED_EDGE('',*,*,#12020,.T.);
#16095=ORIENTED_EDGE('',*,*,#12054,.F.);
#16096=ORIENTED_EDGE('',*,*,#12045,.T.);
#16097=ORIENTED_EDGE('',*,*,#12055,.T.);
#16098=ORIENTED_EDGE('',*,*,#12054,.T.);
#16099=ORIENTED_EDGE('',*,*,#12055,.F.);
#16100=ORIENTED_EDGE('',*,*,#12056,.F.);
#16101=ORIENTED_EDGE('',*,*,#12057,.T.);
#16102=ORIENTED_EDGE('',*,*,#11989,.T.);
#16103=ORIENTED_EDGE('',*,*,#11999,.T.);
#16104=ORIENTED_EDGE('',*,*,#11990,.T.);
#16105=ORIENTED_EDGE('',*,*,#12057,.F.);
#16106=ORIENTED_EDGE('',*,*,#12056,.T.);
#16107=ORIENTED_EDGE('',*,*,#12058,.F.);
#16108=ORIENTED_EDGE('',*,*,#12058,.T.);
#16109=ORIENTED_EDGE('',*,*,#12059,.T.);
#16110=ORIENTED_EDGE('',*,*,#12050,.F.);
#16111=ORIENTED_EDGE('',*,*,#12059,.F.);
#21354=CONICAL_SURFACE('',#23527,1.02473275573014,1.0471975511966);
#21355=CONICAL_SURFACE('',#23532,1.02473275573014,1.0471975511966);
#21356=CONICAL_SURFACE('',#23550,0.61785,0.785398163397448);
#21357=CONICAL_SURFACE('',#23554,0.67,0.785398163397446);
#21358=CONICAL_SURFACE('',#23558,0.39,0.20943951023932);
#21751=ADVANCED_FACE('',(#2921),#2446,.T.);
#21752=ADVANCED_FACE('',(#2922),#2447,.T.);
#21753=ADVANCED_FACE('',(#2923),#2448,.T.);
#21754=ADVANCED_FACE('',(#2924),#2449,.T.);
#21755=ADVANCED_FACE('',(#2925),#2450,.T.);
#21756=ADVANCED_FACE('',(#2926),#2451,.T.);
#21757=ADVANCED_FACE('',(#2927),#2452,.T.);
#21758=ADVANCED_FACE('',(#2928),#2453,.T.);
#21759=ADVANCED_FACE('',(#2929),#2454,.T.);
#21760=ADVANCED_FACE('',(#2930),#2455,.T.);
#21761=ADVANCED_FACE('',(#2931),#2456,.T.);
#21762=ADVANCED_FACE('',(#2932),#2457,.T.);
#21763=ADVANCED_FACE('',(#2933),#2458,.T.);
#21764=ADVANCED_FACE('',(#2934),#2459,.T.);
#21765=ADVANCED_FACE('',(#2935),#2460,.T.);
#21766=ADVANCED_FACE('',(#2936),#2461,.T.);
#21767=ADVANCED_FACE('',(#2937),#2462,.T.);
#21768=ADVANCED_FACE('',(#2938),#2463,.T.);
#21769=ADVANCED_FACE('',(#2939),#2464,.T.);
#21770=ADVANCED_FACE('',(#2940),#1975,.F.);
#21771=ADVANCED_FACE('',(#2941),#324,.F.);
#21772=ADVANCED_FACE('',(#2942),#2465,.T.);
#21773=ADVANCED_FACE('',(#2943),#325,.F.);
#21774=ADVANCED_FACE('',(#2944),#2466,.T.);
#21775=ADVANCED_FACE('',(#2945),#326,.T.);
#21776=ADVANCED_FACE('',(#2946),#327,.F.);
#21777=ADVANCED_FACE('',(#2947),#328,.F.);
#21778=ADVANCED_FACE('',(#2948),#1976,.T.);
#21779=ADVANCED_FACE('',(#2949),#2467,.T.);
#21780=ADVANCED_FACE('',(#2950),#329,.F.);
#21781=ADVANCED_FACE('',(#2951),#330,.F.);
#21782=ADVANCED_FACE('',(#2952),#331,.T.);
#21783=ADVANCED_FACE('',(#2953),#21354,.T.);
#21784=ADVANCED_FACE('',(#2954),#1977,.T.);
#21785=ADVANCED_FACE('',(#2955),#1978,.T.);
#21786=ADVANCED_FACE('',(#2956),#1979,.T.);
#21787=ADVANCED_FACE('',(#2957),#21355,.T.);
#21788=ADVANCED_FACE('',(#2958),#1980,.T.);
#21789=ADVANCED_FACE('',(#2959,#1634),#1981,.T.);
#21790=ADVANCED_FACE('',(#2960),#1982,.T.);
#21791=ADVANCED_FACE('',(#2961,#1635),#1983,.F.);
#21792=ADVANCED_FACE('',(#2962),#1984,.F.);
#21793=ADVANCED_FACE('',(#2963),#1985,.T.);
#21794=ADVANCED_FACE('',(#2964),#1986,.T.);
#21795=ADVANCED_FACE('',(#2965),#2468,.F.);
#21796=ADVANCED_FACE('',(#2966),#2469,.F.);
#21797=ADVANCED_FACE('',(#2967,#1636),#1987,.T.);
#21798=ADVANCED_FACE('',(#2968),#21356,.T.);
#21799=ADVANCED_FACE('',(#2969,#1637),#1988,.T.);
#21800=ADVANCED_FACE('',(#2970),#2470,.T.);
#21801=ADVANCED_FACE('',(#2971),#21357,.T.);
#21802=ADVANCED_FACE('',(#2972,#1638),#1989,.T.);
#21803=ADVANCED_FACE('',(#2973),#21358,.F.);
#22811=CLOSED_SHELL('',(#21751,#21752,#21753,#21754,#21755,#21756,#21757,
#21758,#21759,#21760,#21761,#21762,#21763,#21764,#21765,#21766,#21767,#21768,
#21769,#21770,#21771,#21772,#21773,#21774,#21775,#21776,#21777,#21778,#21779,
#21780,#21781,#21782,#21783,#21784,#21785,#21786,#21787,#21788,#21789,#21790,
#21791,#21792,#21793,#21794,#21795,#21796,#21797,#21798,#21799,#21800,#21801,
#21802,#21803));
#23491=AXIS2_PLACEMENT_3D('',#37140,#26342,#26343);
#23492=AXIS2_PLACEMENT_3D('',#37141,#26344,#26345);
#23493=AXIS2_PLACEMENT_3D('',#37158,#26347,#26348);
#23494=AXIS2_PLACEMENT_3D('',#37169,#26349,#26350);
#23495=AXIS2_PLACEMENT_3D('',#37207,#26352,#26353);
#23496=AXIS2_PLACEMENT_3D('',#37245,#26355,#26356);
#23497=AXIS2_PLACEMENT_3D('',#37283,#26358,#26359);
#23498=AXIS2_PLACEMENT_3D('',#37288,#26361,#26362);
#23499=AXIS2_PLACEMENT_3D('',#37322,#26363,#26364);
#23500=AXIS2_PLACEMENT_3D('',#37344,#26366,#26367);
#23501=AXIS2_PLACEMENT_3D('',#37355,#26368,#26369);
#23502=AXIS2_PLACEMENT_3D('',#37439,#26371,#26372);
#23503=AXIS2_PLACEMENT_3D('',#37529,#26374,#26375);
#23504=AXIS2_PLACEMENT_3D('',#37613,#26377,#26378);
#23505=AXIS2_PLACEMENT_3D('',#37703,#26380,#26381);
#23506=AXIS2_PLACEMENT_3D('',#37793,#26383,#26384);
#23507=AXIS2_PLACEMENT_3D('',#37877,#26386,#26387);
#23508=AXIS2_PLACEMENT_3D('',#37891,#26389,#26390);
#23509=AXIS2_PLACEMENT_3D('',#37897,#26391,#26392);
#23510=AXIS2_PLACEMENT_3D('',#37934,#26394,#26395);
#23511=AXIS2_PLACEMENT_3D('',#37971,#26397,#26398);
#23512=AXIS2_PLACEMENT_3D('',#38009,#26400,#26401);
#23513=AXIS2_PLACEMENT_3D('',#38046,#26403,#26404);
#23514=AXIS2_PLACEMENT_3D('',#38083,#26406,#26407);
#23515=AXIS2_PLACEMENT_3D('',#38120,#26409,#26410);
#23516=AXIS2_PLACEMENT_3D('',#38196,#26411,#26412);
#23517=AXIS2_PLACEMENT_3D('',#38198,#26413,#26414);
#23518=AXIS2_PLACEMENT_3D('',#38774,#26415,#26416);
#23519=AXIS2_PLACEMENT_3D('',#38776,#26417,#26418);
#23520=AXIS2_PLACEMENT_3D('',#39270,#26419,#26420);
#23521=AXIS2_PLACEMENT_3D('',#39271,#26421,#26422);
#23522=AXIS2_PLACEMENT_3D('',#40593,#26423,#26424);
#23523=AXIS2_PLACEMENT_3D('',#40595,#26425,#26426);
#23524=AXIS2_PLACEMENT_3D('',#40596,#26427,#26428);
#23525=AXIS2_PLACEMENT_3D('',#40662,#26429,#26430);
#23526=AXIS2_PLACEMENT_3D('',#40663,#26431,#26432);
#23527=AXIS2_PLACEMENT_3D('',#41734,#26433,#26434);
#23528=AXIS2_PLACEMENT_3D('',#41736,#26435,#26436);
#23529=AXIS2_PLACEMENT_3D('',#41766,#26438,#26439);
#23530=AXIS2_PLACEMENT_3D('',#41774,#26442,#26443);
#23531=AXIS2_PLACEMENT_3D('',#41780,#26445,#26446);
#23532=AXIS2_PLACEMENT_3D('',#41786,#26448,#26449);
#23533=AXIS2_PLACEMENT_3D('',#41797,#26451,#26452);
#23534=AXIS2_PLACEMENT_3D('',#41805,#26453,#26454);
#23535=AXIS2_PLACEMENT_3D('',#41807,#26456,#26457);
#23536=AXIS2_PLACEMENT_3D('',#41808,#26458,#26459);
#23537=AXIS2_PLACEMENT_3D('',#41810,#26460,#26461);
#23538=AXIS2_PLACEMENT_3D('',#41811,#26462,#26463);
#23539=AXIS2_PLACEMENT_3D('',#41813,#26464,#26465);
#23540=AXIS2_PLACEMENT_3D('',#41814,#26466,#26467);
#23541=AXIS2_PLACEMENT_3D('',#41816,#26468,#26469);
#23542=AXIS2_PLACEMENT_3D('',#41817,#26470,#26471);
#23543=AXIS2_PLACEMENT_3D('',#41819,#26473,#26474);
#23544=AXIS2_PLACEMENT_3D('',#41820,#26475,#26476);
#23545=AXIS2_PLACEMENT_3D('',#41823,#26478,#26479);
#23546=AXIS2_PLACEMENT_3D('',#41824,#26480,#26481);
#23547=AXIS2_PLACEMENT_3D('',#41826,#26482,#26483);
#23548=AXIS2_PLACEMENT_3D('',#41828,#26485,#26486);
#23549=AXIS2_PLACEMENT_3D('',#41830,#26487,#26488);
#23550=AXIS2_PLACEMENT_3D('',#41831,#26489,#26490);
#23551=AXIS2_PLACEMENT_3D('',#41833,#26492,#26493);
#23552=AXIS2_PLACEMENT_3D('',#41835,#26494,#26495);
#23553=AXIS2_PLACEMENT_3D('',#41836,#26496,#26497);
#23554=AXIS2_PLACEMENT_3D('',#41838,#26499,#26500);
#23555=AXIS2_PLACEMENT_3D('',#41840,#26501,#26502);
#23556=AXIS2_PLACEMENT_3D('',#41842,#26504,#26505);
#23557=AXIS2_PLACEMENT_3D('',#41844,#26506,#26507);
#23558=AXIS2_PLACEMENT_3D('',#41845,#26508,#26509);
#26342=DIRECTION('axis',(0.,0.,1.));
#26343=DIRECTION('refdir',(1.,0.,0.));
#26344=DIRECTION('center_axis',(0.,0.,1.));
#26345=DIRECTION('ref_axis',(0.185354282886115,-0.982671760974016,0.));
#26346=DIRECTION('',(0.,0.,1.));
#26347=DIRECTION('center_axis',(0.,0.,1.));
#26348=DIRECTION('ref_axis',(1.,-1.15782485934285E-14,0.));
#26349=DIRECTION('center_axis',(0.,0.,1.));
#26350=DIRECTION('ref_axis',(1.,-1.15782485934285E-14,0.));
#26351=DIRECTION('',(0.,0.,1.));
#26352=DIRECTION('center_axis',(0.,0.,1.));
#26353=DIRECTION('ref_axis',(1.,-1.15782485934285E-14,0.));
#26354=DIRECTION('',(0.,0.,1.));
#26355=DIRECTION('center_axis',(0.,0.,1.));
#26356=DIRECTION('ref_axis',(1.,-1.15782485934285E-14,0.));
#26357=DIRECTION('',(0.,0.,1.));
#26358=DIRECTION('center_axis',(0.,0.,1.));
#26359=DIRECTION('ref_axis',(1.,-1.15782485934285E-14,0.));
#26360=DIRECTION('',(0.,0.,1.));
#26361=DIRECTION('center_axis',(0.,0.,-1.));
#26362=DIRECTION('ref_axis',(1.,-1.15782485934285E-14,0.));
#26363=DIRECTION('center_axis',(0.,0.,1.));
#26364=DIRECTION('ref_axis',(1.,0.,0.));
#26365=DIRECTION('',(0.,0.,-1.));
#26366=DIRECTION('center_axis',(0.,0.,-1.));
#26367=DIRECTION('ref_axis',(1.,0.,0.));
#26368=DIRECTION('center_axis',(0.,0.,1.));
#26369=DIRECTION('ref_axis',(1.,0.,0.));
#26370=DIRECTION('',(0.,0.,-1.));
#26371=DIRECTION('center_axis',(0.,0.,1.));
#26372=DIRECTION('ref_axis',(1.,0.,0.));
#26373=DIRECTION('',(0.,0.,-1.));
#26374=DIRECTION('center_axis',(0.,0.,1.));
#26375=DIRECTION('ref_axis',(1.,0.,0.));
#26376=DIRECTION('',(0.,0.,-1.));
#26377=DIRECTION('center_axis',(0.,0.,1.));
#26378=DIRECTION('ref_axis',(1.,0.,0.));
#26379=DIRECTION('',(0.,0.,-1.));
#26380=DIRECTION('center_axis',(0.,0.,1.));
#26381=DIRECTION('ref_axis',(1.,0.,0.));
#26382=DIRECTION('',(0.,0.,-1.));
#26383=DIRECTION('center_axis',(0.,0.,1.));
#26384=DIRECTION('ref_axis',(1.,0.,0.));
#26385=DIRECTION('',(0.,0.,-1.));
#26386=DIRECTION('center_axis',(0.,0.,1.));
#26387=DIRECTION('ref_axis',(-0.503961761468012,-0.863725965210065,0.));
#26388=DIRECTION('',(0.,0.,1.));
#26389=DIRECTION('center_axis',(0.,0.,1.));
#26390=DIRECTION('ref_axis',(1.,2.05501931194342E-14,0.));
#26391=DIRECTION('center_axis',(0.,0.,1.));
#26392=DIRECTION('ref_axis',(1.,2.05501931194342E-14,0.));
#26393=DIRECTION('',(0.,0.,1.));
#26394=DIRECTION('center_axis',(0.,0.,1.));
#26395=DIRECTION('ref_axis',(1.,2.05501931194342E-14,0.));
#26396=DIRECTION('',(0.,0.,1.));
#26397=DIRECTION('center_axis',(0.,0.,1.));
#26398=DIRECTION('ref_axis',(1.,2.05501931194342E-14,0.));
#26399=DIRECTION('',(0.,0.,1.));
#26400=DIRECTION('center_axis',(0.,0.,1.));
#26401=DIRECTION('ref_axis',(1.,2.05501931194342E-14,0.));
#26402=DIRECTION('',(0.,0.,1.));
#26403=DIRECTION('center_axis',(0.,0.,1.));
#26404=DIRECTION('ref_axis',(1.,2.05501931194342E-14,0.));
#26405=DIRECTION('',(0.,0.,1.));
#26406=DIRECTION('center_axis',(0.,0.,1.));
#26407=DIRECTION('ref_axis',(1.,2.05501931194342E-14,0.));
#26408=DIRECTION('',(0.,0.,1.));
#26409=DIRECTION('center_axis',(0.,0.,1.));
#26410=DIRECTION('ref_axis',(1.,0.,0.));
#26411=DIRECTION('center_axis',(0.,0.,-1.));
#26412=DIRECTION('ref_axis',(1.,0.,0.));
#26413=DIRECTION('center_axis',(0.,0.,-1.));
#26414=DIRECTION('ref_axis',(1.,0.,0.));
#26415=DIRECTION('center_axis',(0.,0.,1.));
#26416=DIRECTION('ref_axis',(0.888916624476397,0.458069028345607,0.));
#26417=DIRECTION('center_axis',(0.,0.,-1.));
#26418=DIRECTION('ref_axis',(1.,2.05501931194342E-14,0.));
#26419=DIRECTION('center_axis',(0.,0.,1.));
#26420=DIRECTION('ref_axis',(1.,0.,0.));
#26421=DIRECTION('center_axis',(0.,0.,-1.));
#26422=DIRECTION('ref_axis',(1.,0.,0.));
#26423=DIRECTION('center_axis',(0.,0.,1.));
#26424=DIRECTION('ref_axis',(1.,0.,0.));
#26425=DIRECTION('center_axis',(0.,0.,1.));
#26426=DIRECTION('ref_axis',(1.,0.,0.));
#26427=DIRECTION('center_axis',(0.,0.,1.));
#26428=DIRECTION('ref_axis',(1.,0.,0.));
#26429=DIRECTION('center_axis',(0.,0.,-1.));
#26430=DIRECTION('ref_axis',(1.,-1.15782485934285E-14,0.));
#26431=DIRECTION('center_axis',(0.,0.,1.));
#26432=DIRECTION('ref_axis',(-0.997062746034551,0.0765890362260817,0.));
#26433=DIRECTION('center_axis',(0.,0.,1.));
#26434=DIRECTION('ref_axis',(1.,0.,0.));
#26435=DIRECTION('center_axis',(0.,0.,-1.));
#26436=DIRECTION('ref_axis',(1.,0.,0.));
#26437=DIRECTION('',(-0.866025403784439,-1.06057523872491E-16,0.5));
#26438=DIRECTION('center_axis',(0.5,-0.866025403784439,0.));
#26439=DIRECTION('ref_axis',(0.866025403784439,0.5,0.));
#26440=DIRECTION('',(0.,0.,1.));
#26441=DIRECTION('',(0.,0.,1.));
#26442=DIRECTION('center_axis',(1.,-3.03625687323721E-16,0.));
#26443=DIRECTION('ref_axis',(3.03625687323721E-16,1.,0.));
#26444=DIRECTION('',(0.,0.,1.));
#26445=DIRECTION('center_axis',(0.5,0.866025403784439,0.));
#26446=DIRECTION('ref_axis',(-0.866025403784439,0.5,0.));
#26447=DIRECTION('',(0.,0.,1.));
#26448=DIRECTION('center_axis',(0.,0.,-1.));
#26449=DIRECTION('ref_axis',(1.,0.,0.));
#26450=DIRECTION('',(0.866025403784439,1.06057523872491E-16,0.5));
#26451=DIRECTION('center_axis',(0.,0.,1.));
#26452=DIRECTION('ref_axis',(1.,0.,0.));
#26453=DIRECTION('center_axis',(-0.5,0.866025403784439,0.));
#26454=DIRECTION('ref_axis',(-0.866025403784439,-0.5,0.));
#26455=DIRECTION('',(0.,0.,1.));
#26456=DIRECTION('center_axis',(0.,0.,1.));
#26457=DIRECTION('ref_axis',(1.,0.,0.));
#26458=DIRECTION('center_axis',(0.,0.,1.));
#26459=DIRECTION('ref_axis',(1.,0.,0.));
#26460=DIRECTION('center_axis',(0.,0.,-1.));
#26461=DIRECTION('ref_axis',(1.,0.,0.));
#26462=DIRECTION('center_axis',(0.,0.,1.));
#26463=DIRECTION('ref_axis',(1.,0.,0.));
#26464=DIRECTION('center_axis',(0.,0.,-1.));
#26465=DIRECTION('ref_axis',(1.,0.,0.));
#26466=DIRECTION('center_axis',(0.,0.,1.));
#26467=DIRECTION('ref_axis',(1.,0.,0.));
#26468=DIRECTION('center_axis',(0.,0.,1.));
#26469=DIRECTION('ref_axis',(1.,0.,0.));
#26470=DIRECTION('center_axis',(-0.5,-0.866025403784439,0.));
#26471=DIRECTION('ref_axis',(0.866025403784439,-0.5,0.));
#26472=DIRECTION('',(0.,0.,1.));
#26473=DIRECTION('center_axis',(-1.,-2.0241712488248E-16,0.));
#26474=DIRECTION('ref_axis',(2.0241712488248E-16,-1.,0.));
#26475=DIRECTION('center_axis',(0.,0.,1.));
#26476=DIRECTION('ref_axis',(1.,0.,0.));
#26477=DIRECTION('',(0.,0.,-1.));
#26478=DIRECTION('center_axis',(0.,0.,1.));
#26479=DIRECTION('ref_axis',(1.,0.,0.));
#26480=DIRECTION('center_axis',(0.,0.,1.));
#26481=DIRECTION('ref_axis',(1.,0.,0.));
#26482=DIRECTION('center_axis',(0.,0.,1.));
#26483=DIRECTION('ref_axis',(1.,0.,0.));
#26484=DIRECTION('',(0.,0.,-1.));
#26485=DIRECTION('center_axis',(0.,0.,-1.));
#26486=DIRECTION('ref_axis',(-1.,0.,0.));
#26487=DIRECTION('center_axis',(0.,0.,1.));
#26488=DIRECTION('ref_axis',(1.,0.,0.));
#26489=DIRECTION('center_axis',(0.,0.,1.));
#26490=DIRECTION('ref_axis',(1.,0.,0.));
#26491=DIRECTION('',(0.707106781186548,8.65956056235493E-17,-0.707106781186548));
#26492=DIRECTION('center_axis',(0.,0.,1.));
#26493=DIRECTION('ref_axis',(1.,0.,0.));
#26494=DIRECTION('center_axis',(0.,0.,1.));
#26495=DIRECTION('ref_axis',(1.,0.,0.));
#26496=DIRECTION('center_axis',(0.,0.,1.));
#26497=DIRECTION('ref_axis',(1.,0.,0.));
#26498=DIRECTION('',(0.,0.,-1.));
#26499=DIRECTION('center_axis',(0.,0.,-1.));
#26500=DIRECTION('ref_axis',(1.,0.,0.));
#26501=DIRECTION('center_axis',(0.,0.,1.));
#26502=DIRECTION('ref_axis',(1.,0.,0.));
#26503=DIRECTION('',(-0.707106781186546,-8.65956056235491E-17,-0.707106781186549));
#26504=DIRECTION('center_axis',(0.,0.,1.));
#26505=DIRECTION('ref_axis',(1.,0.,0.));
#26506=DIRECTION('center_axis',(0.,0.,1.));
#26507=DIRECTION('ref_axis',(1.,0.,0.));
#26508=DIRECTION('center_axis',(0.,0.,1.));
#26509=DIRECTION('ref_axis',(1.,0.,0.));
#26510=DIRECTION('',(0.207911690817759,2.54618386665283E-17,-0.978147600733806));
#37140=CARTESIAN_POINT('',(0.,0.,0.));
#37141=CARTESIAN_POINT('Origin',(0.,0.,-0.930039011722494));
#37142=CARTESIAN_POINT('',(-0.572251846808819,1.31896832121565E-5,-0.194775853827758));
#37143=CARTESIAN_POINT('',(-0.572209896248783,5.87811292650231E-6,-0.188250461961717));
#37144=CARTESIAN_POINT('',(-0.57225,6.55557234450825E-15,-0.930039011722494));
#37145=CARTESIAN_POINT('',(0.532887356432457,0.208459172818158,-0.12));
#37146=CARTESIAN_POINT('Ctrl Pts',(-0.572251846808819,1.31896832121572E-5,
-0.194775853827758));
#37147=CARTESIAN_POINT('Ctrl Pts',(-0.572182461406416,-0.0721591436399304,
-0.192092383539388));
#37148=CARTESIAN_POINT('Ctrl Pts',(-0.540797694659007,-0.237406800584547,
-0.185950422500778));
#37149=CARTESIAN_POINT('Ctrl Pts',(-0.385757245550577,-0.453572246869937,
-0.176349970711929));
#37150=CARTESIAN_POINT('Ctrl Pts',(-0.128270146612636,-0.581450425290948,
-0.165974498461211));
#37151=CARTESIAN_POINT('Ctrl Pts',(0.159119430707533,-0.573773118428659,
-0.155599026210492));
#37152=CARTESIAN_POINT('Ctrl Pts',(0.409415432322886,-0.432341853180699,
-0.145223553959774));
#37153=CARTESIAN_POINT('Ctrl Pts',(0.56426305151595,-0.190104706888137,
-0.134848081709056));
#37154=CARTESIAN_POINT('Ctrl Pts',(0.583151179466301,0.0420829677627029,
-0.126440230389131));
#37155=CARTESIAN_POINT('Ctrl Pts',(0.54751143363328,0.171111722668445,-0.121490869819446));
#37156=CARTESIAN_POINT('Ctrl Pts',(0.532887356432457,0.208459172818158,
-0.12));
#37157=CARTESIAN_POINT('',(0.570996795169322,0.0378513197440182,-0.12));
#37158=CARTESIAN_POINT('Origin',(0.,0.,-0.12));
#37159=CARTESIAN_POINT('Ctrl Pts',(-0.572209896248783,5.87811292651272E-6,
-0.188250461961717));
#37160=CARTESIAN_POINT('Ctrl Pts',(-0.572189385338301,-0.0537745726271744,
-0.186251252475915));
#37161=CARTESIAN_POINT('Ctrl Pts',(-0.551638057130558,-0.200606777068497,
-0.180793552239873));
#37162=CARTESIAN_POINT('Ctrl Pts',(-0.427655041590171,-0.414301519355521,
-0.171877361253592));
#37163=CARTESIAN_POINT('Ctrl Pts',(-0.183688600698895,-0.566391183638125,
-0.161501889002873));
#37164=CARTESIAN_POINT('Ctrl Pts',(0.103112831945545,-0.586430161623632,
-0.151126416752155));
#37165=CARTESIAN_POINT('Ctrl Pts',(0.365851355459577,-0.469776284513869,
-0.140750944501437));
#37166=CARTESIAN_POINT('Ctrl Pts',(0.543351022386391,-0.243565284402786,
-0.130375472250718));
#37167=CARTESIAN_POINT('Ctrl Pts',(0.577149518655877,-0.0549640805153465,
-0.123458490750239));
#37168=CARTESIAN_POINT('Ctrl Pts',(0.570996795169322,0.0378513197440182,
-0.12));
#37169=CARTESIAN_POINT('Origin',(0.,0.,-0.930039011722494));
#37170=CARTESIAN_POINT('',(-0.572223068770992,1.08892936001897E-5,-0.328460064354073));
#37171=CARTESIAN_POINT('',(-0.572206446074254,-2.92925376449427E-6,-0.321934672488033));
#37172=CARTESIAN_POINT('',(-0.57225,6.55557234450825E-15,-0.930039011722494));
#37173=CARTESIAN_POINT('Ctrl Pts',(-0.572223068770992,1.08892936001997E-5,
-0.328460064354073));
#37174=CARTESIAN_POINT('Ctrl Pts',(-0.572178592440248,-0.0614397738734596,
-0.326175570310044));
#37175=CARTESIAN_POINT('Ctrl Pts',(-0.547362804764057,-0.215955547533754,
-0.320432585515775));
#37176=CARTESIAN_POINT('Ctrl Pts',(-0.410649598305695,-0.431165515585077,
-0.311231109971268));
#37177=CARTESIAN_POINT('Ctrl Pts',(-0.160760107350392,-0.57331752294948,
-0.300855637720549));
#37178=CARTESIAN_POINT('Ctrl Pts',(0.126606838000238,-0.581813976495778,
-0.290480165469831));
#37179=CARTESIAN_POINT('Ctrl Pts',(0.3844583637991,-0.454674125457656,-0.280104693219112));
#37180=CARTESIAN_POINT('Ctrl Pts',(0.552682425815823,-0.221537651868143,
-0.269729220968394));
#37181=CARTESIAN_POINT('Ctrl Pts',(0.592061522393167,0.0632451413900827,
-0.259353748717676));
#37182=CARTESIAN_POINT('Ctrl Pts',(0.493415341577429,0.333283802752439,
-0.248978276466957));
#37183=CARTESIAN_POINT('Ctrl Pts',(0.279740925892577,0.525625166857998,
-0.238602804216239));
#37184=CARTESIAN_POINT('Ctrl Pts',(0.000851470205678055,0.595429299999864,
-0.228227331965521));
#37185=CARTESIAN_POINT('Ctrl Pts',(-0.278236497349112,0.526423100377946,
-0.217851859714802));
#37186=CARTESIAN_POINT('Ctrl Pts',(-0.492460118502939,0.334693554718123,
-0.207476387464084));
#37187=CARTESIAN_POINT('Ctrl Pts',(-0.56616513883061,0.134706710058056,
-0.199784385501736));
#37188=CARTESIAN_POINT('Ctrl Pts',(-0.57227188619843,0.020857480506449,
-0.195550874289627));
#37189=CARTESIAN_POINT('Ctrl Pts',(-0.572251846808819,1.31896832121572E-5,
-0.194775853827758));
#37190=CARTESIAN_POINT('Ctrl Pts',(-0.572206446074254,-2.92925376450121E-6,
-0.321934672488033));
#37191=CARTESIAN_POINT('Ctrl Pts',(-0.572214485737319,-0.0430512316554342,
-0.320334439246571));
#37192=CARTESIAN_POINT('Ctrl Pts',(-0.557042913275609,-0.179131739323211,
-0.31527571525487));
#37193=CARTESIAN_POINT('Ctrl Pts',(-0.450274644860222,-0.389601769278859,
-0.30675850051293));
#37194=CARTESIAN_POINT('Ctrl Pts',(-0.215241042075345,-0.555164919115264,
-0.296383028262211));
#37195=CARTESIAN_POINT('Ctrl Pts',(0.0699709674208999,-0.591304370416951,
-0.286007556011493));
#37196=CARTESIAN_POINT('Ctrl Pts',(0.338870887774159,-0.489595052448449,
-0.275632083760774));
#37197=CARTESIAN_POINT('Ctrl Pts',(0.528770989858389,-0.273748118747132,
-0.265256611510057));
#37198=CARTESIAN_POINT('Ctrl Pts',(0.595400531599021,0.00591678855841044,
-0.254881139259338));
#37199=CARTESIAN_POINT('Ctrl Pts',(0.523226356835316,0.284202314475096,
-0.24450566700862));
#37200=CARTESIAN_POINT('Ctrl Pts',(0.329074261287382,0.496232767362635,
-0.234130194757902));
#37201=CARTESIAN_POINT('Ctrl Pts',(0.0582061064454895,0.592578090033583,
-0.223754722507183));
#37202=CARTESIAN_POINT('Ctrl Pts',(-0.226231237425986,0.550777869717469,
-0.213379250256465));
#37203=CARTESIAN_POINT('Ctrl Pts',(-0.457928466129024,0.380576366952199,
-0.203003778005746));
#37204=CARTESIAN_POINT('Ctrl Pts',(-0.558795180707474,0.171543964843103,
-0.194627515240831));
#37205=CARTESIAN_POINT('Ctrl Pts',(-0.57222486776007,0.0392617963722867,
-0.189709743226154));
#37206=CARTESIAN_POINT('Ctrl Pts',(-0.572209896248783,5.87811292651272E-6,
-0.188250461961717));
#37207=CARTESIAN_POINT('Origin',(0.,0.,-0.930039011722494));
#37208=CARTESIAN_POINT('',(-0.57220691239729,3.53495086150753E-6,-0.462144274880389));
#37209=CARTESIAN_POINT('',(-0.572221465652637,-1.05155042379457E-5,-0.455618883014349));
#37210=CARTESIAN_POINT('',(-0.57225,6.55557234450825E-15,-0.930039011722494));
#37211=CARTESIAN_POINT('Ctrl Pts',(-0.57220691239729,3.53495086147584E-6,
-0.462144274880389));
#37212=CARTESIAN_POINT('Ctrl Pts',(-0.572195468328224,-0.0507191652367547,
-0.460258757080701));
#37213=CARTESIAN_POINT('Ctrl Pts',(-0.553245437112089,-0.194487822942528,
-0.454914748530773));
#37214=CARTESIAN_POINT('Ctrl Pts',(-0.434242783628202,-0.407394157101084,
-0.446112249230605));
#37215=CARTESIAN_POINT('Ctrl Pts',(-0.192741275441066,-0.563371631442748,
-0.435736776979888));
#37216=CARTESIAN_POINT('Ctrl Pts',(0.0936933474406337,-0.588012203120214,
-0.425361304729168));
#37217=CARTESIAN_POINT('Ctrl Pts',(0.35828556050624,-0.475571499888217,
-0.414985832478451));
#37218=CARTESIAN_POINT('Ctrl Pts',(0.539351885579122,-0.252262438534088,
-0.404610360227732));
#37219=CARTESIAN_POINT('Ctrl Pts',(0.594680949235049,0.0298557028055502,
-0.394234887977014));
#37220=CARTESIAN_POINT('Ctrl Pts',(0.511374075994885,0.30501368620711,-0.383859415726295));
#37221=CARTESIAN_POINT('Ctrl Pts',(0.308852312449722,0.509064871569989,
-0.373483943475578));
#37222=CARTESIAN_POINT('Ctrl Pts',(0.0343288650529642,0.594439503565886,
-0.363108471224859));
#37223=CARTESIAN_POINT('Ctrl Pts',(-0.248197553305573,0.5412344860607,-0.352732998974141));
#37224=CARTESIAN_POINT('Ctrl Pts',(-0.472862524479398,0.361853322940755,
-0.342357526723422));
#37225=CARTESIAN_POINT('Ctrl Pts',(-0.562095633396269,0.156185112186377,
-0.334266548516733));
#37226=CARTESIAN_POINT('Ctrl Pts',(-0.572245925064243,0.0315902564366742,
-0.329634061060284));
#37227=CARTESIAN_POINT('Ctrl Pts',(-0.572223068770992,1.08892936001997E-5,
-0.328460064354073));
#37228=CARTESIAN_POINT('Ctrl Pts',(-0.572221465652637,-1.051550423797E-5,
-0.455618883014349));
#37229=CARTESIAN_POINT('Ctrl Pts',(-0.572243953210631,-0.0323234178361406,
-0.454417626017228));
#37230=CARTESIAN_POINT('Ctrl Pts',(-0.561794458224291,-0.157652709186653,
-0.449757878269868));
#37231=CARTESIAN_POINT('Ctrl Pts',(-0.471468172615134,-0.363668195390408,
-0.441639639772268));
#37232=CARTESIAN_POINT('Ctrl Pts',(-0.24611537226857,-0.542184486739477,
-0.431264167521549));
#37233=CARTESIAN_POINT('Ctrl Pts',(0.0366134635183988,-0.594303162045059,
-0.420888695270832));
#37234=CARTESIAN_POINT('Ctrl Pts',(0.310806727710773,-0.507873972691536,
-0.410513223020113));
#37235=CARTESIAN_POINT('Ctrl Pts',(0.51254268190422,-0.30304586015049,-0.400137750769395));
#37236=CARTESIAN_POINT('Ctrl Pts',(0.594791312689474,-0.0275697021364228,
-0.389762278518676));
#37237=CARTESIAN_POINT('Ctrl Pts',(0.53837827792754,0.254333686297961,-0.379386806267958));
#37238=CARTESIAN_POINT('Ctrl Pts',(0.356454955565181,0.476945131829576,
-0.36901133401724));
#37239=CARTESIAN_POINT('Ctrl Pts',(0.0914325078965691,0.588367989131544,
-0.358635861766521));
#37240=CARTESIAN_POINT('Ctrl Pts',(-0.1949052878214,0.562626628325057,-0.348260389515803));
#37241=CARTESIAN_POINT('Ctrl Pts',(-0.435805479980445,0.405722044928676,
-0.337884917265085));
#37242=CARTESIAN_POINT('Ctrl Pts',(-0.553622904582432,0.19302062926978,
-0.329109678255828));
#37243=CARTESIAN_POINT('Ctrl Pts',(-0.572197110082555,0.0499865529700694,
-0.323792929996811));
#37244=CARTESIAN_POINT('Ctrl Pts',(-0.572206446074254,-2.92925376450121E-6,
-0.321934672488033));
#37245=CARTESIAN_POINT('Origin',(0.,0.,-0.930039011722494));
#37246=CARTESIAN_POINT('',(-0.572208961924848,-5.40006758461863E-6,-0.595828485406705));
#37247=CARTESIAN_POINT('',(-0.572249685678755,-1.32408837813236E-5,-0.589303093540665));
#37248=CARTESIAN_POINT('',(-0.57225,6.55557234450825E-15,-0.930039011722494));
#37249=CARTESIAN_POINT('Ctrl Pts',(-0.572208961924848,-5.40006758461067E-6,
-0.595828485406705));
#37250=CARTESIAN_POINT('Ctrl Pts',(-0.572222810317603,-0.0399947468816952,
-0.594341943851358));
#37251=CARTESIAN_POINT('Ctrl Pts',(-0.558462838001496,-0.173011307588341,
-0.589396911545771));
#37252=CARTESIAN_POINT('Ctrl Pts',(-0.4564620684611,-0.382333849583464,
-0.580993388489942));
#37253=CARTESIAN_POINT('Ctrl Pts',(-0.224112632886457,-0.551643292344488,
-0.570617916239226));
#37254=CARTESIAN_POINT('Ctrl Pts',(0.0604834222543564,-0.592350023747205,
-0.560242443988507));
#37255=CARTESIAN_POINT('Ctrl Pts',(0.330979180111506,-0.494964217078851,
-0.549866971737789));
#37256=CARTESIAN_POINT('Ctrl Pts',(0.524314895013938,-0.282189095361197,
-0.539491499487071));
#37257=CARTESIAN_POINT('Ctrl Pts',(0.595418869741894,-0.00362819397533901,
-0.529116027236352));
#37258=CARTESIAN_POINT('Ctrl Pts',(0.527714879176066,0.27577853563061,-0.518740554985634));
#37259=CARTESIAN_POINT('Ctrl Pts',(0.336986522471297,0.490893958039981,
-0.508365082734915));
#37260=CARTESIAN_POINT('Ctrl Pts',(0.0676976498285046,0.591568949974742,
-0.497989610484197));
#37261=CARTESIAN_POINT('Ctrl Pts',(-0.217373344570204,0.554333494794116,
-0.487614138233479));
#37262=CARTESIAN_POINT('Ctrl Pts',(-0.451768834165619,0.387868166836234,
-0.47723866598276));
#37263=CARTESIAN_POINT('Ctrl Pts',(-0.557388196836304,0.177664246876017,
-0.468748711531731));
#37264=CARTESIAN_POINT('Ctrl Pts',(-0.572216459488857,0.0423184021916877,
-0.46371724783094));
#37265=CARTESIAN_POINT('Ctrl Pts',(-0.57220691239729,3.53495086147584E-6,
-0.462144274880389));
#37266=CARTESIAN_POINT('Ctrl Pts',(-0.572249685678755,-1.32408837812507E-5,
-0.589303093540665));
#37267=CARTESIAN_POINT('Ctrl Pts',(-0.572270338122677,-0.0215909230762567,
-0.588500812787885));
#37268=CARTESIAN_POINT('Ctrl Pts',(-0.565907101669391,-0.136174074584614,
-0.584240041284865));
#37269=CARTESIAN_POINT('Ctrl Pts',(-0.491170026481974,-0.336584016022301,
-0.576520779031606));
#37270=CARTESIAN_POINT('Ctrl Pts',(-0.276211019809465,-0.527488640774144,
-0.566145306780888));
#37271=CARTESIAN_POINT('Ctrl Pts',(0.0031401178304551,-0.595421643954287,
-0.555769834530169));
#37272=CARTESIAN_POINT('Ctrl Pts',(0.281759210488034,-0.524546033533648,
-0.545394362279452));
#37273=CARTESIAN_POINT('Ctrl Pts',(0.494692741566129,-0.331384799915253,
-0.535018890028733));
#37274=CARTESIAN_POINT('Ctrl Pts',(0.59230024480053,-0.0609689603923613,
-0.524643417778015));
#37275=CARTESIAN_POINT('Ctrl Pts',(0.551826816631903,0.223660364318458,
-0.514267945527296));
#37276=CARTESIAN_POINT('Ctrl Pts',(0.382707889009843,0.456148512904055,
-0.503892473276577));
#37277=CARTESIAN_POINT('Ctrl Pts',(0.124369579435742,0.582296317894835,
-0.49351700102586));
#37278=CARTESIAN_POINT('Ctrl Pts',(-0.162962585060135,0.572695372777406,
-0.483141528775141));
#37279=CARTESIAN_POINT('Ctrl Pts',(-0.412303839155969,0.429583913041453,
-0.472766056524423));
#37280=CARTESIAN_POINT('Ctrl Pts',(-0.547786258426805,0.214489182365462,
-0.463591841270825));
#37281=CARTESIAN_POINT('Ctrl Pts',(-0.57217921018603,0.060707360836633,
-0.457876116767467));
#37282=CARTESIAN_POINT('Ctrl Pts',(-0.572221465652637,-1.051550423797E-5,
-0.455618883014349));
#37283=CARTESIAN_POINT('Origin',(0.,0.,-0.930039011722494));
#37284=CARTESIAN_POINT('',(-0.57225,6.55557234450825E-15,-0.72625));
#37285=CARTESIAN_POINT('',(-0.572279863946809,-1.0961849272878E-5,-0.722987304066981));
#37286=CARTESIAN_POINT('',(-0.57225,6.55557234450825E-15,-0.930039011722494));
#37287=CARTESIAN_POINT('',(-0.565534825602702,-0.0874095162469292,-0.72625));
#37288=CARTESIAN_POINT('Origin',(0.,0.,-0.72625));
#37289=CARTESIAN_POINT('Ctrl Pts',(-0.565534825602701,-0.0874095162469292,
-0.72625));
#37290=CARTESIAN_POINT('Ctrl Pts',(-0.551326428453064,-0.179337074585254,
-0.722791509249761));
#37291=CARTESIAN_POINT('Ctrl Pts',(-0.477265386956567,-0.356050729042777,
-0.715874527749281));
#37292=CARTESIAN_POINT('Ctrl Pts',(-0.254761663575757,-0.538176058210883,
-0.705499055498564));
#37293=CARTESIAN_POINT('Ctrl Pts',(0.0270755327719408,-0.594810479406871,
-0.695123583247846));
#37294=CARTESIAN_POINT('Ctrl Pts',(0.302628938713621,-0.512792550344605,
-0.684748110997126));
#37295=CARTESIAN_POINT('Ctrl Pts',(0.507617355421152,-0.311222115434097,
-0.674372638746409));
#37296=CARTESIAN_POINT('Ctrl Pts',(0.594273793373837,-0.0371010254861046,
-0.66399716649569));
#37297=CARTESIAN_POINT('Ctrl Pts',(0.542385624529068,0.245671060423536,
-0.653621694244972));
#37298=CARTESIAN_POINT('Ctrl Pts',(0.364054758182736,0.471169804196079,
-0.643246221994254));
#37299=CARTESIAN_POINT('Ctrl Pts',(0.100852138510465,0.586826789571409,
-0.632870749743535));
#37300=CARTESIAN_POINT('Ctrl Pts',(-0.185861335713837,0.565678625875551,
-0.622495277492817));
#37301=CARTESIAN_POINT('Ctrl Pts',(-0.429245823844828,0.412655851503898,
-0.612119805242099));
#37302=CARTESIAN_POINT('Ctrl Pts',(-0.552028076495681,0.199139421463527,
-0.603230874546727));
#37303=CARTESIAN_POINT('Ctrl Pts',(-0.572190591549094,0.0530418625337585,
-0.597800434601597));
#37304=CARTESIAN_POINT('Ctrl Pts',(-0.572208961924848,-5.40006758461067E-6,
-0.595828485406705));
#37305=CARTESIAN_POINT('Ctrl Pts',(-0.57227986394681,-1.09618492728416E-5,
-0.722987304066981));
#37306=CARTESIAN_POINT('Ctrl Pts',(-0.572288362754473,-0.010857064175054,
-0.722583999558541));
#37307=CARTESIAN_POINT('Ctrl Pts',(-0.569393706449464,-0.114707216006389,
-0.718722204299863));
#37308=CARTESIAN_POINT('Ctrl Pts',(-0.509318192700196,-0.308427575223672,
-0.711401918290944));
#37309=CARTESIAN_POINT('Ctrl Pts',(-0.305432606070274,-0.511127575150115,
-0.701026446040226));
#37310=CARTESIAN_POINT('Ctrl Pts',(-0.0303432431553614,-0.594654413195259,
-0.690650973789507));
#37311=CARTESIAN_POINT('Ctrl Pts',(0.251820278225985,-0.539559427088026,
-0.680275501538789));
#37312=CARTESIAN_POINT('Ctrl Pts',(0.47527762677182,-0.358674800641695,
-0.669900029288071));
#37313=CARTESIAN_POINT('Ctrl Pts',(0.587935213613219,-0.0941755582271385,
-0.659524557037353));
#37314=CARTESIAN_POINT('Ctrl Pts',(0.563529430095987,0.192279525622204,
-0.649149084786634));
#37315=CARTESIAN_POINT('Ctrl Pts',(0.407749978910367,0.433908628992312,
-0.638773612535916));
#37316=CARTESIAN_POINT('Ctrl Pts',(0.156913157834808,0.574382355007991,
-0.628398140285198));
#37317=CARTESIAN_POINT('Ctrl Pts',(-0.130504285744414,0.580952155897969,
-0.618022668034479));
#37318=CARTESIAN_POINT('Ctrl Pts',(-0.387497714117257,0.452086632150457,
-0.607647195783761));
#37319=CARTESIAN_POINT('Ctrl Pts',(-0.541268381761995,0.235941679265191,
-0.598074004285823));
#37320=CARTESIAN_POINT('Ctrl Pts',(-0.572181309081377,0.0714266571357631,
-0.591959303538124));
#37321=CARTESIAN_POINT('Ctrl Pts',(-0.572249685678755,-1.32408837812507E-5,
-0.589303093540665));
#37322=CARTESIAN_POINT('Origin',(0.,0.,0.895));
#37323=CARTESIAN_POINT('',(-0.692512978718214,1.7491275774939E-5,0.74826868253652));
#37324=CARTESIAN_POINT('',(-0.692497106487793,1.22237887413546E-5,0.72673131746348));
#37325=CARTESIAN_POINT('',(-0.6925,-8.48067908409542E-17,0.895));
#37326=CARTESIAN_POINT('',(0.301885354887797,0.623234692956248,0.7));
#37327=CARTESIAN_POINT('Ctrl Pts',(-0.692512978718214,1.7491275774939E-5,
0.74826868253652));
#37328=CARTESIAN_POINT('Ctrl Pts',(-0.692536236153761,0.0225620266177927,
0.747491425144957));
#37329=CARTESIAN_POINT('Ctrl Pts',(-0.691457063407575,0.0451043386912214,
0.746714167753393));
#37330=CARTESIAN_POINT('Ctrl Pts',(-0.68925900073676,0.0675370076365317,
0.74593691036183));
#37331=CARTESIAN_POINT('Ctrl Pts',(-0.678019345746454,0.182245047040874,
0.741962453656916));
#37332=CARTESIAN_POINT('Ctrl Pts',(-0.637523809648264,0.294086221483862,
0.737987996952002));
#37333=CARTESIAN_POINT('Ctrl Pts',(-0.572718974199324,0.389399622791066,
0.734013540247089));
#37334=CARTESIAN_POINT('Ctrl Pts',(-0.507914138750383,0.484713024098269,
0.730039083542176));
#37335=CARTESIAN_POINT('Ctrl Pts',(-0.418800003950691,0.563498652269687,
0.726064626837263));
#37336=CARTESIAN_POINT('Ctrl Pts',(-0.316262007750742,0.616131421297654,
0.72209017013235));
#37337=CARTESIAN_POINT('Ctrl Pts',(-0.213724011550792,0.668764190325621,
0.718115713427437));
#37338=CARTESIAN_POINT('Ctrl Pts',(-0.0977621539505856,0.695244100210136,
0.714141256722523));
#37339=CARTESIAN_POINT('Ctrl Pts',(0.0174586834402198,0.692339189277836,
0.710166800017609));
#37340=CARTESIAN_POINT('Ctrl Pts',(0.115705001414163,0.689862234504694,
0.706777866678406));
#37341=CARTESIAN_POINT('Ctrl Pts',(0.213412552912613,0.666020739137871,
0.703388933339203));
#37342=CARTESIAN_POINT('Ctrl Pts',(0.301912013981581,0.623256720988311,
0.7));
#37343=CARTESIAN_POINT('',(-0.3018853548878,0.623234692956246,0.7));
#37344=CARTESIAN_POINT('Origin',(0.,0.,0.7));
#37345=CARTESIAN_POINT('Ctrl Pts',(-0.301885354887799,0.623234692956247,
0.7));
#37346=CARTESIAN_POINT('Ctrl Pts',(-0.405642496870894,0.572976320013088,
0.703974456704914));
#37347=CARTESIAN_POINT('Ctrl Pts',(-0.496552660568787,0.496329702965772,
0.707948913409827));
#37348=CARTESIAN_POINT('Ctrl Pts',(-0.563546539109462,0.402559533859148,
0.71192337011474));
#37349=CARTESIAN_POINT('Ctrl Pts',(-0.630540417650137,0.308789364752525,
0.715897826819654));
#37350=CARTESIAN_POINT('Ctrl Pts',(-0.673618011033594,0.197895643586594,
0.719872283524567));
#37351=CARTESIAN_POINT('Ctrl Pts',(-0.687511393683796,0.0834733607376968,
0.72384674022948));
#37352=CARTESIAN_POINT('Ctrl Pts',(-0.690872568830618,0.055791597193332,
0.724808265974147));
#37353=CARTESIAN_POINT('Ctrl Pts',(-0.692525640229921,0.0279033127500774,
0.725769791718813));
#37354=CARTESIAN_POINT('Ctrl Pts',(-0.692497106487793,1.22237887413546E-5,
0.72673131746348));
#37355=CARTESIAN_POINT('Origin',(0.,0.,0.895));
#37356=CARTESIAN_POINT('',(-0.692502505300729,-1.80142461571609E-5,0.89826868253652));
#37357=CARTESIAN_POINT('',(-0.692519446907948,-1.67109334056352E-5,0.87673131746348));
#37358=CARTESIAN_POINT('',(-0.6925,-8.48067908409542E-17,0.895));
#37359=CARTESIAN_POINT('Ctrl Pts',(-0.692502505300729,-1.80142461571609E-5,
0.89826868253652));
#37360=CARTESIAN_POINT('Ctrl Pts',(-0.692409964808609,0.0894315645319258,
0.895184905603917));
#37361=CARTESIAN_POINT('Ctrl Pts',(-0.675000463397104,0.178916114041078,
0.892101128671314));
#37362=CARTESIAN_POINT('Ctrl Pts',(-0.641206247017397,0.261713119701919,
0.889017351738711));
#37363=CARTESIAN_POINT('Ctrl Pts',(-0.597651329520742,0.368424182624908,
0.885042895033797));
#37364=CARTESIAN_POINT('Ctrl Pts',(-0.526880147296139,0.46402672372688,
0.881068438328884));
#37365=CARTESIAN_POINT('Ctrl Pts',(-0.43753750447404,0.536842751989744,
0.877093981623971));
#37366=CARTESIAN_POINT('Ctrl Pts',(-0.348194861651941,0.609658780252608,
0.873119524919057));
#37367=CARTESIAN_POINT('Ctrl Pts',(-0.240280758232347,0.659688295676364,
0.869145068214144));
#37368=CARTESIAN_POINT('Ctrl Pts',(-0.126977060875423,0.680820118935961,
0.865170611509231));
#37369=CARTESIAN_POINT('Ctrl Pts',(-0.0136733635184988,0.701951942195558,
0.861196154804318));
#37370=CARTESIAN_POINT('Ctrl Pts',(0.105019927775755,0.694186073290997,
0.857221698099404));
#37371=CARTESIAN_POINT('Ctrl Pts',(0.214604252685671,0.658471125218892,
0.853247241394491));
#37372=CARTESIAN_POINT('Ctrl Pts',(0.324188577595589,0.622756177146787,
0.849272784689577));
#37373=CARTESIAN_POINT('Ctrl Pts',(0.424663936121169,0.55909214990714,0.845298327984664));
#37374=CARTESIAN_POINT('Ctrl Pts',(0.503757115234358,0.475255696844551,
0.841323871279751));
#37375=CARTESIAN_POINT('Ctrl Pts',(0.582850294347546,0.391419243781962,
0.837349414574837));
#37376=CARTESIAN_POINT('Ctrl Pts',(0.640561294048343,0.287410364896433,
0.833374957869924));
#37377=CARTESIAN_POINT('Ctrl Pts',(0.669840630764095,0.175933900582539,
0.82940050116501));
#37378=CARTESIAN_POINT('Ctrl Pts',(0.699119967479848,0.0644574362686454,
0.825426044460097));
#37379=CARTESIAN_POINT('Ctrl Pts',(0.699967641210555,-0.0544866134736121,
0.821451587755184));
#37380=CARTESIAN_POINT('Ctrl Pts',(0.67228010730006,-0.1663690631073,0.81747713105027));
#37381=CARTESIAN_POINT('Ctrl Pts',(0.644592573389564,-0.278251512740987,
0.813502674345357));
#37382=CARTESIAN_POINT('Ctrl Pts',(0.588369831837864,-0.383072362266105,
0.809528217640443));
#37383=CARTESIAN_POINT('Ctrl Pts',(0.5104795734465,-0.468027579985086,0.80555376093553));
#37384=CARTESIAN_POINT('Ctrl Pts',(0.432589315055136,-0.552982797704068,
0.801579304230617));
#37385=CARTESIAN_POINT('Ctrl Pts',(0.333031539824107,-0.618072383616913,
0.797604847525703));
#37386=CARTESIAN_POINT('Ctrl Pts',(0.223967376371222,-0.65534556996308,
0.79363039082079));
#37387=CARTESIAN_POINT('Ctrl Pts',(0.114903212918336,-0.692618756309248,
0.789655934115876));
#37388=CARTESIAN_POINT('Ctrl Pts',(-0.00366733875640471,-0.702075543088738,
0.785681477410963));
#37389=CARTESIAN_POINT('Ctrl Pts',(-0.117260710663312,-0.682560728047434,
0.78170702070605));
#37390=CARTESIAN_POINT('Ctrl Pts',(-0.23085408257022,-0.66304591300613,
0.777732564001136));
#37391=CARTESIAN_POINT('Ctrl Pts',(-0.339470274709293,-0.614559496144031,
0.773758107296224));
#37392=CARTESIAN_POINT('Ctrl Pts',(-0.429841660219421,-0.54302424791586,
0.76978365059131));
#37393=CARTESIAN_POINT('Ctrl Pts',(-0.52021304572955,-0.471488999687688,
0.765809193886397));
#37394=CARTESIAN_POINT('Ctrl Pts',(-0.592339624610732,-0.376904920093444,
0.761834737181483));
#37395=CARTESIAN_POINT('Ctrl Pts',(-0.637411027110111,-0.270825428113474,
0.757860280476569));
#37396=CARTESIAN_POINT('Ctrl Pts',(-0.673668122814433,-0.185491178906639,
0.754663081163219));
#37397=CARTESIAN_POINT('Ctrl Pts',(-0.6924173107223,-0.0927180345585824,
0.75146588184987));
#37398=CARTESIAN_POINT('Ctrl Pts',(-0.692512978718214,1.7491275774939E-5,
0.74826868253652));
#37399=CARTESIAN_POINT('Ctrl Pts',(-0.692497106487793,1.22237887413546E-5,
0.72673131746348));
#37400=CARTESIAN_POINT('Ctrl Pts',(-0.692407696302423,-0.0873842145414211,
0.729744248423727));
#37401=CARTESIAN_POINT('Ctrl Pts',(-0.675807013310445,-0.17480818975405,
0.732757179383974));
#37402=CARTESIAN_POINT('Ctrl Pts',(-0.643510339446282,-0.255991965181027,
0.735770110344221));
#37403=CARTESIAN_POINT('Ctrl Pts',(-0.600906730641617,-0.36308416371899,
0.739744567049134));
#37404=CARTESIAN_POINT('Ctrl Pts',(-0.530990341115338,-0.459317716263051,
0.743719023754047));
#37405=CARTESIAN_POINT('Ctrl Pts',(-0.44229971099925,-0.532927429012877,
0.74769348045896));
#37406=CARTESIAN_POINT('Ctrl Pts',(-0.353609080883162,-0.606537141762702,
0.751667937163873));
#37407=CARTESIAN_POINT('Ctrl Pts',(-0.246144210177266,-0.657523014718292,
0.755642393868788));
#37408=CARTESIAN_POINT('Ctrl Pts',(-0.133033022371476,-0.679662110949492,
0.759616850573701));
#37409=CARTESIAN_POINT('Ctrl Pts',(-0.0199218345656862,-0.701801207180692,
0.763591307278615));
#37410=CARTESIAN_POINT('Ctrl Pts',(0.0988356703399968,-0.695093526687502,
0.767565763983527));
#37411=CARTESIAN_POINT('Ctrl Pts',(0.208733556028134,-0.660355882111,0.771540220688441));
#37412=CARTESIAN_POINT('Ctrl Pts',(0.318631441716272,-0.625618237534498,
0.775514677393354));
#37413=CARTESIAN_POINT('Ctrl Pts',(0.419669708186863,-0.562850628874684,
0.779489134098267));
#37414=CARTESIAN_POINT('Ctrl Pts',(0.499506147484576,-0.479721487442206,
0.783463590803181));
#37415=CARTESIAN_POINT('Ctrl Pts',(0.579342586782288,-0.396592346009729,
0.787438047508095));
#37416=CARTESIAN_POINT('Ctrl Pts',(0.637977198907121,-0.293101671804589,
0.791412504213008));
#37417=CARTESIAN_POINT('Ctrl Pts',(0.668247797592216,-0.181890362651708,
0.795386960917921));
#37418=CARTESIAN_POINT('Ctrl Pts',(0.698518396277312,-0.0706790534988262,
0.799361417622835));
#37419=CARTESIAN_POINT('Ctrl Pts',(0.700424981522668,0.048252890601796,
0.803335874327748));
#37420=CARTESIAN_POINT('Ctrl Pts',(0.673734601904745,0.160377435949487,
0.807310331032661));
#37421=CARTESIAN_POINT('Ctrl Pts',(0.647044222286821,0.272501981297179,
0.811284787737575));
#37422=CARTESIAN_POINT('Ctrl Pts',(0.591756877805617,0.377819127891939,
0.815259244442488));
#37423=CARTESIAN_POINT('Ctrl Pts',(0.514626028750265,0.463464392651226,
0.819233701147402));
#37424=CARTESIAN_POINT('Ctrl Pts',(0.437495179694913,0.549109657410513,
0.823208157852315));
#37425=CARTESIAN_POINT('Ctrl Pts',(0.338520826065412,0.615083040334327,
0.827182614557228));
#37426=CARTESIAN_POINT('Ctrl Pts',(0.22979281598256,0.653325714460818,0.831157071262141));
#37427=CARTESIAN_POINT('Ctrl Pts',(0.121064805899708,0.691568388587309,
0.835131527967055));
#37428=CARTESIAN_POINT('Ctrl Pts',(0.00258313936350399,0.702080353916477,
0.839105984671969));
#37429=CARTESIAN_POINT('Ctrl Pts',(-0.111179466074118,0.683577599114679,
0.843080441376882));
#37430=CARTESIAN_POINT('Ctrl Pts',(-0.22494207151174,0.665074844312881,
0.847054898081795));
#37431=CARTESIAN_POINT('Ctrl Pts',(-0.33398561585078,0.617557369380116,
0.851029354786708));
#37432=CARTESIAN_POINT('Ctrl Pts',(-0.424990273328466,0.546829483415133,
0.855003811491622));
#37433=CARTESIAN_POINT('Ctrl Pts',(-0.515994930806152,0.476101597450151,
0.858978268196535));
#37434=CARTESIAN_POINT('Ctrl Pts',(-0.588960701422483,0.382163300452951,
0.862952724901448));
#37435=CARTESIAN_POINT('Ctrl Pts',(-0.634974706950498,0.276489304008043,
0.866927181606362));
#37436=CARTESIAN_POINT('Ctrl Pts',(-0.67281028172387,0.189597577278057,
0.870195226892068));
#37437=CARTESIAN_POINT('Ctrl Pts',(-0.692423363006564,0.0947711677510941,
0.873463272177774));
#37438=CARTESIAN_POINT('Ctrl Pts',(-0.692519446907948,-1.67109334056352E-5,
0.87673131746348));
#37439=CARTESIAN_POINT('Origin',(0.,0.,0.895));
#37440=CARTESIAN_POINT('',(-0.692459617039174,1.37475917892233E-5,1.04826868253652));
#37441=CARTESIAN_POINT('',(-0.692449505282264,9.96448218454668E-6,1.02673131746348));
#37442=CARTESIAN_POINT('',(-0.6925,-8.48067908409542E-17,0.895));
#37443=CARTESIAN_POINT('Ctrl Pts',(-0.692459617039174,1.37475917892232E-5,
1.04826868253652));
#37444=CARTESIAN_POINT('Ctrl Pts',(-0.692488936078667,0.0410896088323068,
1.04685284276779));
#37445=CARTESIAN_POINT('Ctrl Pts',(-0.688893820320347,0.0821603968297718,
1.04543700299906));
#37446=CARTESIAN_POINT('Ctrl Pts',(-0.681627147119585,0.122570961233086,
1.04402116323033));
#37447=CARTESIAN_POINT('Ctrl Pts',(-0.661228597323865,0.236008966146766,
1.04004670652542));
#37448=CARTESIAN_POINT('Ctrl Pts',(-0.611898100953193,0.34424439584463,
1.03607224982051));
#37449=CARTESIAN_POINT('Ctrl Pts',(-0.539661450787553,0.434056133192316,
1.03209779311559));
#37450=CARTESIAN_POINT('Ctrl Pts',(-0.467424800621913,0.523867870540003,
1.02812333641068));
#37451=CARTESIAN_POINT('Ctrl Pts',(-0.372281996661304,0.595255915537511,
1.02414887970577));
#37452=CARTESIAN_POINT('Ctrl Pts',(-0.265854872524943,0.6395001133563,1.02017442300085));
#37453=CARTESIAN_POINT('Ctrl Pts',(-0.159427748388581,0.68374431117509,
1.01619996629594));
#37454=CARTESIAN_POINT('Ctrl Pts',(-0.0417163040764662,0.700844661815162,
1.01222550959103));
#37455=CARTESIAN_POINT('Ctrl Pts',(0.0729008341367396,0.688712332262305,
1.00825105288611));
#37456=CARTESIAN_POINT('Ctrl Pts',(0.187517972349945,0.676580002709448,
1.0042765961812));
#37457=CARTESIAN_POINT('Ctrl Pts',(0.299040804464242,0.635214992963663,
1.00030213947629));
#37458=CARTESIAN_POINT('Ctrl Pts',(0.393846652298814,0.56967009988322,0.996327682771372));
#37459=CARTESIAN_POINT('Ctrl Pts',(0.488652500133385,0.504125206802777,
0.992353226066459));
#37460=CARTESIAN_POINT('Ctrl Pts',(0.566741363688231,0.414400430387678,
0.988378769361545));
#37461=CARTESIAN_POINT('Ctrl Pts',(0.618574573279787,0.311455784213055,
0.984404312656632));
#37462=CARTESIAN_POINT('Ctrl Pts',(0.670407782871342,0.208511138038433,
0.980429855951718));
#37463=CARTESIAN_POINT('Ctrl Pts',(0.695985338499608,0.0923466221042891,
0.976455399246806));
#37464=CARTESIAN_POINT('Ctrl Pts',(0.692182904076904,-0.0228480968935343,
0.972480942541892));
#37465=CARTESIAN_POINT('Ctrl Pts',(0.6883804696542,-0.138042815891358,0.968506485836979));
#37466=CARTESIAN_POINT('Ctrl Pts',(0.655198045180526,-0.25226773795286,
0.964532029132065));
#37467=CARTESIAN_POINT('Ctrl Pts',(0.596688912672601,-0.351570120632219,
0.960557572427152));
#37468=CARTESIAN_POINT('Ctrl Pts',(0.538179780164675,-0.450872503311578,
0.956583115722238));
#37469=CARTESIAN_POINT('Ctrl Pts',(0.454343939622498,-0.535252346608794,
0.952608659017325));
#37470=CARTESIAN_POINT('Ctrl Pts',(0.355422062432155,-0.594402528397402,
0.948634202312412));
#37471=CARTESIAN_POINT('Ctrl Pts',(0.256500185241811,-0.653552710186011,
0.944659745607498));
#37472=CARTESIAN_POINT('Ctrl Pts',(0.1424922714033,-0.687473230466012,0.940685288902585));
#37473=CARTESIAN_POINT('Ctrl Pts',(0.0273245554897345,-0.692020647736393,
0.936710832197671));
#37474=CARTESIAN_POINT('Ctrl Pts',(-0.0878431604238312,-0.696568065006773,
0.932736375492758));
#37475=CARTESIAN_POINT('Ctrl Pts',(-0.204170678412452,-0.671742379267533,
0.928761918787845));
#37476=CARTESIAN_POINT('Ctrl Pts',(-0.307448420839844,-0.62057608458131,
0.924787462082931));
#37477=CARTESIAN_POINT('Ctrl Pts',(-0.410726163267236,-0.569409789895086,
0.920813005378018));
#37478=CARTESIAN_POINT('Ctrl Pts',(-0.500954130133399,-0.491902886261879,
0.916838548673105));
#37479=CARTESIAN_POINT('Ctrl Pts',(-0.567110842408464,-0.397522956125345,
0.912864091968191));
#37480=CARTESIAN_POINT('Ctrl Pts',(-0.633267554683529,-0.303143025988812,
0.908889635263278));
#37481=CARTESIAN_POINT('Ctrl Pts',(-0.675353012367496,-0.191890069348953,
0.904915178558364));
#37482=CARTESIAN_POINT('Ctrl Pts',(-0.688226414825127,-0.0773537986570187,
0.900940721853451));
#37483=CARTESIAN_POINT('Ctrl Pts',(-0.691111357352151,-0.0516861044096396,
0.900050042081141));
#37484=CARTESIAN_POINT('Ctrl Pts',(-0.692529233545428,-0.0258535179808784,
0.89915936230883));
#37485=CARTESIAN_POINT('Ctrl Pts',(-0.692502505300729,-1.80142461571609E-5,
0.89826868253652));
#37486=CARTESIAN_POINT('Ctrl Pts',(-0.692519446907948,-1.67109334056352E-5,
0.87673131746348));
#37487=CARTESIAN_POINT('Ctrl Pts',(-0.692540216132119,-0.0205057905058466,
0.877437728882687));
#37488=CARTESIAN_POINT('Ctrl Pts',(-0.691649074693246,-0.0409930697662103,
0.878144140301895));
#37489=CARTESIAN_POINT('Ctrl Pts',(-0.689832948476493,-0.0613980215631428,
0.878850551721102));
#37490=CARTESIAN_POINT('Ctrl Pts',(-0.679614944034773,-0.176201654796807,
0.882825008426015));
#37491=CARTESIAN_POINT('Ctrl Pts',(-0.640116694711632,-0.288399225371522,
0.886799465130928));
#37492=CARTESIAN_POINT('Ctrl Pts',(-0.576162969353729,-0.384285632221807,
0.890773921835842));
#37493=CARTESIAN_POINT('Ctrl Pts',(-0.512209243995827,-0.480172039072091,
0.894748378540755));
#37494=CARTESIAN_POINT('Ctrl Pts',(-0.423800042603163,-0.559747282197946,
0.898722835245669));
#37495=CARTESIAN_POINT('Ctrl Pts',(-0.321734679564143,-0.613291129761764,
0.902697291950582));
#37496=CARTESIAN_POINT('Ctrl Pts',(-0.219669316525123,-0.666834977325583,
0.906671748655496));
#37497=CARTESIAN_POINT('Ctrl Pts',(-0.103947791839747,-0.694347429327364,
0.910646205360409));
#37498=CARTESIAN_POINT('Ctrl Pts',(0.0112943399504365,-0.692467798585378,
0.914620662065322));
#37499=CARTESIAN_POINT('Ctrl Pts',(0.12653647174062,-0.690588167843393,
0.918595118770236));
#37500=CARTESIAN_POINT('Ctrl Pts',(0.24129921063561,-0.659316454357642,
0.922569575475149));
#37501=CARTESIAN_POINT('Ctrl Pts',(0.341564119009619,-0.602472544311455,
0.926544032180063));
#37502=CARTESIAN_POINT('Ctrl Pts',(0.441829027383627,-0.545628634265269,
0.930518488884976));
#37503=CARTESIAN_POINT('Ctrl Pts',(0.527596105236653,-0.463212527658647,
0.934492945589889));
#37504=CARTESIAN_POINT('Ctrl Pts',(0.588388777731319,-0.365291473122074,
0.938467402294802));
#37505=CARTESIAN_POINT('Ctrl Pts',(0.649181450225985,-0.2673704185855,0.942441858999716));
#37506=CARTESIAN_POINT('Ctrl Pts',(0.684999717362292,-0.153944416118975,
0.946416315704629));
#37507=CARTESIAN_POINT('Ctrl Pts',(0.691468325045282,-0.0388686190472216,
0.950390772409543));
#37508=CARTESIAN_POINT('Ctrl Pts',(0.697936932728271,0.0762071780245319,
0.954365229114456));
#37509=CARTESIAN_POINT('Ctrl Pts',(0.675055880957944,0.192932769701512,
0.95833968581937));
#37510=CARTESIAN_POINT('Ctrl Pts',(0.625620123912279,0.297049953101773,
0.962314142524283));
#37511=CARTESIAN_POINT('Ctrl Pts',(0.576184366866613,0.401167136502033,
0.966288599229196));
#37512=CARTESIAN_POINT('Ctrl Pts',(0.500193904545608,0.492675911625573,
0.97026305593411));
#37513=CARTESIAN_POINT('Ctrl Pts',(0.406931083827991,0.560398346806577,
0.974237512639023));
#37514=CARTESIAN_POINT('Ctrl Pts',(0.313668263110376,0.628120781987582,
0.978211969343936));
#37515=CARTESIAN_POINT('Ctrl Pts',(0.203133083996148,0.672056877226051,
0.98218642604885));
#37516=CARTESIAN_POINT('Ctrl Pts',(0.0888275813995918,0.686839773795016,
0.986160882753763));
#37517=CARTESIAN_POINT('Ctrl Pts',(-0.0254779211969667,0.701622670363981,
0.990135339458677));
#37518=CARTESIAN_POINT('Ctrl Pts',(-0.143553747275854,0.68725236826344,
0.99410979616359));
#37519=CARTESIAN_POINT('Ctrl Pts',(-0.250976760793945,0.645484221052659,
0.998084252868503));
#37520=CARTESIAN_POINT('Ctrl Pts',(-0.358399774312035,0.603716073841877,
1.00205870957342));
#37521=CARTESIAN_POINT('Ctrl Pts',(-0.455169975269328,0.534550081520856,
1.00603316627833));
#37522=CARTESIAN_POINT('Ctrl Pts',(-0.529466741106335,0.446434971913998,
1.01000762298324));
#37523=CARTESIAN_POINT('Ctrl Pts',(-0.603763506943343,0.358319862307138,
1.01398207968816));
#37524=CARTESIAN_POINT('Ctrl Pts',(-0.655586837660064,0.251255635414442,
1.01795653639307));
#37525=CARTESIAN_POINT('Ctrl Pts',(-0.678606437090228,0.138320344221461,
1.02193099309798));
#37526=CARTESIAN_POINT('Ctrl Pts',(-0.68787408063104,0.092852827502517,
1.02353110121982));
#37527=CARTESIAN_POINT('Ctrl Pts',(-0.69247306823634,0.0464336986844112,
1.02513120934165));
#37528=CARTESIAN_POINT('Ctrl Pts',(-0.692449505282264,9.96448218454669E-6,
1.02673131746348));
#37529=CARTESIAN_POINT('Origin',(0.,0.,0.895));
#37530=CARTESIAN_POINT('',(-0.692553258028562,-7.52956544752825E-6,1.19826868253652));
#37531=CARTESIAN_POINT('',(-0.692559371888614,-2.09617465497895E-6,1.17673131746348));
#37532=CARTESIAN_POINT('',(-0.6925,-8.48067908409542E-17,0.895));
#37533=CARTESIAN_POINT('Ctrl Pts',(-0.692553258028562,-7.52956544752825E-6,
1.19826868253652));
#37534=CARTESIAN_POINT('Ctrl Pts',(-0.692493376955139,0.10794222829347,
1.19454632322675));
#37535=CARTESIAN_POINT('Ctrl Pts',(-0.666836185272269,0.215919453832076,
1.19082396391698));
#37536=CARTESIAN_POINT('Ctrl Pts',(-0.618163761380453,0.312270351368743,
1.18710160460721));
#37537=CARTESIAN_POINT('Ctrl Pts',(-0.566194989592747,0.415146629253594,
1.1831271479023));
#37538=CARTESIAN_POINT('Ctrl Pts',(-0.48798800092297,0.504768462738863,
1.17915269119739));
#37539=CARTESIAN_POINT('Ctrl Pts',(-0.393095894211433,0.570188412879551,
1.17517823449247));
#37540=CARTESIAN_POINT('Ctrl Pts',(-0.298203787499896,0.635608363020239,
1.17120377778756));
#37541=CARTESIAN_POINT('Ctrl Pts',(-0.186626562746599,0.676826429816346,
1.16722932108265));
#37542=CARTESIAN_POINT('Ctrl Pts',(-0.0719935422733182,0.688807765707478,
1.16325486437773));
#37543=CARTESIAN_POINT('Ctrl Pts',(0.042639478199963,0.70078910159861,1.15928040767282));
#37544=CARTESIAN_POINT('Ctrl Pts',(0.160328294393228,0.683533706584767,
1.15530595096791));
#37545=CARTESIAN_POINT('Ctrl Pts',(0.266697044089859,0.639149352578659,
1.15133149426299));
#37546=CARTESIAN_POINT('Ctrl Pts',(0.373065793786489,0.594764998572552,
1.14735703755808));
#37547=CARTESIAN_POINT('Ctrl Pts',(0.468114476986484,0.523251685574181,
1.14338258085317));
#37548=CARTESIAN_POINT('Ctrl Pts',(0.540232757060147,0.433344870082916,
1.13940812414825));
#37549=CARTESIAN_POINT('Ctrl Pts',(0.61235103713381,0.343438054591652,1.13543366744334));
#37550=CARTESIAN_POINT('Ctrl Pts',(0.661538914081142,0.235137736607494,
1.13145921073843));
#37551=CARTESIAN_POINT('Ctrl Pts',(0.681788016294753,0.121672959464514,
1.12748475403351));
#37552=CARTESIAN_POINT('Ctrl Pts',(0.702037118508365,0.00820818232153232,
1.1235102973286));
#37553=CARTESIAN_POINT('Ctrl Pts',(0.693347445988256,-0.110421053980272,
1.11953584062369));
#37554=CARTESIAN_POINT('Ctrl Pts',(0.656780455029912,-0.219724013523077,
1.11556138391877));
#37555=CARTESIAN_POINT('Ctrl Pts',(0.620213464071568,-0.329026973065883,
1.11158692721386));
#37556=CARTESIAN_POINT('Ctrl Pts',(0.555769154674989,-0.42900365584969,
1.10761247050895));
#37557=CARTESIAN_POINT('Ctrl Pts',(0.471319494139167,-0.507441762838246,
1.10363801380403));
#37558=CARTESIAN_POINT('Ctrl Pts',(0.386869833603345,-0.585879869826803,
1.09966355709912));
#37559=CARTESIAN_POINT('Ctrl Pts',(0.28241482192828,-0.642779401020109,
1.09568910039421));
#37560=CARTESIAN_POINT('Ctrl Pts',(0.170713792619461,-0.671189994887787,
1.09171464368929));
#37561=CARTESIAN_POINT('Ctrl Pts',(0.0590127633106426,-0.699600588755465,
1.08774018698438));
#37562=CARTESIAN_POINT('Ctrl Pts',(-0.0599342836319292,-0.699522245297516,
1.08376573027947));
#37563=CARTESIAN_POINT('Ctrl Pts',(-0.171597791252629,-0.670964534282704,
1.07979127357455));
#37564=CARTESIAN_POINT('Ctrl Pts',(-0.283261298873331,-0.642406823267892,
1.07581681686964));
#37565=CARTESIAN_POINT('Ctrl Pts',(-0.38764126717216,-0.585369744696218,
1.07184236016473));
#37566=CARTESIAN_POINT('Ctrl Pts',(-0.47198752930255,-0.506820461712886,
1.06786790345981));
#37567=CARTESIAN_POINT('Ctrl Pts',(-0.556333791432939,-0.428271178729555,
1.0638934467549));
#37568=CARTESIAN_POINT('Ctrl Pts',(-0.62064634739489,-0.328209691334567,
1.05991899004999));
#37569=CARTESIAN_POINT('Ctrl Pts',(-0.657069323765481,-0.218858657572326,
1.05594453334507));
#37570=CARTESIAN_POINT('Ctrl Pts',(-0.680517168622571,-0.148462266883901,
1.05338591640889));
#37571=CARTESIAN_POINT('Ctrl Pts',(-0.692406633507664,-0.0742159756859151,
1.0508272994727));
#37572=CARTESIAN_POINT('Ctrl Pts',(-0.692459617039174,1.37475917892232E-5,
1.04826868253652));
#37573=CARTESIAN_POINT('Ctrl Pts',(-0.692449505282264,9.96448218454669E-6,
1.02673131746348));
#37574=CARTESIAN_POINT('Ctrl Pts',(-0.692414540978377,-0.0688767101246464,
1.02910566604656));
#37575=CARTESIAN_POINT('Ctrl Pts',(-0.68220135351308,-0.137773525156493,
1.03148001462964));
#37576=CARTESIAN_POINT('Ctrl Pts',(-0.661960581745391,-0.203586350969775,
1.03385436321272));
#37577=CARTESIAN_POINT('Ctrl Pts',(-0.628079258826783,-0.313751399474762,
1.03782881991764));
#37578=CARTESIAN_POINT('Ctrl Pts',(-0.566100744845961,-0.41527514099147,
1.04180327662255));
#37579=CARTESIAN_POINT('Ctrl Pts',(-0.483595806560603,-0.495756300981426,
1.04577773332746));
#37580=CARTESIAN_POINT('Ctrl Pts',(-0.401090868275244,-0.576237460971383,
1.04975219003238));
#37581=CARTESIAN_POINT('Ctrl Pts',(-0.298059505685348,-0.635676039434589,
1.05372664673729));
#37582=CARTESIAN_POINT('Ctrl Pts',(-0.187087151464033,-0.666811526477261,
1.0577011034422));
#37583=CARTESIAN_POINT('Ctrl Pts',(-0.0761147972427186,-0.697947013519933,
1.06167556014712));
#37584=CARTESIAN_POINT('Ctrl Pts',(0.0427985486100149,-0.700779409142074,
1.06565001685203));
#37585=CARTESIAN_POINT('Ctrl Pts',(0.155127445776281,-0.674962732047294,
1.06962447355694));
#37586=CARTESIAN_POINT('Ctrl Pts',(0.267456342942549,-0.649146054952514,
1.07359893026186));
#37587=CARTESIAN_POINT('Ctrl Pts',(0.373200791422349,-0.594680305140813,
1.07757338696677));
#37588=CARTESIAN_POINT('Ctrl Pts',(0.459443951105567,-0.518218554162569,
1.08154784367168));
#37589=CARTESIAN_POINT('Ctrl Pts',(0.545687110788785,-0.441756803184324,
1.0855223003766));
#37590=CARTESIAN_POINT('Ctrl Pts',(0.612428981675421,-0.343299051039535,
1.08949675708151));
#37591=CARTESIAN_POINT('Ctrl Pts',(0.651516945946883,-0.234872057150013,
1.09347121378642));
#37592=CARTESIAN_POINT('Ctrl Pts',(0.690604910218345,-0.12644506326049,
1.09744567049134));
#37593=CARTESIAN_POINT('Ctrl Pts',(0.702038967874634,-0.0080488276262343,
1.10142012719625));
#37594=CARTESIAN_POINT('Ctrl Pts',(0.684422431934264,0.105854375209623,
1.10539458390116));
#37595=CARTESIAN_POINT('Ctrl Pts',(0.666805895993895,0.21975757804548,1.10936904060608));
#37596=CARTESIAN_POINT('Ctrl Pts',(0.620138766456867,0.329167748082939,
1.11334349731099));
#37597=CARTESIAN_POINT('Ctrl Pts',(0.550121501922133,0.420720271925147,
1.1173179540159));
#37598=CARTESIAN_POINT('Ctrl Pts',(0.480104237387399,0.512272795767356,
1.12129241072082));
#37599=CARTESIAN_POINT('Ctrl Pts',(0.38673683785496,0.585967673414315,1.12526686742573));
#37600=CARTESIAN_POINT('Ctrl Pts',(0.281424268678516,0.632802967032073,
1.12924132413064));
#37601=CARTESIAN_POINT('Ctrl Pts',(0.176111699502072,0.679638260649832,
1.13321578083556));
#37602=CARTESIAN_POINT('Ctrl Pts',(0.0588539606816214,0.699613970238391,
1.13719023754047));
#37603=CARTESIAN_POINT('Ctrl Pts',(-0.056025742302142,0.690290033453567,
1.14116469424538));
#37604=CARTESIAN_POINT('Ctrl Pts',(-0.170905445285905,0.680966096668744,
1.1451391509503));
#37605=CARTESIAN_POINT('Ctrl Pts',(-0.283407112432982,0.642342513510539,
1.14911360765521));
#37606=CARTESIAN_POINT('Ctrl Pts',(-0.379788499421787,0.579137211542119,
1.15308806436013));
#37607=CARTESIAN_POINT('Ctrl Pts',(-0.476169886410592,0.515931909573698,
1.15706252106504));
#37608=CARTESIAN_POINT('Ctrl Pts',(-0.556430993241123,0.428144888795061,
1.16103697776995));
#37609=CARTESIAN_POINT('Ctrl Pts',(-0.610767807514664,0.326499463076991,
1.16501143447486));
#37610=CARTESIAN_POINT('Ctrl Pts',(-0.664177296537632,0.226588742846052,
1.16891806213774));
#37611=CARTESIAN_POINT('Ctrl Pts',(-0.692539802909692,0.11328860312279,
1.17282468980061));
#37612=CARTESIAN_POINT('Ctrl Pts',(-0.692559371888614,-2.09617465497895E-6,
1.17673131746348));
#37613=CARTESIAN_POINT('Origin',(0.,0.,0.895));
#37614=CARTESIAN_POINT('',(-0.692440804635195,-1.82486148905814E-6,1.34826868253652));
#37615=CARTESIAN_POINT('',(-0.692444362555486,-6.68421405300118E-6,1.32673131746348));
#37616=CARTESIAN_POINT('',(-0.6925,-8.48067908409542E-17,0.895));
#37617=CARTESIAN_POINT('Ctrl Pts',(-0.692440804635195,-1.82486148905814E-6,
1.34826868253652));
#37618=CARTESIAN_POINT('Ctrl Pts',(-0.692435348926581,0.0596050059372995,
1.34621426039063));
#37619=CARTESIAN_POINT('Ctrl Pts',(-0.684818864295023,0.119213205203163,
1.34415983824473));
#37620=CARTESIAN_POINT('Ctrl Pts',(-0.669608294980035,0.176816117822777,
1.34210541609884));
#37621=CARTESIAN_POINT('Ctrl Pts',(-0.640182137692788,0.288253916885169,
1.33813095939392));
#37622=CARTESIAN_POINT('Ctrl Pts',(-0.582334178987605,0.392186682593103,
1.33415650268901));
#37623=CARTESIAN_POINT('Ctrl Pts',(-0.503130632212173,0.475918874555073,
1.3301820459841));
#37624=CARTESIAN_POINT('Ctrl Pts',(-0.423927085436742,0.559651066517042,
1.32620758927918));
#37625=CARTESIAN_POINT('Ctrl Pts',(-0.323367950591062,0.623182684733047,
1.32223313257427));
#37626=CARTESIAN_POINT('Ctrl Pts',(-0.213736674088512,0.658753248475913,
1.31825867586936));
#37627=CARTESIAN_POINT('Ctrl Pts',(-0.104105397585963,0.69432381221878,
1.31428421916444));
#37628=CARTESIAN_POINT('Ctrl Pts',(0.0145980205734564,0.701933321488508,
1.31030976245953));
#37629=CARTESIAN_POINT('Ctrl Pts',(0.12787378304877,0.680652263521384,1.30633530575461));
#37630=CARTESIAN_POINT('Ctrl Pts',(0.241149545524084,0.659371205554261,
1.3023608490497));
#37631=CARTESIAN_POINT('Ctrl Pts',(0.348997652315293,0.609199580350287,
1.29838639234479));
#37632=CARTESIAN_POINT('Ctrl Pts',(0.438244298351508,0.536265925815152,
1.29441193563988));
#37633=CARTESIAN_POINT('Ctrl Pts',(0.527490944387723,0.463332271280017,
1.29043747893496));
#37634=CARTESIAN_POINT('Ctrl Pts',(0.598136129668944,0.367636587413722,
1.28646302223005));
#37635=CARTESIAN_POINT('Ctrl Pts',(0.641550440774931,0.26086824293018,1.28248856552513));
#37636=CARTESIAN_POINT('Ctrl Pts',(0.684964751880918,0.154099898446638,
1.27851410882022));
#37637=CARTESIAN_POINT('Ctrl Pts',(0.701148188811671,0.0362588933458479,
1.27453965211531));
#37638=CARTESIAN_POINT('Ctrl Pts',(0.688123920912985,-0.0782603200563889,
1.2705651954104));
#37639=CARTESIAN_POINT('Ctrl Pts',(0.675099653014299,-0.192779533458624,
1.26659073870548));
#37640=CARTESIAN_POINT('Ctrl Pts',(0.632867680286175,-0.303976955162307,
1.26261628200057));
#37641=CARTESIAN_POINT('Ctrl Pts',(0.566586700391767,-0.398269656347502,
1.25864182529565));
#37642=CARTESIAN_POINT('Ctrl Pts',(0.500305720497359,-0.492562357532699,
1.25466736859074));
#37643=CARTESIAN_POINT('Ctrl Pts',(0.409975733436666,-0.569950338199408,
1.25069291188583));
#37644=CARTESIAN_POINT('Ctrl Pts',(0.306630680156813,-0.620980542541035,
1.24671845518091));
#37645=CARTESIAN_POINT('Ctrl Pts',(0.203285626876962,-0.672010746882661,
1.242743998476));
#37646=CARTESIAN_POINT('Ctrl Pts',(0.0869255073779509,-0.696683174899206,
1.23876954177109));
#37647=CARTESIAN_POINT('Ctrl Pts',(-0.0282361183815551,-0.691984053173721,
1.23479508506617));
#37648=CARTESIAN_POINT('Ctrl Pts',(-0.143397744141063,-0.687284931448236,
1.23082062836126));
#37649=CARTESIAN_POINT('Ctrl Pts',(-0.257360876161066,-0.65321425998072,
1.22684617165635));
#37650=CARTESIAN_POINT('Ctrl Pts',(-0.35620475003347,-0.593933821466316,
1.22287171495143));
#37651=CARTESIAN_POINT('Ctrl Pts',(-0.455048623905873,-0.534653382951911,
1.21889725824652));
#37652=CARTESIAN_POINT('Ctrl Pts',(-0.538773239630678,-0.450163177390616,
1.21492280154161));
#37653=CARTESIAN_POINT('Ctrl Pts',(-0.597151512097071,-0.350783807819245,
1.21094834483669));
#37654=CARTESIAN_POINT('Ctrl Pts',(-0.655529784563464,-0.251404438247874,
1.20697388813178));
#37655=CARTESIAN_POINT('Ctrl Pts',(-0.688561713771447,-0.137135904666427,
1.20299943142687));
#37656=CARTESIAN_POINT('Ctrl Pts',(-0.692212400922621,-0.0219362767334871,
1.19902497472195));
#37657=CARTESIAN_POINT('Ctrl Pts',(-0.692443961809965,-0.0146292337135863,
1.19877287732681));
#37658=CARTESIAN_POINT('Ctrl Pts',(-0.692557313484087,-0.00731844463249064,
1.19852077993167));
#37659=CARTESIAN_POINT('Ctrl Pts',(-0.692553258028562,-7.52956544752825E-6,
1.19826868253652));
#37660=CARTESIAN_POINT('Ctrl Pts',(-0.692559371888614,-2.09617465497895E-6,
1.17673131746348));
#37661=CARTESIAN_POINT('Ctrl Pts',(-0.692559711656109,-0.0019691122992305,
1.17679914650552));
#37662=CARTESIAN_POINT('Ctrl Pts',(-0.692551507208319,-0.00393612557791079,
1.17686697554756));
#37663=CARTESIAN_POINT('Ctrl Pts',(-0.69253474129393,-0.00590306587988918,
1.17693480458961));
#37664=CARTESIAN_POINT('Ctrl Pts',(-0.691552339083105,-0.121156338461197,
1.18090926129452));
#37665=CARTESIAN_POINT('Ctrl Pts',(-0.661175012944903,-0.236159052966311,
1.18488371799943));
#37666=CARTESIAN_POINT('Ctrl Pts',(-0.605113398003355,-0.336863458455597,
1.18885817470434));
#37667=CARTESIAN_POINT('Ctrl Pts',(-0.549051783061807,-0.437567863944884,
1.19283263140926));
#37668=CARTESIAN_POINT('Ctrl Pts',(-0.467305879316914,-0.523973960418344,
1.19680708811417));
#37669=CARTESIAN_POINT('Ctrl Pts',(-0.369861069297117,-0.585527115942743,
1.20078154481909));
#37670=CARTESIAN_POINT('Ctrl Pts',(-0.272416259277321,-0.647080271467141,
1.204756001524));
#37671=CARTESIAN_POINT('Ctrl Pts',(-0.159272542982623,-0.683780486042478,
1.20873045822891));
#37672=CARTESIAN_POINT('Ctrl Pts',(-0.0442505919835302,-0.6911447744105,
1.21270491493383));
#37673=CARTESIAN_POINT('Ctrl Pts',(0.0707713590155626,-0.698509062778522,
1.21667937163874));
#37674=CARTESIAN_POINT('Ctrl Pts',(0.18767154471905,-0.67653742493923,1.22065382834365));
#37675=CARTESIAN_POINT('Ctrl Pts',(0.292170435286043,-0.627913728812006,
1.22462828504857));
#37676=CARTESIAN_POINT('Ctrl Pts',(0.396669325853035,-0.579290032684783,
1.22860274175348));
#37677=CARTESIAN_POINT('Ctrl Pts',(0.488766921283533,-0.504014278269628,
1.23257719845839));
#37678=CARTESIAN_POINT('Ctrl Pts',(0.55721336466491,-0.411281509825865,
1.23655165516331));
#37679=CARTESIAN_POINT('Ctrl Pts',(0.625659808046288,-0.3185487413821,1.24052611186822));
#37680=CARTESIAN_POINT('Ctrl Pts',(0.670455099378544,-0.208358958909726,
1.24450056857313));
#37681=CARTESIAN_POINT('Ctrl Pts',(0.686127427856067,-0.0941720066126366,
1.24847502527805));
#37682=CARTESIAN_POINT('Ctrl Pts',(0.70179975633359,0.0200149456844525,
1.25244948198296));
#37683=CARTESIAN_POINT('Ctrl Pts',(0.688349121956381,0.138199067806256,
1.25642393868787));
#37684=CARTESIAN_POINT('Ctrl Pts',(0.647418539522168,0.245943995187554,
1.26039839539279));
#37685=CARTESIAN_POINT('Ctrl Pts',(0.606487957087956,0.353688922568853,
1.2643728520977));
#37686=CARTESIAN_POINT('Ctrl Pts',(0.538077426596741,0.450994655209645,
1.26834730880261));
#37687=CARTESIAN_POINT('Ctrl Pts',(0.450543395095222,0.525975154567118,
1.27232176550753));
#37688=CARTESIAN_POINT('Ctrl Pts',(0.363009363593702,0.600955653924592,
1.27629622221244));
#37689=CARTESIAN_POINT('Ctrl Pts',(0.256351831081878,0.653610919998746,
1.28027067891735));
#37690=CARTESIAN_POINT('Ctrl Pts',(0.143599172229069,0.677509034493976,
1.28424513562227));
#37691=CARTESIAN_POINT('Ctrl Pts',(0.0308465133762598,0.701407148989206,
1.28821959232718));
#37692=CARTESIAN_POINT('Ctrl Pts',(-0.0880012718175337,0.696548111905513,
1.29219404903209));
#37693=CARTESIAN_POINT('Ctrl Pts',(-0.198426751365481,0.663525461778502,
1.29616850573701));
#37694=CARTESIAN_POINT('Ctrl Pts',(-0.308852230913428,0.630502811651492,
1.30014296244192));
#37695=CARTESIAN_POINT('Ctrl Pts',(-0.410855404815529,0.569316548481164,
1.30411741914683));
#37696=CARTESIAN_POINT('Ctrl Pts',(-0.491976435161048,0.487440664421897,
1.30809187585175));
#37697=CARTESIAN_POINT('Ctrl Pts',(-0.573097465506566,0.40556478036263,
1.31206633255666));
#37698=CARTESIAN_POINT('Ctrl Pts',(-0.633336352295502,0.302999275414424,
1.31604078926157));
#37699=CARTESIAN_POINT('Ctrl Pts',(-0.665334826793653,0.192272677053432,
1.32001524596649));
#37700=CARTESIAN_POINT('Ctrl Pts',(-0.683358593602554,0.129903754168789,
1.32225393646548));
#37701=CARTESIAN_POINT('Ctrl Pts',(-0.692422451300573,0.0649455399355973,
1.32449262696448));
#37702=CARTESIAN_POINT('Ctrl Pts',(-0.692444362555486,-6.68421405300118E-6,
1.32673131746348));
#37703=CARTESIAN_POINT('Origin',(0.,0.,0.895));
#37704=CARTESIAN_POINT('',(-0.692545368475526,1.10096728344264E-5,1.49826868253652));
#37705=CARTESIAN_POINT('',(-0.692531307667519,1.47955152054312E-5,1.47673131746348));
#37706=CARTESIAN_POINT('',(-0.6925,-8.48067908409542E-17,0.895));
#37707=CARTESIAN_POINT('Ctrl Pts',(-0.692545368475526,1.10096728344264E-5,
1.49826868253652));
#37708=CARTESIAN_POINT('Ctrl Pts',(-0.692553862205703,0.0112195835652045,
1.4978821975545));
#37709=CARTESIAN_POINT('Ctrl Pts',(-0.692287383186695,0.0224277534934861,
1.49749571257248));
#37710=CARTESIAN_POINT('Ctrl Pts',(-0.691743262005351,0.0336224285249397,
1.49710922759046));
#37711=CARTESIAN_POINT('Ctrl Pts',(-0.686147737785575,0.148743981257509,
1.49313477088554));
#37712=CARTESIAN_POINT('Ctrl Pts',(-0.651190884302411,0.262438416055945,
1.48916031418063));
#37713=CARTESIAN_POINT('Ctrl Pts',(-0.591142732692494,0.360817790316279,
1.48518585747572));
#37714=CARTESIAN_POINT('Ctrl Pts',(-0.531094581082575,0.459197164576613,
1.4812114007708));
#37715=CARTESIAN_POINT('Ctrl Pts',(-0.445955131345907,0.542261478298842,
1.47723694406589));
#37716=CARTESIAN_POINT('Ctrl Pts',(-0.346124292649832,0.599864303212682,
1.47326248736098));
#37717=CARTESIAN_POINT('Ctrl Pts',(-0.246293453953757,0.657467128126522,
1.46928803065606));
#37718=CARTESIAN_POINT('Ctrl Pts',(-0.131771226298275,0.68960846423197,
1.46531357395115));
#37719=CARTESIAN_POINT('Ctrl Pts',(-0.0165466684475456,0.692362200000473,
1.46133911724624));
#37720=CARTESIAN_POINT('Ctrl Pts',(0.0986778894031835,0.695115935768976,
1.45736466054132));
#37721=CARTESIAN_POINT('Ctrl Pts',(0.214604777449164,0.668482071200535,
1.45339020383641));
#37722=CARTESIAN_POINT('Ctrl Pts',(0.31707335559214,0.61571397207006,1.4494157471315));
#37723=CARTESIAN_POINT('Ctrl Pts',(0.419541933735116,0.562945872939585,
1.44544129042658));
#37724=CARTESIAN_POINT('Ctrl Pts',(0.508552201975089,0.484043539247076,
1.44146683372167));
#37725=CARTESIAN_POINT('Ctrl Pts',(0.573231424962209,0.388645007254125,
1.43749237701676));
#37726=CARTESIAN_POINT('Ctrl Pts',(0.63791064794933,0.293246475261173,1.43351792031184));
#37727=CARTESIAN_POINT('Ctrl Pts',(0.678258825683598,0.181351744967778,
1.42954346360693));
#37728=CARTESIAN_POINT('Ctrl Pts',(0.689347368834701,0.066628922463654,
1.42556900690202));
#37729=CARTESIAN_POINT('Ctrl Pts',(0.700435911985803,-0.0480939000404694,
1.4215945501971));
#37730=CARTESIAN_POINT('Ctrl Pts',(0.68226482055374,-0.16564481475532,1.41762009349219));
#37731=CARTESIAN_POINT('Ctrl Pts',(0.637053720117189,-0.271664804332269,
1.41364563678728));
#37732=CARTESIAN_POINT('Ctrl Pts',(0.591842619680638,-0.377684793909216,
1.40967118008236));
#37733=CARTESIAN_POINT('Ctrl Pts',(0.5195915102396,-0.47217385834826,1.40569672337745));
#37734=CARTESIAN_POINT('Ctrl Pts',(0.429125971215483,-0.543590019275841,
1.40172226667254));
#37735=CARTESIAN_POINT('Ctrl Pts',(0.338660432191365,-0.615006180203423,
1.39774780996762));
#37736=CARTESIAN_POINT('Ctrl Pts',(0.229980463584167,-0.663349437619542,
1.39377335326271));
#37737=CARTESIAN_POINT('Ctrl Pts',(0.116361483610661,-0.682714591436233,
1.3897988965578));
#37738=CARTESIAN_POINT('Ctrl Pts',(0.00274250363715367,-0.702079745252923,
1.38582443985288));
#37739=CARTESIAN_POINT('Ctrl Pts',(-0.115815487702663,-0.692466795470184,
1.38184998314797));
#37740=CARTESIAN_POINT('Ctrl Pts',(-0.22483045716799,-0.655049978060916,
1.37787552644306));
#37741=CARTESIAN_POINT('Ctrl Pts',(-0.333845426633318,-0.617633160651648,
1.37390106973814));
#37742=CARTESIAN_POINT('Ctrl Pts',(-0.433317374224156,-0.552412475615852,
1.36992661303323));
#37743=CARTESIAN_POINT('Ctrl Pts',(-0.511095655051393,-0.467354725680162,
1.36595215632832));
#37744=CARTESIAN_POINT('Ctrl Pts',(-0.58887393587863,-0.382296975744473,
1.3619776996234));
#37745=CARTESIAN_POINT('Ctrl Pts',(-0.644958549942266,-0.277402160908889,
1.35800324291849));
#37746=CARTESIAN_POINT('Ctrl Pts',(-0.672498679039428,-0.165483337282674,
1.35402878621358));
#37747=CARTESIAN_POINT('Ctrl Pts',(-0.685803138881955,-0.111416070956344,
1.35210875165456));
#37748=CARTESIAN_POINT('Ctrl Pts',(-0.692445903465104,-0.0557095455536165,
1.35018871709554));
#37749=CARTESIAN_POINT('Ctrl Pts',(-0.692440804635195,-1.82486148905814E-6,
1.34826868253652));
#37750=CARTESIAN_POINT('Ctrl Pts',(-0.692444362555486,-6.68421405300118E-6,
1.32673131746348));
#37751=CARTESIAN_POINT('Ctrl Pts',(-0.692461351422783,-0.0503673194731426,
1.3284670836694));
#37752=CARTESIAN_POINT('Ctrl Pts',(-0.687042630329724,-0.10072435369821,
1.33020284987531));
#37753=CARTESIAN_POINT('Ctrl Pts',(-0.676149960582673,-0.14986809163355,
1.33193861608123));
#37754=CARTESIAN_POINT('Ctrl Pts',(-0.651208557666179,-0.262394570185764,
1.33591307278614));
#37755=CARTESIAN_POINT('Ctrl Pts',(-0.597567689625827,-0.368559835516417,
1.33988752949105));
#37756=CARTESIAN_POINT('Ctrl Pts',(-0.521779667488874,-0.455395644117324,
1.34386198619597));
#37757=CARTESIAN_POINT('Ctrl Pts',(-0.445991645351922,-0.54223145271823,
1.34783644290088));
#37758=CARTESIAN_POINT('Ctrl Pts',(-0.34805646911837,-0.609737804589392,
1.35181089960579));
#37759=CARTESIAN_POINT('Ctrl Pts',(-0.239937064792858,-0.64966869943412,
1.35578535631071));
#37760=CARTESIAN_POINT('Ctrl Pts',(-0.131817660467342,-0.68959959427885,
1.35975981301562));
#37761=CARTESIAN_POINT('Ctrl Pts',(-0.0135140280498643,-0.701955032097146,
1.36373426972053));
#37762=CARTESIAN_POINT('Ctrl Pts',(0.100522869535734,-0.685225777963829,
1.36770872642545));
#37763=CARTESIAN_POINT('Ctrl Pts',(0.214559767121331,-0.668496523830512,
1.37168318313036));
#37764=CARTESIAN_POINT('Ctrl Pts',(0.32432992987505,-0.622682577745584,
1.37565763983527));
#37765=CARTESIAN_POINT('Ctrl Pts',(0.416424770759598,-0.553380180692849,
1.37963209654019));
#37766=CARTESIAN_POINT('Ctrl Pts',(0.508519611644146,-0.484077783640114,
1.3836065532451));
#37767=CARTESIAN_POINT('Ctrl Pts',(0.582939130659523,-0.391286935619573,
1.38758100995001));
#37768=CARTESIAN_POINT('Ctrl Pts',(0.630592873961455,-0.286342175368675,
1.39155546665493));
#37769=CARTESIAN_POINT('Ctrl Pts',(0.678246617263387,-0.181397415117777,
1.39552992335984));
#37770=CARTESIAN_POINT('Ctrl Pts',(0.699134584851872,-0.0642987426365235,
1.39950438006475));
#37771=CARTESIAN_POINT('Ctrl Pts',(0.690705280724573,0.0506500667819962,
1.40347883676967));
#37772=CARTESIAN_POINT('Ctrl Pts',(0.682275976597274,0.165598876200516,
1.40745329347458));
#37773=CARTESIAN_POINT('Ctrl Pts',(0.64452940075419,0.278397822556301,1.41142775017949));
#37774=CARTESIAN_POINT('Ctrl Pts',(0.582076353023386,0.375268348434599,
1.41540220688441));
#37775=CARTESIAN_POINT('Ctrl Pts',(0.519623305292582,0.472138874312898,
1.41937666358932));
#37776=CARTESIAN_POINT('Ctrl Pts',(0.432463785674058,0.553080979713709,
1.42335112029423));
#37777=CARTESIAN_POINT('Ctrl Pts',(0.331244457847782,0.608207467260103,
1.42732557699915));
#37778=CARTESIAN_POINT('Ctrl Pts',(0.230025130021506,0.663333954806497,
1.43130003370406));
#37779=CARTESIAN_POINT('Ctrl Pts',(0.114745993987475,0.692644824498473,
1.43527449040897));
#37780=CARTESIAN_POINT('Ctrl Pts',(-0.00051143401784693,0.692559710437379,
1.43924894711389));
#37781=CARTESIAN_POINT('Ctrl Pts',(-0.11576886202317,0.692474596376285,
1.4432234038188));
#37782=CARTESIAN_POINT('Ctrl Pts',(-0.231004581999785,0.662993498562121,
1.44719786052371));
#37783=CARTESIAN_POINT('Ctrl Pts',(-0.332142381046561,0.607717576509441,
1.45117231722863));
#37784=CARTESIAN_POINT('Ctrl Pts',(-0.433280180093337,0.552441654456761,
1.45514677393354));
#37785=CARTESIAN_POINT('Ctrl Pts',(-0.520320058210273,0.471370908165566,
1.45912123063845));
#37786=CARTESIAN_POINT('Ctrl Pts',(-0.582629966103052,0.374408248686699,
1.46309568734337));
#37787=CARTESIAN_POINT('Ctrl Pts',(-0.64493987399583,0.277445589207832,
1.46707014404828));
#37788=CARTESIAN_POINT('Ctrl Pts',(-0.68251981166445,0.164591016541294,
1.47104460075319));
#37789=CARTESIAN_POINT('Ctrl Pts',(-0.6907793343792,0.0496298829382655,
1.47501905745811));
#37790=CARTESIAN_POINT('Ctrl Pts',(-0.691965446214347,0.0331208465377808,
1.47558981079323));
#37791=CARTESIAN_POINT('Ctrl Pts',(-0.692546897704824,0.0165683675781126,
1.47616056412836));
#37792=CARTESIAN_POINT('Ctrl Pts',(-0.692531307667519,1.47955152054312E-5,
1.47673131746348));
#37793=CARTESIAN_POINT('Origin',(0.,0.,0.895));
#37794=CARTESIAN_POINT('',(-0.692468966846601,-1.59520066716212E-5,1.64826868253652));
#37795=CARTESIAN_POINT('',(-0.692483926679543,-1.76726015421153E-5,1.62673131746348));
#37796=CARTESIAN_POINT('',(-0.6925,-8.48067908409542E-17,0.895));
#37797=CARTESIAN_POINT('Ctrl Pts',(-0.692468966846601,-1.59520066716212E-5,
1.64826868253652));
#37798=CARTESIAN_POINT('Ctrl Pts',(-0.692403402184756,0.078109577227228,
1.64557567801346));
#37799=CARTESIAN_POINT('Ctrl Pts',(-0.679206900677884,0.156256752068032,
1.6428826734904));
#37800=CARTESIAN_POINT('Ctrl Pts',(-0.653279802282823,0.229923313136639,
1.64018966896734));
#37801=CARTESIAN_POINT('Ctrl Pts',(-0.61501542909934,0.33864372376346,1.63621521226242));
#37802=CARTESIAN_POINT('Ctrl Pts',(-0.549022315525714,0.437604829530587,
1.63224075555751));
#37803=CARTESIAN_POINT('Ctrl Pts',(-0.463361629978389,0.514718550810581,
1.6282662988526));
#37804=CARTESIAN_POINT('Ctrl Pts',(-0.377700944431063,0.591832272090574,
1.62429184214769));
#37805=CARTESIAN_POINT('Ctrl Pts',(-0.272372686910038,0.647098608883435,
1.62031738544277));
#37806=CARTESIAN_POINT('Ctrl Pts',(-0.160242852952848,0.673766613758384,
1.61634292873786));
#37807=CARTESIAN_POINT('Ctrl Pts',(-0.0481130189956584,0.700434618633334,
1.61236847203294));
#37808=CARTESIAN_POINT('Ctrl Pts',(0.0708183913976963,0.698504291590372,
1.60839401532803));
#37809=CARTESIAN_POINT('Ctrl Pts',(0.182023728166554,0.668211466628036,
1.60441955862312));
#37810=CARTESIAN_POINT('Ctrl Pts',(0.293229064935411,0.6379186416657,1.6004451019182));
#37811=CARTESIAN_POINT('Ctrl Pts',(0.396708328079772,0.579263318783989,
1.59647064521329));
#37812=CARTESIAN_POINT('Ctrl Pts',(0.479821374788218,0.499410311096158,
1.59249618850838));
#37813=CARTESIAN_POINT('Ctrl Pts',(0.562934421496663,0.419557303408327,
1.58852173180346));
#37814=CARTESIAN_POINT('Ctrl Pts',(0.625681251769195,0.318506610914376,
1.58454727509855));
#37815=CARTESIAN_POINT('Ctrl Pts',(0.660397247090718,0.208601735049309,
1.58057281839364));
#37816=CARTESIAN_POINT('Ctrl Pts',(0.69511324241224,0.0986968591842446,
1.57659836168873));
#37817=CARTESIAN_POINT('Ctrl Pts',(0.701798402782755,-0.0200622000519314,
1.57262390498381));
#37818=CARTESIAN_POINT('Ctrl Pts',(0.679636126415314,-0.133168853970496,
1.5686494482789));
#37819=CARTESIAN_POINT('Ctrl Pts',(0.657473850047873,-0.246275507889063,
1.56467499157399));
#37820=CARTESIAN_POINT('Ctrl Pts',(0.606464136942474,-0.353729756490014,
1.56070053486907));
#37821=CARTESIAN_POINT('Ctrl Pts',(0.532837898476493,-0.442405902401399,
1.55672607816416));
#37822=CARTESIAN_POINT('Ctrl Pts',(0.459211660010513,-0.531082048312783,
1.55275162145925));
#37823=CARTESIAN_POINT('Ctrl Pts',(0.36296889618395,-0.600980091534601,
1.54877716475433));
#37824=CARTESIAN_POINT('Ctrl Pts',(0.255865802433896,-0.643561884485609,
1.54480270804942));
#37825=CARTESIAN_POINT('Ctrl Pts',(0.148762708683842,-0.686143677436617,
1.5408282513445));
#37826=CARTESIAN_POINT('Ctrl Pts',(0.0307992850102965,-0.701409220116816,
1.53685379463959));
#37827=CARTESIAN_POINT('Ctrl Pts',(-0.0836150627124207,-0.687493803335081,
1.53287933793468));
#37828=CARTESIAN_POINT('Ctrl Pts',(-0.198029410435138,-0.673578386553346,
1.52890488122976));
#37829=CARTESIAN_POINT('Ctrl Pts',(-0.308894682207027,-0.630482010309677,
1.52493042452485));
#37830=CARTESIAN_POINT('Ctrl Pts',(-0.402668521786135,-0.563468960767016,
1.52095596781994));
#37831=CARTESIAN_POINT('Ctrl Pts',(-0.496442361365244,-0.496455911224355,
1.51698151111502));
#37832=CARTESIAN_POINT('Ctrl Pts',(-0.573124768751571,-0.4055261883827,
1.51300705441011));
#37833=CARTESIAN_POINT('Ctrl Pts',(-0.623348874966542,-0.301786991628521,
1.5090325977052));
#37834=CARTESIAN_POINT('Ctrl Pts',(-0.668689077737925,-0.208135624373867,
1.50544462598231));
#37835=CARTESIAN_POINT('Ctrl Pts',(-0.692466516087684,-0.104044899484275,
1.50185665425941));
#37836=CARTESIAN_POINT('Ctrl Pts',(-0.692545368475526,1.10096728344264E-5,
1.49826868253652));
#37837=CARTESIAN_POINT('Ctrl Pts',(-0.692531307667519,1.47955152054312E-5,
1.47673131746348));
#37838=CARTESIAN_POINT('Ctrl Pts',(-0.692438336046953,-0.0987028913474132,
1.48013502083327));
#37839=CARTESIAN_POINT('Ctrl Pts',(-0.671112380384256,-0.197459452965884,
1.48353872420306));
#37840=CARTESIAN_POINT('Ctrl Pts',(-0.630169276665042,-0.287273209389724,
1.48694242757285));
#37841=CARTESIAN_POINT('Ctrl Pts',(-0.582360588475253,-0.392147473575174,
1.49091688427776));
#37842=CARTESIAN_POINT('Ctrl Pts',(-0.507804104334794,-0.484828307406556,
1.49489134098267));
#37843=CARTESIAN_POINT('Ctrl Pts',(-0.415607008579433,-0.553994610538978,
1.49886579768759));
#37844=CARTESIAN_POINT('Ctrl Pts',(-0.323409912824072,-0.623160913671399,
1.5028402543925));
#37845=CARTESIAN_POINT('Ctrl Pts',(-0.213572205453808,-0.668812686104861,
1.50681471109742));
#37846=CARTESIAN_POINT('Ctrl Pts',(-0.0995107241808008,-0.685373496611229,
1.51078916780233));
#37847=CARTESIAN_POINT('Ctrl Pts',(0.0145507570922064,-0.701934307117598,
1.51476362450724));
#37848=CARTESIAN_POINT('Ctrl Pts',(0.132836012267957,-0.689404155696873,
1.51873808121216));
#37849=CARTESIAN_POINT('Ctrl Pts',(0.240896323230717,-0.649313618787479,
1.52271253791707));
#37850=CARTESIAN_POINT('Ctrl Pts',(0.348956634193476,-0.609223081878085,
1.52668699462198));
#37851=CARTESIAN_POINT('Ctrl Pts',(0.446792000943244,-0.54157215948002,
1.5306614513269));
#37852=CARTESIAN_POINT('Ctrl Pts',(0.522451689348894,-0.454624511413833,
1.53463590803181));
#37853=CARTESIAN_POINT('Ctrl Pts',(0.598111377754543,-0.367676863347648,
1.53861036473672));
#37854=CARTESIAN_POINT('Ctrl Pts',(0.651595387816075,-0.26143248961334,
1.54258482144163));
#37855=CARTESIAN_POINT('Ctrl Pts',(0.676370568943166,-0.148869296885099,
1.54655927814655));
#37856=CARTESIAN_POINT('Ctrl Pts',(0.701145750070258,-0.0363061041568547,
1.55053373485146));
#37857=CARTESIAN_POINT('Ctrl Pts',(0.697212102262908,0.0825759075653193,
1.55450819155638));
#37858=CARTESIAN_POINT('Ctrl Pts',(0.665050126386205,0.193255125390099,
1.55848264826129));
#37859=CARTESIAN_POINT('Ctrl Pts',(0.632888150509503,0.303934343214878,
1.5624571049662));
#37860=CARTESIAN_POINT('Ctrl Pts',(0.572497846563448,0.406410767142259,
1.56643156167112));
#37861=CARTESIAN_POINT('Ctrl Pts',(0.491255979126122,0.488166751240568,
1.57040601837603));
#37862=CARTESIAN_POINT('Ctrl Pts',(0.410014111688796,0.569922735338878,
1.57438047508094));
#37863=CARTESIAN_POINT('Ctrl Pts',(0.307920680760198,0.630958279608118,
1.57835493178586));
#37864=CARTESIAN_POINT('Ctrl Pts',(0.197446549249608,0.663817802097849,
1.58232938849077));
#37865=CARTESIAN_POINT('Ctrl Pts',(0.0869724177390183,0.696677324587579,
1.58630384519568));
#37866=CARTESIAN_POINT('Ctrl Pts',(-0.0318824143535636,0.701360825297801,
1.5902783019006));
#37867=CARTESIAN_POINT('Ctrl Pts',(-0.14459965419217,0.67729620838021,1.59425275860551));
#37868=CARTESIAN_POINT('Ctrl Pts',(-0.257316894030777,0.653231591462618,
1.59822721531042));
#37869=CARTESIAN_POINT('Ctrl Pts',(-0.363896541615409,0.600418856917212,
1.60220167201534));
#37870=CARTESIAN_POINT('Ctrl Pts',(-0.451319736154936,0.52530915672931,
1.60617612872025));
#37871=CARTESIAN_POINT('Ctrl Pts',(-0.538742930694463,0.450199456541409,
1.61015058542516));
#37872=CARTESIAN_POINT('Ctrl Pts',(-0.607009672188885,0.35279279071101,
1.61412504213008));
#37873=CARTESIAN_POINT('Ctrl Pts',(-0.647781077390964,0.244987529539448,
1.61809949883499));
#37874=CARTESIAN_POINT('Ctrl Pts',(-0.677297176576543,0.16694286157434,
1.62097677171115));
#37875=CARTESIAN_POINT('Ctrl Pts',(-0.69240322209232,0.0834483851266751,
1.62385404458732));
#37876=CARTESIAN_POINT('Ctrl Pts',(-0.692483926679543,-1.76726015421153E-5,
1.62673131746348));
#37877=CARTESIAN_POINT('Origin',(0.,0.,0.422718733092612));
#37878=CARTESIAN_POINT('',(-0.606822805098715,-1.39790256400196E-5,1.69771873309261));
#37879=CARTESIAN_POINT('',(-0.606828099052645,1.21067951662501E-5,1.72728126690739));
#37880=CARTESIAN_POINT('',(-0.60685,-1.25452023855349E-14,0.422718733092612));
#37881=CARTESIAN_POINT('',(0.298621660385098,-0.528323265936631,1.7475));
#37882=CARTESIAN_POINT('Ctrl Pts',(-0.606822805098715,-1.39790256400533E-5,
1.69771873309261));
#37883=CARTESIAN_POINT('Ctrl Pts',(-0.606850144986406,-0.0325916380113017,
1.69900018527446));
#37884=CARTESIAN_POINT('Ctrl Pts',(-0.59627583269252,-0.166192123249729,
1.70425609416123));
#37885=CARTESIAN_POINT('Ctrl Pts',(-0.499613590710631,-0.388133987750645,
1.71348645975291));
#37886=CARTESIAN_POINT('Ctrl Pts',(-0.252692420892918,-0.580008494847657,
1.72540982986765));
#37887=CARTESIAN_POINT('Ctrl Pts',(0.0408047583705589,-0.62771684740776,
1.73674767661668));
#37888=CARTESIAN_POINT('Ctrl Pts',(0.223596410438565,-0.57063337113422,
1.7441110666608));
#37889=CARTESIAN_POINT('Ctrl Pts',(0.298621660385098,-0.528323265936631,
1.7475));
#37890=CARTESIAN_POINT('',(-0.401912945313201,-0.454678905261359,1.7475));
#37891=CARTESIAN_POINT('Origin',(0.,0.,1.7475));
#37892=CARTESIAN_POINT('Ctrl Pts',(-0.606828099052645,1.21067951662536E-5,
1.72728126690739));
#37893=CARTESIAN_POINT('Ctrl Pts',(-0.606765611668105,-0.0702881660046895,
1.73004638790001));
#37894=CARTESIAN_POINT('Ctrl Pts',(-0.577018035169713,-0.241685874256128,
1.73678596559755));
#37895=CARTESIAN_POINT('Ctrl Pts',(-0.477608641113037,-0.38776777370368,
1.74352554329509));
#37896=CARTESIAN_POINT('Ctrl Pts',(-0.401912945313201,-0.454678905261359,
1.7475));
#37897=CARTESIAN_POINT('Origin',(0.,0.,0.422718733092612));
#37898=CARTESIAN_POINT('',(-0.60688975719765,9.647971041945E-6,1.54771873309261));
#37899=CARTESIAN_POINT('',(-0.606835914664954,-1.54868133572239E-5,1.57728126690739));
#37900=CARTESIAN_POINT('',(-0.60685,-1.25452023855349E-14,0.422718733092612));
#37901=CARTESIAN_POINT('Ctrl Pts',(-0.60688975719765,9.64797104193935E-6,
1.54771873309261));
#37902=CARTESIAN_POINT('Ctrl Pts',(-0.60682065745532,-0.0911763859235254,
1.5513067048155));
#37903=CARTESIAN_POINT('Ctrl Pts',(-0.562903026131426,-0.28343503097576,
1.55886913324331));
#37904=CARTESIAN_POINT('Ctrl Pts',(-0.367843073028309,-0.514736421708243,
1.57040601837603));
#37905=CARTESIAN_POINT('Ctrl Pts',(-0.0763834766033089,-0.628034772279233,
1.58232938849077));
#37906=CARTESIAN_POINT('Ctrl Pts',(0.233736828044883,-0.5879023770064,1.59425275860551));
#37907=CARTESIAN_POINT('Ctrl Pts',(0.486754537336504,-0.404143701789823,
1.60617612872025));
#37908=CARTESIAN_POINT('Ctrl Pts',(0.620856679132942,-0.121651525197101,
1.61809949883499));
#37909=CARTESIAN_POINT('Ctrl Pts',(0.603281706262845,0.190560468004963,
1.63002286894973));
#37910=CARTESIAN_POINT('Ctrl Pts',(0.43832323427345,0.456217996120286,1.64194623906447));
#37911=CARTESIAN_POINT('Ctrl Pts',(0.166281107894437,0.610420087199418,
1.65386960917921));
#37912=CARTESIAN_POINT('Ctrl Pts',(-0.146383988411153,0.615494826402396,
1.66579297929395));
#37913=CARTESIAN_POINT('Ctrl Pts',(-0.423287034230507,0.470202220700963,
1.67771634940869));
#37914=CARTESIAN_POINT('Ctrl Pts',(-0.578133869070706,0.23799899265915,
1.68835826734158));
#37915=CARTESIAN_POINT('Ctrl Pts',(-0.606765349625733,0.0684488042459758,
1.69502572856955));
#37916=CARTESIAN_POINT('Ctrl Pts',(-0.606822805098715,-1.39790256400533E-5,
1.69771873309261));
#37917=CARTESIAN_POINT('Ctrl Pts',(-0.606835914664954,-1.54868133571684E-5,
1.57728126690739));
#37918=CARTESIAN_POINT('Ctrl Pts',(-0.606862883249031,-0.0279068554810485,
1.57837845073614));
#37919=CARTESIAN_POINT('Ctrl Pts',(-0.598137372064807,-0.156815636589154,
1.5834500912698));
#37920=CARTESIAN_POINT('Ctrl Pts',(-0.508466394890466,-0.376462544933448,
1.59249618850838));
#37921=CARTESIAN_POINT('Ctrl Pts',(-0.266054119846729,-0.574001132528779,
1.60441955862312));
#37922=CARTESIAN_POINT('Ctrl Pts',(0.041355953716283,-0.631309625261172,
1.61634292873786));
#37923=CARTESIAN_POINT('Ctrl Pts',(0.338662659096756,-0.534387172794291,
1.6282662988526));
#37924=CARTESIAN_POINT('Ctrl Pts',(0.553233053245814,-0.306912647437654,
1.64018966896734));
#37925=CARTESIAN_POINT('Ctrl Pts',(0.63264703504302,-0.004457885988231,
1.65211303908208));
#37926=CARTESIAN_POINT('Ctrl Pts',(0.557503379173826,0.299084810277989,
1.66403640919682));
#37927=CARTESIAN_POINT('Ctrl Pts',(0.346160212094308,0.529562476556959,
1.67595977931156));
#37928=CARTESIAN_POINT('Ctrl Pts',(0.0502486745876001,0.630661949020613,
1.6878831494263));
#37929=CARTESIAN_POINT('Ctrl Pts',(-0.257937943046404,0.577697854759531,
1.69980651954104));
#37930=CARTESIAN_POINT('Ctrl Pts',(-0.503111198644335,0.383582524720304,
1.71172988965578));
#37931=CARTESIAN_POINT('Ctrl Pts',(-0.597016914950347,0.162533434793575,
1.7208881387779));
#37932=CARTESIAN_POINT('Ctrl Pts',(-0.606855428137301,0.0307581865173095,
1.7260719311951));
#37933=CARTESIAN_POINT('Ctrl Pts',(-0.606828099052645,1.21067951662536E-5,
1.72728126690739));
#37934=CARTESIAN_POINT('Origin',(0.,0.,0.422718733092612));
#37935=CARTESIAN_POINT('',(-0.606798126054683,-1.59915840535429E-6,1.39771873309261));
#37936=CARTESIAN_POINT('',(-0.606877435462865,1.29655716943344E-5,1.42728126690739));
#37937=CARTESIAN_POINT('',(-0.60685,-1.25452023855349E-14,0.422718733092612));
#37938=CARTESIAN_POINT('Ctrl Pts',(-0.606798126054683,-1.59915840541175E-6,
1.39771873309261));
#37939=CARTESIAN_POINT('Ctrl Pts',(-0.606802594249528,-0.0488192602443514,
1.39963876765163));
#37940=CARTESIAN_POINT('Ctrl Pts',(-0.588931640835428,-0.198685886988713,
1.40553325891556));
#37941=CARTESIAN_POINT('Ctrl Pts',(-0.466892707499535,-0.426934784279433,
1.41540220688441));
#37942=CARTESIAN_POINT('Ctrl Pts',(-0.205385625641773,-0.598396904339966,
1.42732557699915));
#37943=CARTESIAN_POINT('Ctrl Pts',(0.106297769497149,-0.623668898169518,
1.43924894711389));
#37944=CARTESIAN_POINT('Ctrl Pts',(0.392012306461527,-0.496576743239674,
1.45117231722863));
#37945=CARTESIAN_POINT('Ctrl Pts',(0.581957082335726,-0.248169427334259,
1.46309568734337));
#37946=CARTESIAN_POINT('Ctrl Pts',(0.629728028915714,0.0608664106211582,
1.47501905745811));
#37947=CARTESIAN_POINT('Ctrl Pts',(0.523654563249111,0.355032405185257,
1.48694242757285));
#37948=CARTESIAN_POINT('Ctrl Pts',(0.289650745423433,0.562462937465252,
1.49886579768759));
#37949=CARTESIAN_POINT('Ctrl Pts',(-0.0151156026373754,0.632482117450919,
1.51078916780233));
#37950=CARTESIAN_POINT('Ctrl Pts',(-0.316189164454242,0.547984053267855,
1.52271253791707));
#37951=CARTESIAN_POINT('Ctrl Pts',(-0.540016782097706,0.329611870817301,
1.53463590803181));
#37952=CARTESIAN_POINT('Ctrl Pts',(-0.604262251146843,0.120658502190452,
1.54297130642366));
#37953=CARTESIAN_POINT('Ctrl Pts',(-0.606897200403655,0.00983191954734194,
1.54733224811059));
#37954=CARTESIAN_POINT('Ctrl Pts',(-0.60688975719765,9.64797104193935E-6,
1.54771873309261));
#37955=CARTESIAN_POINT('Ctrl Pts',(-0.606877435462865,1.29655716943379E-5,
1.42728126690739));
#37956=CARTESIAN_POINT('Ctrl Pts',(-0.606795962787138,-0.0864950896955681,
1.43068497027718));
#37957=CARTESIAN_POINT('Ctrl Pts',(-0.566285570456084,-0.274091234023481,
1.43806313035188));
#37958=CARTESIAN_POINT('Ctrl Pts',(-0.379662553523367,-0.506081476332481,
1.4494157471315));
#37959=CARTESIAN_POINT('Ctrl Pts',(-0.0909043756851951,-0.626097843558096,
1.46133911724624));
#37960=CARTESIAN_POINT('Ctrl Pts',(0.220062008878289,-0.593156663530657,
1.47326248736098));
#37961=CARTESIAN_POINT('Ctrl Pts',(0.477266596511919,-0.415305563499184,
1.48518585747572));
#37962=CARTESIAN_POINT('Ctrl Pts',(0.617873548883792,-0.135994091149731,
1.49710922759046));
#37963=CARTESIAN_POINT('Ctrl Pts',(0.607532173409899,0.176541138367681,
1.5090325977052));
#37964=CARTESIAN_POINT('Ctrl Pts',(0.44876889853771,0.445946847509907,1.52095596781994));
#37965=CARTESIAN_POINT('Ctrl Pts',(0.180370060014882,0.606406428909711,
1.53287933793468));
#37966=CARTESIAN_POINT('Ctrl Pts',(-0.132093715531906,0.618719132473601,
1.54480270804942));
#37967=CARTESIAN_POINT('Ctrl Pts',(-0.412286607098983,0.479876931929719,
1.55672607816416));
#37968=CARTESIAN_POINT('Ctrl Pts',(-0.575241902336924,0.247363534614087,
1.56755226445015));
#37969=CARTESIAN_POINT('Ctrl Pts',(-0.606765191807545,0.0731272960492705,
1.57440399403123));
#37970=CARTESIAN_POINT('Ctrl Pts',(-0.606835914664954,-1.54868133571684E-5,
1.57728126690739));
#37971=CARTESIAN_POINT('Origin',(0.,0.,0.422718733092612));
#37972=CARTESIAN_POINT('',(-0.606896670952539,-6.59829139776882E-6,1.24771873309261));
#37973=CARTESIAN_POINT('',(-0.606801243923172,-5.85749501685884E-6,1.27728126690739));
#37974=CARTESIAN_POINT('',(-0.60685,-1.25452023855349E-14,0.422718733092612));
#37975=CARTESIAN_POINT('Ctrl Pts',(-0.606896670952539,-6.59829139778353E-6,
1.24771873309261));
#37976=CARTESIAN_POINT('Ctrl Pts',(-0.606900224819954,-0.00641328249130264,
1.24797083048776));
#37977=CARTESIAN_POINT('Ctrl Pts',(-0.605234866882428,-0.113823082303296,
1.25219738458781));
#37978=CARTESIAN_POINT('Ctrl Pts',(-0.545505882342923,-0.320445693797292,
1.26039839539279));
#37979=CARTESIAN_POINT('Ctrl Pts',(-0.325397796916506,-0.542566478973631,
1.27232176550753));
#37980=CARTESIAN_POINT('Ctrl Pts',(-0.0257940712861588,-0.632136675277145,
1.28424513562227));
#37981=CARTESIAN_POINT('Ctrl Pts',(0.280111221932506,-0.567274019933433,
1.29616850573701));
#37982=CARTESIAN_POINT('Ctrl Pts',(0.517584518601595,-0.363824650687545,
1.30809187585175));
#37983=CARTESIAN_POINT('Ctrl Pts',(0.628610392897891,-0.0714918476801203,
1.32001524596649));
#37984=CARTESIAN_POINT('Ctrl Pts',(0.586064896718421,0.238306624285571,
1.33193861608123));
#37985=CARTESIAN_POINT('Ctrl Pts',(0.4003420200921,0.489886086036881,1.34386198619597));
#37986=CARTESIAN_POINT('Ctrl Pts',(0.116814408801508,0.621784934073119,
1.35578535631071));
#37987=CARTESIAN_POINT('Ctrl Pts',(-0.195251306621063,0.601779891327988,
1.36770872642545));
#37988=CARTESIAN_POINT('Ctrl Pts',(-0.459616552748575,0.434758248666402,
1.37963209654019));
#37989=CARTESIAN_POINT('Ctrl Pts',(-0.587206566371662,0.205523141855759,
1.38963543209591));
#37990=CARTESIAN_POINT('Ctrl Pts',(-0.606793345120716,0.052232921087437,
1.39566431094672));
#37991=CARTESIAN_POINT('Ctrl Pts',(-0.606798126054683,-1.59915840541175E-6,
1.39771873309261));
#37992=CARTESIAN_POINT('Ctrl Pts',(-0.606801243923172,-5.85749501688312E-6,
1.27728126690739));
#37993=CARTESIAN_POINT('Ctrl Pts',(-0.60681613156811,-0.0441377730285598,
1.2790170331133));
#37994=CARTESIAN_POINT('Ctrl Pts',(-0.591194722324054,-0.189310005818757,
1.28472725602413));
#37995=CARTESIAN_POINT('Ctrl Pts',(-0.476652695565553,-0.416010003536527,
1.29441193563987));
#37996=CARTESIAN_POINT('Ctrl Pts',(-0.219185713483245,-0.593481034437674,
1.30633530575462));
#37997=CARTESIAN_POINT('Ctrl Pts',(0.0918289839862619,-0.625962900603877,
1.31825867586936));
#37998=CARTESIAN_POINT('Ctrl Pts',(0.380409590197501,-0.505520186459593,
1.3301820459841));
#37999=CARTESIAN_POINT('Ctrl Pts',(0.576055013076121,-0.26157740181873,
1.34210541609884));
#38000=CARTESIAN_POINT('Ctrl Pts',(0.630968499564522,0.0462695125289182,
1.35402878621358));
#38001=CARTESIAN_POINT('Ctrl Pts',(0.531734523173002,0.34281264868491,1.36595215632832));
#38002=CARTESIAN_POINT('Ctrl Pts',(0.302596236614874,0.555605645056675,
1.37787552644306));
#38003=CARTESIAN_POINT('Ctrl Pts',(-0.000467201806429895,0.632662545876497,
1.3897988965578));
#38004=CARTESIAN_POINT('Ctrl Pts',(-0.303416501450367,0.555158123312486,
1.40172226667254));
#38005=CARTESIAN_POINT('Ctrl Pts',(-0.532240256115767,0.3420269360772,1.41364563678728));
#38006=CARTESIAN_POINT('Ctrl Pts',(-0.6028333913918,0.130031956601212,1.42216530353223));
#38007=CARTESIAN_POINT('Ctrl Pts',(-0.606891097288336,0.0145191535953422,
1.42671051357226));
#38008=CARTESIAN_POINT('Ctrl Pts',(-0.606877435462865,1.29655716943379E-5,
1.42728126690739));
#38009=CARTESIAN_POINT('Origin',(0.,0.,0.422718733092612));
#38010=CARTESIAN_POINT('',(-0.606814611697072,1.20472578674858E-5,1.09771873309261));
#38011=CARTESIAN_POINT('',(-0.606902028636254,-1.83691493421678E-6,1.12728126690739));
#38012=CARTESIAN_POINT('',(-0.60685,-1.25452023855349E-14,0.422718733092612));
#38013=CARTESIAN_POINT('Ctrl Pts',(-0.606814611697072,1.20472578674785E-5,
1.09771873309261));
#38014=CARTESIAN_POINT('Ctrl Pts',(-0.606768181291156,-0.0650367723393511,
1.1002773500288));
#38015=CARTESIAN_POINT('Ctrl Pts',(-0.580164840953881,-0.231166986996602,
1.10681042366989));
#38016=CARTESIAN_POINT('Ctrl Pts',(-0.431166912267969,-0.462987261281848,
1.1173179540159));
#38017=CARTESIAN_POINT('Ctrl Pts',(-0.156756874309222,-0.612935064016377,
1.12924132413064));
#38018=CARTESIAN_POINT('Ctrl Pts',(0.155949329750418,-0.613141025290557,
1.14116469424539));
#38019=CARTESIAN_POINT('Ctrl Pts',(0.4305566532234,-0.463554828158465,1.15308806436012));
#38020=CARTESIAN_POINT('Ctrl Pts',(0.59997771816483,-0.200720821166321,
1.16501143447486));
#38021=CARTESIAN_POINT('Ctrl Pts',(0.622822459401631,0.111149873634038,
1.17693480458961));
#38022=CARTESIAN_POINT('Ctrl Pts',(0.493509839363413,0.395866326927988,
1.18885817470434));
#38023=CARTESIAN_POINT('Ctrl Pts',(0.243631311999152,0.583871470580239,
1.20078154481908));
#38024=CARTESIAN_POINT('Ctrl Pts',(-0.0657670624710998,0.629235094251649,
1.21270491493383));
#38025=CARTESIAN_POINT('Ctrl Pts',(-0.359098349871265,0.520874731066591,
1.22462828504856));
#38026=CARTESIAN_POINT('Ctrl Pts',(-0.560353771743364,0.290244704085391,
1.23629955776816));
#38027=CARTESIAN_POINT('Ctrl Pts',(-0.60684419610863,0.0945916841009262,
1.24399637378284));
#38028=CARTESIAN_POINT('Ctrl Pts',(-0.606896670952539,-6.59829139778353E-6,
1.24771873309261));
#38029=CARTESIAN_POINT('Ctrl Pts',(-0.606902028636254,-1.83691493418382E-6,
1.12728126690739));
#38030=CARTESIAN_POINT('Ctrl Pts',(-0.60690232638052,-0.00172556794049109,
1.12734909594943));
#38031=CARTESIAN_POINT('Ctrl Pts',(-0.606473854563749,-0.104451525220278,
1.13139138169638));
#38032=CARTESIAN_POINT('Ctrl Pts',(-0.552779171463751,-0.307729268722068,
1.13940812414825));
#38033=CARTESIAN_POINT('Ctrl Pts',(-0.337873026968778,-0.534886841191037,
1.15133149426299));
#38034=CARTESIAN_POINT('Ctrl Pts',(-0.0404235068239226,-0.631369982916851,
1.16325486437773));
#38035=CARTESIAN_POINT('Ctrl Pts',(0.26690159510024,-0.573607578197252,
1.17517823449247));
#38036=CARTESIAN_POINT('Ctrl Pts',(0.509021851217201,-0.375711152636948,
1.18710160460721));
#38037=CARTESIAN_POINT('Ctrl Pts',(0.626786569823609,-0.0860273858787084,
1.19902497472195));
#38038=CARTESIAN_POINT('Ctrl Pts',(0.591425483303132,0.224673124632266,
1.21094834483669));
#38039=CARTESIAN_POINT('Ctrl Pts',(0.411577409244242,0.480485329049876,
1.22287171495143));
#38040=CARTESIAN_POINT('Ctrl Pts',(0.131179761858824,0.618913552373053,
1.23479508506618));
#38041=CARTESIAN_POINT('Ctrl Pts',(-0.181265487721769,0.606139371921474,
1.24671845518091));
#38042=CARTESIAN_POINT('Ctrl Pts',(-0.449427044757826,0.445283557604159,
1.25864182529566));
#38043=CARTESIAN_POINT('Ctrl Pts',(-0.584737949218254,0.214896975434926,
1.26882942920448));
#38044=CARTESIAN_POINT('Ctrl Pts',(-0.606782042702892,0.0569129255016839,
1.27504257640839));
#38045=CARTESIAN_POINT('Ctrl Pts',(-0.606801243923172,-5.85749501688312E-6,
1.27728126690739));
#38046=CARTESIAN_POINT('Origin',(0.,0.,0.422718733092612));
#38047=CARTESIAN_POINT('',(-0.606852195439347,-1.57862025725476E-5,0.947718733092612));
#38048=CARTESIAN_POINT('',(-0.60680575058562,8.7320520037043E-6,0.977281266907388));
#38049=CARTESIAN_POINT('',(-0.60685,-1.25452023855349E-14,0.422718733092612));
#38050=CARTESIAN_POINT('Ctrl Pts',(-0.606852195439347,-1.5786202572584E-5,
0.947718733092612));
#38051=CARTESIAN_POINT('Ctrl Pts',(-0.606875617872986,-0.0226558951432442,
0.948609412864922));
#38052=CARTESIAN_POINT('Ctrl Pts',(-0.600088688538456,-0.146308396998802,
0.953474549342146));
#38053=CARTESIAN_POINT('Ctrl Pts',(-0.518063329334561,-0.363142530047957,
0.962314142524282));
#38054=CARTESIAN_POINT('Ctrl Pts',(-0.280858238968939,-0.566904542191545,
0.974237512639023));
#38055=CARTESIAN_POINT('Ctrl Pts',(0.0249613464089441,-0.632170104895623,
0.986160882753763));
#38056=CARTESIAN_POINT('Ctrl Pts',(0.324682801338475,-0.542994649017271,
0.998084252868503));
#38057=CARTESIAN_POINT('Ctrl Pts',(0.545083291589825,-0.321164001053741,
1.01000762298324));
#38058=CARTESIAN_POINT('Ctrl Pts',(0.632318328233213,-0.0208720416904643,
1.02193099309798));
#38059=CARTESIAN_POINT('Ctrl Pts',(0.565076134877199,0.284519018936116,
1.03385436321272));
#38060=CARTESIAN_POINT('Ctrl Pts',(0.35978417741182,0.520401245221327,1.04577773332746));
#38061=CARTESIAN_POINT('Ctrl Pts',(0.0665958857068623,0.62914791452485,
1.0577011034422));
#38062=CARTESIAN_POINT('Ctrl Pts',(-0.242861977025874,0.584191895235632,
1.06962447355694));
#38063=CARTESIAN_POINT('Ctrl Pts',(-0.492987943452569,0.396516075278645,
1.08154784367169));
#38064=CARTESIAN_POINT('Ctrl Pts',(-0.59484605707748,0.173030452641354,
1.09091259685024));
#38065=CARTESIAN_POINT('Ctrl Pts',(-0.606840304490021,0.0360075510756424,
1.09630289332388));
#38066=CARTESIAN_POINT('Ctrl Pts',(-0.606814611697072,1.20472578674785E-5,
1.09771873309261));
#38067=CARTESIAN_POINT('Ctrl Pts',(-0.60680575058562,8.73205200368002E-6,
0.977281266907388));
#38068=CARTESIAN_POINT('Ctrl Pts',(-0.606775110747621,-0.0603578794789066,
0.97965561549047));
#38069=CARTESIAN_POINT('Ctrl Pts',(-0.582843583723735,-0.22179680306636,
0.986004420778464));
#38070=CARTESIAN_POINT('Ctrl Pts',(-0.441771228592792,-0.452880002671609,
0.996327682771373));
#38071=CARTESIAN_POINT('Ctrl Pts',(-0.170906611750865,-0.6091412359152,
1.00825105288611));
#38072=CARTESIAN_POINT('Ctrl Pts',(0.141710993725228,-0.616587471077492,
1.02017442300085));
#38073=CARTESIAN_POINT('Ctrl Pts',(0.419708186042773,-0.473399570976854,
1.03209779311559));
#38074=CARTESIAN_POINT('Ctrl Pts',(0.595169432313768,-0.214558761349135,
1.04402116323033));
#38075=CARTESIAN_POINT('Ctrl Pts',(0.625229033275726,0.0966993856312912,
1.05594453334507));
#38076=CARTESIAN_POINT('Ctrl Pts',(0.502543339876973,0.384333587886446,
1.06786790345981));
#38077=CARTESIAN_POINT('Ctrl Pts',(0.257084828369703,0.578073962615934,
1.07979127357455));
#38078=CARTESIAN_POINT('Ctrl Pts',(-0.0511802639184789,0.630589165636079,
1.09171464368929));
#38079=CARTESIAN_POINT('Ctrl Pts',(-0.346941866986512,0.529049578172294,
1.10363801380403));
#38080=CARTESIAN_POINT('Ctrl Pts',(-0.556744209089362,0.29957451493303,
1.11549355487673));
#38081=CARTESIAN_POINT('Ctrl Pts',(-0.606884879993859,0.0992768069387203,
1.12337463924452));
#38082=CARTESIAN_POINT('Ctrl Pts',(-0.606902028636254,-1.83691493418382E-6,
1.12728126690739));
#38083=CARTESIAN_POINT('Origin',(0.,0.,0.422718733092612));
#38084=CARTESIAN_POINT('',(-0.606861373480359,1.53279143725419E-5,0.797718733092612));
#38085=CARTESIAN_POINT('',(-0.606867041669442,-1.46440865503583E-5,0.827281266907388));
#38086=CARTESIAN_POINT('',(-0.60685,-1.25452023855349E-14,0.422718733092612));
#38087=CARTESIAN_POINT('Ctrl Pts',(-0.606861373480359,1.53279143725385E-5,
0.797718733092612));
#38088=CARTESIAN_POINT('Ctrl Pts',(-0.606777537923217,-0.0812504538222047,
0.800915932405962));
#38089=CARTESIAN_POINT('Ctrl Pts',(-0.569922761574246,-0.263612138122336,
0.808087588424225));
#38090=CARTESIAN_POINT('Ctrl Pts',(-0.392666097338528,-0.496059852941866,
0.819233701147401));
#38091=CARTESIAN_POINT('Ctrl Pts',(-0.107119225715726,-0.623528367336511,
0.831157071262142));
#38092=CARTESIAN_POINT('Ctrl Pts',(0.204597189954239,-0.59866691871355,
0.843080441376881));
#38093=CARTESIAN_POINT('Ctrl Pts',(0.466329908650049,-0.427549452094589,
0.855003811491622));
#38094=CARTESIAN_POINT('Ctrl Pts',(0.614136857577049,-0.151980358083104,
0.866927181606362));
#38095=CARTESIAN_POINT('Ctrl Pts',(0.611908363121538,0.160717966477571,
0.878850551721102));
#38096=CARTESIAN_POINT('Ctrl Pts',(0.460188853366613,0.434152427784503,
0.890773921835841));
#38097=CARTESIAN_POINT('Ctrl Pts',(0.1960438512529,0.601522167555102,0.902697291950583));
#38098=CARTESIAN_POINT('Ctrl Pts',(-0.115995241116418,0.621938272442033,
0.914620662065322));
#38099=CARTESIAN_POINT('Ctrl Pts',(-0.399696354445721,0.490413024348575,
0.926544032180063));
#38100=CARTESIAN_POINT('Ctrl Pts',(-0.571852165804536,0.257853209547959,
0.937576722522492));
#38101=CARTESIAN_POINT('Ctrl Pts',(-0.606771100569104,0.0783704620017294,
0.944634956160009));
#38102=CARTESIAN_POINT('Ctrl Pts',(-0.606852195439347,-1.5786202572584E-5,
0.947718733092612));
#38103=CARTESIAN_POINT('Ctrl Pts',(-0.606867041669442,-1.46440865504086E-5,
0.827281266907388));
#38104=CARTESIAN_POINT('Ctrl Pts',(-0.606885242107981,-0.0179695869580834,
0.827987678326596));
#38105=CARTESIAN_POINT('Ctrl Pts',(-0.601710640579271,-0.13693331365204,
0.832668546450717));
#38106=CARTESIAN_POINT('Ctrl Pts',(-0.526332568352355,-0.351050058657002,
0.841323871279751));
#38107=CARTESIAN_POINT('Ctrl Pts',(-0.293908927059336,-0.560249638256679,
0.85324724139449));
#38108=CARTESIAN_POINT('Ctrl Pts',(0.0103175303644349,-0.632578583371251,
0.865170611509231));
#38109=CARTESIAN_POINT('Ctrl Pts',(0.31202338494245,-0.550366716242752,
0.877093981623972));
#38110=CARTESIAN_POINT('Ctrl Pts',(0.537501007448335,-0.333698639877864,
0.889017351738711));
#38111=CARTESIAN_POINT('Ctrl Pts',(0.631665550747977,-0.0355070026353613,
0.900940721853452));
#38112=CARTESIAN_POINT('Ctrl Pts',(0.571512339483762,0.271359099787061,
0.912864091968191));
#38113=CARTESIAN_POINT('Ctrl Pts',(0.371736980381227,0.51193137495119,0.924787462082931));
#38114=CARTESIAN_POINT('Ctrl Pts',(0.0811451820615032,0.627437307350318,
0.936710832197672));
#38115=CARTESIAN_POINT('Ctrl Pts',(-0.229270623235126,0.589658457546506,
0.948634202312412));
#38116=CARTESIAN_POINT('Ctrl Pts',(-0.483674939990074,0.407824309791941,
0.960557572427152));
#38117=CARTESIAN_POINT('Ctrl Pts',(-0.592785805966434,0.182407101947706,
0.970106593958811));
#38118=CARTESIAN_POINT('Ctrl Pts',(-0.606826399219094,0.0406906715474857,
0.975681158785556));
#38119=CARTESIAN_POINT('Ctrl Pts',(-0.60680575058562,8.73205200368002E-6,
0.977281266907388));
#38120=CARTESIAN_POINT('Origin',(1.1271216279739E-16,-2.42910627858037E-17,
1.7475));
#38121=CARTESIAN_POINT('',(0.365377360036753,0.588264935868672,1.7475));
#38122=CARTESIAN_POINT('Ctrl Pts',(0.298621660385102,-0.528323265936629,
1.7475));
#38123=CARTESIAN_POINT('Ctrl Pts',(0.312129560427946,-0.521873925222218,
1.7475));
#38124=CARTESIAN_POINT('Ctrl Pts',(0.325379783927112,-0.514929522576798,
1.7475));
#38125=CARTESIAN_POINT('Ctrl Pts',(0.338343379574887,-0.50750179203716,
1.7475));
#38126=CARTESIAN_POINT('Ctrl Pts',(0.36077543119364,-0.494648935514754,
1.7475));
#38127=CARTESIAN_POINT('Ctrl Pts',(0.382349984001486,-0.480350324006014,
1.7475));
#38128=CARTESIAN_POINT('Ctrl Pts',(0.402968596112581,-0.464732386935322,
1.7475));
#38129=CARTESIAN_POINT('Ctrl Pts',(0.412005321941232,-0.457887357087701,
1.7475));
#38130=CARTESIAN_POINT('Ctrl Pts',(0.420858285551003,-0.450788564790034,
1.7475));
#38131=CARTESIAN_POINT('Ctrl Pts',(0.429518414483015,-0.4434452100822,1.7475));
#38132=CARTESIAN_POINT('Ctrl Pts',(0.43632784881018,-0.437671151518334,
1.7475));
#38133=CARTESIAN_POINT('Ctrl Pts',(0.443012226475618,-0.431750667617364,
1.7475));
#38134=CARTESIAN_POINT('Ctrl Pts',(0.449562091487209,-0.425694086415582,
1.7475));
#38135=CARTESIAN_POINT('Ctrl Pts',(0.470631367154316,-0.406211581247191,
1.7475));
#38136=CARTESIAN_POINT('Ctrl Pts',(0.490328809845417,-0.38530767574534,
1.7475));
#38137=CARTESIAN_POINT('Ctrl Pts',(0.508518158509955,-0.363142905055253,
1.7475));
#38138=CARTESIAN_POINT('Ctrl Pts',(0.516442502170421,-0.353486635150102,
1.7475));
#38139=CARTESIAN_POINT('Ctrl Pts',(0.524080348515509,-0.343590638760223,
1.7475));
#38140=CARTESIAN_POINT('Ctrl Pts',(0.531418980886992,-0.333466452816219,
1.7475));
#38141=CARTESIAN_POINT('Ctrl Pts',(0.537374715310306,-0.325250076837359,
1.7475));
#38142=CARTESIAN_POINT('Ctrl Pts',(0.543135758395536,-0.316879252360657,
1.7475));
#38143=CARTESIAN_POINT('Ctrl Pts',(0.54867910249215,-0.308385145523163,
1.7475));
#38144=CARTESIAN_POINT('Ctrl Pts',(0.55198380721638,-0.303321322223592,
1.7475));
#38145=CARTESIAN_POINT('Ctrl Pts',(0.555212267947236,-0.298212252230868,
1.7475));
#38146=CARTESIAN_POINT('Ctrl Pts',(0.558363346279548,-0.293059483804602,
1.7475));
#38147=CARTESIAN_POINT('Ctrl Pts',(0.574646861887172,-0.266432032423531,
1.7475));
#38148=CARTESIAN_POINT('Ctrl Pts',(0.588867110740308,-0.238640752575286,
1.7475));
#38149=CARTESIAN_POINT('Ctrl Pts',(0.600996416107695,-0.209953544278971,
1.7475));
#38150=CARTESIAN_POINT('Ctrl Pts',(0.60904684941943,-0.190913339560379,
1.7475));
#38151=CARTESIAN_POINT('Ctrl Pts',(0.616175424072814,-0.171477546535687,
1.7475));
#38152=CARTESIAN_POINT('Ctrl Pts',(0.62236375672442,-0.151717176539816,
1.7475));
#38153=CARTESIAN_POINT('Ctrl Pts',(0.627198272740129,-0.136279767046878,
1.7475));
#38154=CARTESIAN_POINT('Ctrl Pts',(0.631458783571978,-0.12064412869836,
1.7475));
#38155=CARTESIAN_POINT('Ctrl Pts',(0.635132620377226,-0.104842682574537,
1.7475));
#38156=CARTESIAN_POINT('Ctrl Pts',(0.636966965175414,-0.0969530287772681,
1.7475));
#38157=CARTESIAN_POINT('Ctrl Pts',(0.638655092015668,-0.0890204207899287,
1.7475));
#38158=CARTESIAN_POINT('Ctrl Pts',(0.640191602362932,-0.0810701616342577,
1.7475));
#38159=CARTESIAN_POINT('Ctrl Pts',(0.646042674165708,-0.0507953657285062,
1.7475));
#38160=CARTESIAN_POINT('Ctrl Pts',(0.649715322524794,-0.0201981047171755,
1.7475));
#38161=CARTESIAN_POINT('Ctrl Pts',(0.651168459719186,0.0104864299067928,
1.7475));
#38162=CARTESIAN_POINT('Ctrl Pts',(0.652471176970355,0.0379946877319891,
1.7475));
#38163=CARTESIAN_POINT('Ctrl Pts',(0.651989846702894,0.0655739643226442,
1.7475));
#38164=CARTESIAN_POINT('Ctrl Pts',(0.649775510912856,0.0930641486169698,
1.7475));
#38165=CARTESIAN_POINT('Ctrl Pts',(0.648444472381905,0.109588514380875,
1.7475));
#38166=CARTESIAN_POINT('Ctrl Pts',(0.646486693282225,0.126080801141174,
1.7475));
#38167=CARTESIAN_POINT('Ctrl Pts',(0.643908241891283,0.142506225480307,
1.7475));
#38168=CARTESIAN_POINT('Ctrl Pts',(0.642438854943278,0.151866612968763,
1.7475));
#38169=CARTESIAN_POINT('Ctrl Pts',(0.64076665037931,0.16121004588847,1.7475));
#38170=CARTESIAN_POINT('Ctrl Pts',(0.638898832841581,0.170500427755555,
1.7475));
#38171=CARTESIAN_POINT('Ctrl Pts',(0.63245057878856,0.202573551237074,1.7475));
#38172=CARTESIAN_POINT('Ctrl Pts',(0.623667987104589,0.234074759209373,
1.7475));
#38173=CARTESIAN_POINT('Ctrl Pts',(0.61264701184346,0.26474553850838,1.7475));
#38174=CARTESIAN_POINT('Ctrl Pts',(0.60450404702486,0.287406970085287,1.7475));
#38175=CARTESIAN_POINT('Ctrl Pts',(0.595137974178845,0.309615432087503,
1.7475));
#38176=CARTESIAN_POINT('Ctrl Pts',(0.584569321392081,0.331264976054902,
1.7475));
#38177=CARTESIAN_POINT('Ctrl Pts',(0.577683443413199,0.345370474746717,
1.7475));
#38178=CARTESIAN_POINT('Ctrl Pts',(0.570286748895561,0.359238659304976,
1.7475));
#38179=CARTESIAN_POINT('Ctrl Pts',(0.562398175902974,0.372848797290938,
1.7475));
#38180=CARTESIAN_POINT('Ctrl Pts',(0.557821697642751,0.380744585371992,
1.7475));
#38181=CARTESIAN_POINT('Ctrl Pts',(0.553079623629564,0.388553501647874,
1.7475));
#38182=CARTESIAN_POINT('Ctrl Pts',(0.548175280753752,0.396271270275225,
1.7475));
#38183=CARTESIAN_POINT('Ctrl Pts',(0.54441947391472,0.402181633585185,1.7475));
#38184=CARTESIAN_POINT('Ctrl Pts',(0.540573489524936,0.408030640947142,
1.7475));
#38185=CARTESIAN_POINT('Ctrl Pts',(0.536640687844456,0.413815061624329,
1.7475));
#38186=CARTESIAN_POINT('Ctrl Pts',(0.518064650144307,0.441136962219085,
1.7475));
#38187=CARTESIAN_POINT('Ctrl Pts',(0.497547892662459,0.467031617110893,
1.7475));
#38188=CARTESIAN_POINT('Ctrl Pts',(0.475299963702939,0.491327450504889,
1.7475));
#38189=CARTESIAN_POINT('Ctrl Pts',(0.452956133924144,0.515728012313458,
1.7475));
#38190=CARTESIAN_POINT('Ctrl Pts',(0.4288654429408,0.538516969116918,1.7475));
#38191=CARTESIAN_POINT('Ctrl Pts',(0.40319570009474,0.55949438395691,1.7475));
#38192=CARTESIAN_POINT('Ctrl Pts',(0.390944685394277,0.569505961366299,
1.7475));
#38193=CARTESIAN_POINT('Ctrl Pts',(0.378333424832096,0.579104441213069,
1.7475));
#38194=CARTESIAN_POINT('Ctrl Pts',(0.365377360036757,0.58826493586867,1.7475));
#38195=CARTESIAN_POINT('',(-0.6925,-8.48067908409542E-17,1.7475));
#38196=CARTESIAN_POINT('Origin',(0.,0.,1.7475));
#38197=CARTESIAN_POINT('',(-0.235097938825072,0.6513885053826,1.7475));
#38198=CARTESIAN_POINT('Origin',(0.,0.,1.7475));
#38199=CARTESIAN_POINT('Ctrl Pts',(-0.235110047033021,0.651400850437653,
1.7475));
#38200=CARTESIAN_POINT('Ctrl Pts',(-0.250726404295242,0.644704975861436,
1.7475));
#38201=CARTESIAN_POINT('Ctrl Pts',(-0.266073638896426,0.63743919485856,
1.7475));
#38202=CARTESIAN_POINT('Ctrl Pts',(-0.281117933505346,0.629609469190081,
1.7475));
#38203=CARTESIAN_POINT('Ctrl Pts',(-0.306227709788298,0.616541215409952,
1.7475));
#38204=CARTESIAN_POINT('Ctrl Pts',(-0.330494626537405,0.601902955535088,
1.7475));
#38205=CARTESIAN_POINT('Ctrl Pts',(-0.353792461978798,0.585802237765094,
1.7475));
#38206=CARTESIAN_POINT('Ctrl Pts',(-0.363257657218618,0.579261010466207,
1.7475));
#38207=CARTESIAN_POINT('Ctrl Pts',(-0.372562694887073,0.572478166005196,
1.7475));
#38208=CARTESIAN_POINT('Ctrl Pts',(-0.381698167526852,0.565460062323596,
1.7475));
#38209=CARTESIAN_POINT('Ctrl Pts',(-0.388587317293776,0.560167641312798,
1.7475));
#38210=CARTESIAN_POINT('Ctrl Pts',(-0.395379904167447,0.554741287066626,
1.7475));
#38211=CARTESIAN_POINT('Ctrl Pts',(-0.402060898620473,0.549193220426858,
1.7475));
#38212=CARTESIAN_POINT('Ctrl Pts',(-0.427000921363888,0.528482395241975,
1.7475));
#38213=CARTESIAN_POINT('Ctrl Pts',(-0.450429447471031,0.506047454222527,
1.7475));
#38214=CARTESIAN_POINT('Ctrl Pts',(-0.472148997050359,0.482046003595282,
1.7475));
#38215=CARTESIAN_POINT('Ctrl Pts',(-0.485933688015498,0.466813064329979,
1.7475));
#38216=CARTESIAN_POINT('Ctrl Pts',(-0.499029320708669,0.450948438789647,
1.7475));
#38217=CARTESIAN_POINT('Ctrl Pts',(-0.511376451188905,0.434487136701648,
1.7475));
#38218=CARTESIAN_POINT('Ctrl Pts',(-0.515784428166145,0.42861038333491,
1.7475));
#38219=CARTESIAN_POINT('Ctrl Pts',(-0.520091038783305,0.422665405887042,
1.7475));
#38220=CARTESIAN_POINT('Ctrl Pts',(-0.524293998238925,0.416654482991514,
1.7475));
#38221=CARTESIAN_POINT('Ctrl Pts',(-0.526867829583898,0.412973481087001,
1.7475));
#38222=CARTESIAN_POINT('Ctrl Pts',(-0.529402816011311,0.409267709604622,
1.7475));
#38223=CARTESIAN_POINT('Ctrl Pts',(-0.531898464539994,0.405537607383136,
1.7475));
#38224=CARTESIAN_POINT('Ctrl Pts',(-0.549961436224517,0.378539923200975,
1.7475));
#38225=CARTESIAN_POINT('Ctrl Pts',(-0.565967543335006,0.350269649024675,
1.7475));
#38226=CARTESIAN_POINT('Ctrl Pts',(-0.579839900985994,0.32098090427459,
1.7475));
#38227=CARTESIAN_POINT('Ctrl Pts',(-0.593599071234153,0.291931132382169,
1.7475));
#38228=CARTESIAN_POINT('Ctrl Pts',(-0.605259453146915,0.26187818221775,
1.7475));
#38229=CARTESIAN_POINT('Ctrl Pts',(-0.614696977596504,0.231057442915654,
1.7475));
#38230=CARTESIAN_POINT('Ctrl Pts',(-0.617111680413263,0.223171590390992,
1.7475));
#38231=CARTESIAN_POINT('Ctrl Pts',(-0.61938059889099,0.215235463519407,
1.7475));
#38232=CARTESIAN_POINT('Ctrl Pts',(-0.621501097336438,0.20725302330997,
1.7475));
#38233=CARTESIAN_POINT('Ctrl Pts',(-0.623104950924263,0.201215449739949,
1.7475));
#38234=CARTESIAN_POINT('Ctrl Pts',(-0.624623079632104,0.195154132702508,
1.7475));
#38235=CARTESIAN_POINT('Ctrl Pts',(-0.626052823098529,0.189078984025834,
1.7475));
#38236=CARTESIAN_POINT('Ctrl Pts',(-0.633111115640263,0.159087466245572,
1.7475));
#38237=CARTESIAN_POINT('Ctrl Pts',(-0.638034496402489,0.128701730040447,
1.7475));
#38238=CARTESIAN_POINT('Ctrl Pts',(-0.640738798776169,0.0981336645007876,
1.7475));
#38239=CARTESIAN_POINT('Ctrl Pts',(-0.643080565572788,0.0716635176657487,
1.7475));
#38240=CARTESIAN_POINT('Ctrl Pts',(-0.643757566809919,0.0450560119454282,
1.7475));
#38241=CARTESIAN_POINT('Ctrl Pts',(-0.64278612619871,0.0184659463280288,
1.7475));
#38242=CARTESIAN_POINT('Ctrl Pts',(-0.642239859902067,0.00351366154119593,
1.7475));
#38243=CARTESIAN_POINT('Ctrl Pts',(-0.641171886318131,-0.0114330384723897,
1.7475));
#38244=CARTESIAN_POINT('Ctrl Pts',(-0.639581752812397,-0.0263454637940612,
1.7475));
#38245=CARTESIAN_POINT('Ctrl Pts',(-0.638821341683572,-0.033476672671481,
1.7475));
#38246=CARTESIAN_POINT('Ctrl Pts',(-0.637941215467033,-0.0406019406396422,
1.7475));
#38247=CARTESIAN_POINT('Ctrl Pts',(-0.636942000003881,-0.0477119642894318,
1.7475));
#38248=CARTESIAN_POINT('Ctrl Pts',(-0.632589769711551,-0.0786807207278065,
1.7475));
#38249=CARTESIAN_POINT('Ctrl Pts',(-0.626003853427657,-0.109216644694058,
1.7475));
#38250=CARTESIAN_POINT('Ctrl Pts',(-0.617229743220339,-0.139071444102893,
1.7475));
#38251=CARTESIAN_POINT('Ctrl Pts',(-0.609757341898868,-0.164497047073868,
1.7475));
#38252=CARTESIAN_POINT('Ctrl Pts',(-0.600696874850192,-0.189429019959063,
1.7475));
#38253=CARTESIAN_POINT('Ctrl Pts',(-0.590048925338361,-0.213702422383968,
1.7475));
#38254=CARTESIAN_POINT('Ctrl Pts',(-0.583925064501878,-0.227662569200301,
1.7475));
#38255=CARTESIAN_POINT('Ctrl Pts',(-0.577275630989656,-0.241404620746393,
1.7475));
#38256=CARTESIAN_POINT('Ctrl Pts',(-0.570116349152705,-0.254901826761342,
1.7475));
#38257=CARTESIAN_POINT('Ctrl Pts',(-0.5668391958013,-0.261080157903191,
1.7475));
#38258=CARTESIAN_POINT('Ctrl Pts',(-0.563455183893963,-0.267207155380128,
1.7475));
#38259=CARTESIAN_POINT('Ctrl Pts',(-0.559965690040735,-0.273280088753028,
1.7475));
#38260=CARTESIAN_POINT('Ctrl Pts',(-0.556766845051595,-0.278847191979564,
1.7475));
#38261=CARTESIAN_POINT('Ctrl Pts',(-0.553481278724128,-0.284365348726348,
1.7475));
#38262=CARTESIAN_POINT('Ctrl Pts',(-0.550114798073169,-0.289825771644315,
1.7475));
#38263=CARTESIAN_POINT('Ctrl Pts',(-0.533995756195628,-0.31597081592334,
1.7475));
#38264=CARTESIAN_POINT('Ctrl Pts',(-0.515996952170829,-0.340844013897456,
1.7475));
#38265=CARTESIAN_POINT('Ctrl Pts',(-0.496279916030761,-0.364250604271942,
1.7475));
#38266=CARTESIAN_POINT('Ctrl Pts',(-0.476916572129198,-0.387237317678789,
1.7475));
#38267=CARTESIAN_POINT('Ctrl Pts',(-0.455895145313256,-0.408810364956492,
1.7475));
#38268=CARTESIAN_POINT('Ctrl Pts',(-0.433336781370987,-0.428747731558718,
1.7475));
#38269=CARTESIAN_POINT('Ctrl Pts',(-0.423171392722634,-0.437732030271826,
1.7475));
#38270=CARTESIAN_POINT('Ctrl Pts',(-0.412693557907652,-0.446383597635371,
1.7475));
#38271=CARTESIAN_POINT('Ctrl Pts',(-0.401912945313201,-0.454678905261359,
1.7475));
#38272=CARTESIAN_POINT('Ctrl Pts',(-0.264547476698427,0.546151586166785,
0.650549949443909));
#38273=CARTESIAN_POINT('Ctrl Pts',(-0.355471695633361,0.502109284909664,
0.654524406148822));
#38274=CARTESIAN_POINT('Ctrl Pts',(-0.514804064846549,0.367775712187168,
0.662473319558649));
#38275=CARTESIAN_POINT('Ctrl Pts',(-0.628053036159548,0.0762413236404022,
0.674396689673389));
#38276=CARTESIAN_POINT('Ctrl Pts',(-0.587854166749295,-0.233845911034667,
0.68632005978813));
#38277=CARTESIAN_POINT('Ctrl Pts',(-0.404047259959307,-0.48683940429689,
0.698243429902869));
#38278=CARTESIAN_POINT('Ctrl Pts',(-0.121527158351189,-0.620878871458333,
0.710166800017609));
#38279=CARTESIAN_POINT('Ctrl Pts',(0.190680748588941,-0.603244694242624,
0.72209017013235));
#38280=CARTESIAN_POINT('Ctrl Pts',(0.456305609272025,-0.438231596848221,
0.734013540247088));
#38281=CARTESIAN_POINT('Ctrl Pts',(0.61045325274331,-0.166159471325954,
0.74593691036183));
#38282=CARTESIAN_POINT('Ctrl Pts',(0.615465575874622,0.146507028070995,
0.75786028047657));
#38283=CARTESIAN_POINT('Ctrl Pts',(0.470117741946454,0.423380863786649,
0.76978365059131));
#38284=CARTESIAN_POINT('Ctrl Pts',(0.209918811260263,0.596821791269607,
0.78170702070605));
#38285=CARTESIAN_POINT('Ctrl Pts',(-0.101563929551992,0.624457254778657,
0.79363039082079));
#38286=CARTESIAN_POINT('Ctrl Pts',(-0.388234290052265,0.499536043242417,
0.805553760935531));
#38287=CARTESIAN_POINT('Ctrl Pts',(-0.580057876616252,0.252576669093317,
0.817477131050269));
#38288=CARTESIAN_POINT('Ctrl Pts',(-0.63017161211444,-0.056087911206034,
0.829400501165011));
#38289=CARTESIAN_POINT('Ctrl Pts',(-0.526332568352355,-0.351050058657002,
0.841323871279751));
#38290=CARTESIAN_POINT('Ctrl Pts',(-0.293908927059336,-0.560249638256679,
0.85324724139449));
#38291=CARTESIAN_POINT('Ctrl Pts',(0.0103175303644349,-0.632578583371251,
0.865170611509231));
#38292=CARTESIAN_POINT('Ctrl Pts',(0.31202338494245,-0.550366716242752,
0.877093981623972));
#38293=CARTESIAN_POINT('Ctrl Pts',(0.537501007448335,-0.333698639877864,
0.889017351738711));
#38294=CARTESIAN_POINT('Ctrl Pts',(0.631665550747977,-0.0355070026353613,
0.900940721853452));
#38295=CARTESIAN_POINT('Ctrl Pts',(0.571512339483762,0.271359099787061,
0.912864091968191));
#38296=CARTESIAN_POINT('Ctrl Pts',(0.371736980381227,0.51193137495119,0.924787462082931));
#38297=CARTESIAN_POINT('Ctrl Pts',(0.0811451820615032,0.627437307350318,
0.936710832197672));
#38298=CARTESIAN_POINT('Ctrl Pts',(-0.229270623235126,0.589658457546506,
0.948634202312412));
#38299=CARTESIAN_POINT('Ctrl Pts',(-0.483674939990074,0.407824309791941,
0.960557572427152));
#38300=CARTESIAN_POINT('Ctrl Pts',(-0.619916044302459,0.12635748196595,
0.972480942541892));
#38301=CARTESIAN_POINT('Ctrl Pts',(-0.604709833109451,-0.185978850876312,
0.984404312656632));
#38302=CARTESIAN_POINT('Ctrl Pts',(-0.441771228592792,-0.452880002671609,
0.996327682771373));
#38303=CARTESIAN_POINT('Ctrl Pts',(-0.170906611750865,-0.6091412359152,
1.00825105288611));
#38304=CARTESIAN_POINT('Ctrl Pts',(0.141710993725228,-0.616587471077492,
1.02017442300085));
#38305=CARTESIAN_POINT('Ctrl Pts',(0.419708186042773,-0.473399570976854,
1.03209779311559));
#38306=CARTESIAN_POINT('Ctrl Pts',(0.595169432313768,-0.214558761349135,
1.04402116323033));
#38307=CARTESIAN_POINT('Ctrl Pts',(0.625229033275726,0.0966993856312912,
1.05594453334507));
#38308=CARTESIAN_POINT('Ctrl Pts',(0.502543339876973,0.384333587886446,
1.06786790345981));
#38309=CARTESIAN_POINT('Ctrl Pts',(0.257084828369703,0.578073962615934,
1.07979127357455));
#38310=CARTESIAN_POINT('Ctrl Pts',(-0.0511802639184789,0.630589165636079,
1.09171464368929));
#38311=CARTESIAN_POINT('Ctrl Pts',(-0.346941866986512,0.529049578172294,
1.10363801380403));
#38312=CARTESIAN_POINT('Ctrl Pts',(-0.557944550077233,0.298261620513743,
1.11556138391877));
#38313=CARTESIAN_POINT('Ctrl Pts',(-0.632639736230396,-0.00539252952743912,
1.12748475403351));
#38314=CARTESIAN_POINT('Ctrl Pts',(-0.552779171463751,-0.307729268722068,
1.13940812414825));
#38315=CARTESIAN_POINT('Ctrl Pts',(-0.337873026968778,-0.534886841191037,
1.15133149426299));
#38316=CARTESIAN_POINT('Ctrl Pts',(-0.0404235068239226,-0.631369982916851,
1.16325486437773));
#38317=CARTESIAN_POINT('Ctrl Pts',(0.26690159510024,-0.573607578197252,
1.17517823449247));
#38318=CARTESIAN_POINT('Ctrl Pts',(0.509021851217201,-0.375711152636948,
1.18710160460721));
#38319=CARTESIAN_POINT('Ctrl Pts',(0.626786569823609,-0.0860273858787084,
1.19902497472195));
#38320=CARTESIAN_POINT('Ctrl Pts',(0.591425483303132,0.224673124632266,
1.21094834483669));
#38321=CARTESIAN_POINT('Ctrl Pts',(0.411577409244242,0.480485329049876,
1.22287171495143));
#38322=CARTESIAN_POINT('Ctrl Pts',(0.131179761858824,0.618913552373053,
1.23479508506618));
#38323=CARTESIAN_POINT('Ctrl Pts',(-0.181265487721769,0.606139371921474,
1.24671845518091));
#38324=CARTESIAN_POINT('Ctrl Pts',(-0.449427044757826,0.445283557604159,
1.25864182529566));
#38325=CARTESIAN_POINT('Ctrl Pts',(-0.607792251030169,0.175643658638878,
1.2705651954104));
#38326=CARTESIAN_POINT('Ctrl Pts',(-0.617672020202178,-0.136906503467616,
1.28248856552514));
#38327=CARTESIAN_POINT('Ctrl Pts',(-0.476652695565553,-0.416010003536527,
1.29441193563987));
#38328=CARTESIAN_POINT('Ctrl Pts',(-0.219185713483245,-0.593481034437674,
1.30633530575462));
#38329=CARTESIAN_POINT('Ctrl Pts',(0.0918289839862619,-0.625962900603877,
1.31825867586936));
#38330=CARTESIAN_POINT('Ctrl Pts',(0.380409590197501,-0.505520186459593,
1.3301820459841));
#38331=CARTESIAN_POINT('Ctrl Pts',(0.576055013076121,-0.26157740181873,
1.34210541609884));
#38332=CARTESIAN_POINT('Ctrl Pts',(0.630968499564522,0.0462695125289182,
1.35402878621358));
#38333=CARTESIAN_POINT('Ctrl Pts',(0.531734523173002,0.34281264868491,1.36595215632832));
#38334=CARTESIAN_POINT('Ctrl Pts',(0.302596236614874,0.555605645056675,
1.37787552644306));
#38335=CARTESIAN_POINT('Ctrl Pts',(-0.000467201806429895,0.632662545876497,
1.3897988965578));
#38336=CARTESIAN_POINT('Ctrl Pts',(-0.303416501450367,0.555158123312486,
1.40172226667254));
#38337=CARTESIAN_POINT('Ctrl Pts',(-0.532240256115767,0.3420269360772,1.41364563678728));
#38338=CARTESIAN_POINT('Ctrl Pts',(-0.631036148567181,0.0453375609608587,
1.42556900690202));
#38339=CARTESIAN_POINT('Ctrl Pts',(-0.575668051287862,-0.262427913831801,
1.43749237701676));
#38340=CARTESIAN_POINT('Ctrl Pts',(-0.379662553523367,-0.506081476332481,
1.4494157471315));
#38341=CARTESIAN_POINT('Ctrl Pts',(-0.0909043756851951,-0.626097843558096,
1.46133911724624));
#38342=CARTESIAN_POINT('Ctrl Pts',(0.220062008878289,-0.593156663530657,
1.47326248736098));
#38343=CARTESIAN_POINT('Ctrl Pts',(0.477266596511919,-0.415305563499184,
1.48518585747572));
#38344=CARTESIAN_POINT('Ctrl Pts',(0.617873548883792,-0.135994091149731,
1.49710922759046));
#38345=CARTESIAN_POINT('Ctrl Pts',(0.607532173409899,0.176541138367681,
1.5090325977052));
#38346=CARTESIAN_POINT('Ctrl Pts',(0.44876889853771,0.445946847509907,1.52095596781994));
#38347=CARTESIAN_POINT('Ctrl Pts',(0.180370060014882,0.606406428909711,
1.53287933793468));
#38348=CARTESIAN_POINT('Ctrl Pts',(-0.132093715531906,0.618719132473601,
1.54480270804942));
#38349=CARTESIAN_POINT('Ctrl Pts',(-0.412286607098983,0.479876931929719,
1.55672607816416));
#38350=CARTESIAN_POINT('Ctrl Pts',(-0.591756666633523,0.223799378893573,
1.5686494482789));
#38351=CARTESIAN_POINT('Ctrl Pts',(-0.626658828732613,-0.0869530124049729,
1.58057281839364));
#38352=CARTESIAN_POINT('Ctrl Pts',(-0.508466394890466,-0.376462544933448,
1.59249618850838));
#38353=CARTESIAN_POINT('Ctrl Pts',(-0.266054119846729,-0.574001132528779,
1.60441955862312));
#38354=CARTESIAN_POINT('Ctrl Pts',(0.041355953716283,-0.631309625261172,
1.61634292873786));
#38355=CARTESIAN_POINT('Ctrl Pts',(0.338662659096756,-0.534387172794291,
1.6282662988526));
#38356=CARTESIAN_POINT('Ctrl Pts',(0.553233053245814,-0.306912647437654,
1.64018966896734));
#38357=CARTESIAN_POINT('Ctrl Pts',(0.63264703504302,-0.004457885988231,
1.65211303908208));
#38358=CARTESIAN_POINT('Ctrl Pts',(0.557503379173826,0.299084810277989,
1.66403640919682));
#38359=CARTESIAN_POINT('Ctrl Pts',(0.346160212094308,0.529562476556959,
1.67595977931156));
#38360=CARTESIAN_POINT('Ctrl Pts',(0.0502486745876001,0.630661949020613,
1.6878831494263));
#38361=CARTESIAN_POINT('Ctrl Pts',(-0.257937943046404,0.577697854759531,
1.69980651954104));
#38362=CARTESIAN_POINT('Ctrl Pts',(-0.503111198644335,0.383582524720304,
1.71172988965578));
#38363=CARTESIAN_POINT('Ctrl Pts',(-0.625369568828046,0.09579278701182,
1.72365325977052));
#38364=CARTESIAN_POINT('Ctrl Pts',(-0.594855848719033,-0.215473244051477,
1.73557662988526));
#38365=CARTESIAN_POINT('Ctrl Pts',(-0.477608641113037,-0.38776777370368,
1.74352554329509));
#38366=CARTESIAN_POINT('Ctrl Pts',(-0.401912945313201,-0.454678905261359,
1.7475));
#38367=CARTESIAN_POINT('Ctrl Pts',(-0.276993436094884,0.571845955096606,
0.667033299629272));
#38368=CARTESIAN_POINT('Ctrl Pts',(-0.372195296045872,0.525731629944139,
0.671007756334186));
#38369=CARTESIAN_POINT('Ctrl Pts',(-0.539023651319926,0.385078170097597,
0.678956669744013));
#38370=CARTESIAN_POINT('Ctrl Pts',(-0.657600558912049,0.0798281899004894,
0.690880039858753));
#38371=CARTESIAN_POINT('Ctrl Pts',(-0.615510484555496,-0.244847477748088,
0.702803409973493));
#38372=CARTESIAN_POINT('Ctrl Pts',(-0.423056157169224,-0.509743359133631,
0.714726780088233));
#38373=CARTESIAN_POINT('Ctrl Pts',(-0.127244552057915,-0.650088876863516,
0.726650150202973));
#38374=CARTESIAN_POINT('Ctrl Pts',(0.199651557474521,-0.63162507822652,
0.738573520317714));
#38375=CARTESIAN_POINT('Ctrl Pts',(0.477773064400501,-0.458848737970438,
0.750496890432453));
#38376=CARTESIAN_POINT('Ctrl Pts',(0.639172772172858,-0.173976646750452,
0.762420260547194));
#38377=CARTESIAN_POINT('Ctrl Pts',(0.644420906172423,0.153399630281469,
0.774343630661934));
#38378=CARTESIAN_POINT('Ctrl Pts',(0.492235005739107,0.443299334019999,
0.786267000776673));
#38379=CARTESIAN_POINT('Ctrl Pts',(0.219794698318813,0.624900001932452,
0.798190370891413));
#38380=CARTESIAN_POINT('Ctrl Pts',(-0.106342128758895,0.653835609600986,
0.810113741006155));
#38381=CARTESIAN_POINT('Ctrl Pts',(-0.406499246764783,0.523037326977394,
0.822037111120894));
#38382=CARTESIAN_POINT('Ctrl Pts',(-0.607347408423773,0.264459447214129,
0.833960481235634));
#38383=CARTESIAN_POINT('Ctrl Pts',(-0.659818805862263,-0.0587266355447204,
0.845883851350374));
#38384=CARTESIAN_POINT('Ctrl Pts',(-0.5510945273644,-0.367565637753413,
0.857807221465114));
#38385=CARTESIAN_POINT('Ctrl Pts',(-0.30773623177639,-0.586607267279053,
0.869730591579855));
#38386=CARTESIAN_POINT('Ctrl Pts',(0.0108029311914999,-0.662339016023882,
0.881653961694595));
#38387=CARTESIAN_POINT('Ctrl Pts',(0.326702906471833,-0.576259391119132,
0.893577331809334));
#38388=CARTESIAN_POINT('Ctrl Pts',(0.562788399328783,-0.349397900269251,
0.905500701924076));
#38389=CARTESIAN_POINT('Ctrl Pts',(0.661383028664851,-0.0371774729743906,
0.917424072038814));
#38390=CARTESIAN_POINT('Ctrl Pts',(0.598399836051714,0.284125520317538,
0.929347442153556));
#38391=CARTESIAN_POINT('Ctrl Pts',(0.389225800995687,0.536015812217164,
0.941270812268294));
#38392=CARTESIAN_POINT('Ctrl Pts',(0.0849627563349745,0.656955862388386,
0.953194182383036));
#38393=CARTESIAN_POINT('Ctrl Pts',(-0.240056939941664,0.617399660418637,
0.965117552497775));
#38394=CARTESIAN_POINT('Ctrl Pts',(-0.50643001873559,0.427010902927905,
0.977040922612516));
#38395=CARTESIAN_POINT('Ctrl Pts',(-0.649080752327234,0.132302124151215,
0.988964292727255));
#38396=CARTESIAN_POINT('Ctrl Pts',(-0.633159146342169,-0.194728453236893,
1.000887662842));
#38397=CARTESIAN_POINT('Ctrl Pts',(-0.462554896016907,-0.474186295950466,
1.01281103295674));
#38398=CARTESIAN_POINT('Ctrl Pts',(-0.178947122199061,-0.637799029909398,
1.02473440307148));
#38399=CARTESIAN_POINT('Ctrl Pts',(0.148377960637735,-0.645595582306399,
1.03665777318622));
#38400=CARTESIAN_POINT('Ctrl Pts',(0.439453870662564,-0.495671232427607,
1.04858114330096));
#38401=CARTESIAN_POINT('Ctrl Pts',(0.623169905729864,-0.224652940531005,
1.0605045134157));
#38402=CARTESIAN_POINT('Ctrl Pts',(0.654643697360791,0.101248726423535,
1.07242788353044));
#38403=CARTESIAN_POINT('Ctrl Pts',(0.526186105557929,0.402415031297763,
1.08435125364518));
#38404=CARTESIAN_POINT('Ctrl Pts',(0.269179698353975,0.605270158764381,
1.09627462375992));
#38405=CARTESIAN_POINT('Ctrl Pts',(-0.0535881019919275,0.660256003699702,
1.10819799387466));
#38406=CARTESIAN_POINT('Ctrl Pts',(-0.363264171184361,0.553939362232308,
1.1201213639894));
#38407=CARTESIAN_POINT('Ctrl Pts',(-0.584193733408707,0.312293703014637,
1.13204473410414));
#38408=CARTESIAN_POINT('Ctrl Pts',(-0.662403045894032,-0.00564622767032119,
1.14396810421888));
#38409=CARTESIAN_POINT('Ctrl Pts',(-0.578785343244735,-0.322206768305185,
1.15589147433362));
#38410=CARTESIAN_POINT('Ctrl Pts',(-0.353768676503191,-0.560051246424626,
1.16781484444836));
#38411=CARTESIAN_POINT('Ctrl Pts',(-0.042325280111924,-0.661073555483839,
1.1797382145631));
#38412=CARTESIAN_POINT('Ctrl Pts',(0.279458306874339,-0.600593647831481,
1.19166158467784));
#38413=CARTESIAN_POINT('Ctrl Pts',(0.532969406382811,-0.393386943042789,
1.20358495479258));
#38414=CARTESIAN_POINT('Ctrl Pts',(0.656274510119339,-0.0900746493982562,
1.21550832490732));
#38415=CARTESIAN_POINT('Ctrl Pts',(0.619249818061811,0.235243146397531,
1.22743169502206));
#38416=CARTESIAN_POINT('Ctrl Pts',(0.430940571531337,0.503090348650062,
1.2393550651368));
#38417=CARTESIAN_POINT('Ctrl Pts',(0.1373512740959,0.648031096939669,1.25127843525154));
#38418=CARTESIAN_POINT('Ctrl Pts',(-0.189793344151622,0.634655939554922,
1.26320180536628));
#38419=CARTESIAN_POINT('Ctrl Pts',(-0.470570889411094,0.466232466839719,
1.27512517548102));
#38420=CARTESIAN_POINT('Ctrl Pts',(-0.636386580381591,0.183907029247991,
1.28704854559576));
#38421=CARTESIAN_POINT('Ctrl Pts',(-0.646731155370297,-0.143347437263448,
1.2989719157105));
#38422=CARTESIAN_POINT('Ctrl Pts',(-0.49907740423886,-0.435581702640041,
1.31089528582524));
#38423=CARTESIAN_POINT('Ctrl Pts',(-0.229497573283767,-0.621402075111968,
1.32281865593998));
#38424=CARTESIAN_POINT('Ctrl Pts',(0.0961491907800454,-0.655412090374398,
1.33474202605472));
#38425=CARTESIAN_POINT('Ctrl Pts',(0.398306424341256,-0.529303001526613,
1.34666539616946));
#38426=CARTESIAN_POINT('Ctrl Pts',(0.603156225275714,-0.273883630412164,
1.3585887662842));
#38427=CARTESIAN_POINT('Ctrl Pts',(0.660653183856468,0.0484463183008557,
1.37051213639894));
#38428=CARTESIAN_POINT('Ctrl Pts',(0.556750623752369,0.358940688760636,
1.38243550651368));
#38429=CARTESIAN_POINT('Ctrl Pts',(0.316832246428428,0.581744791742624,
1.39435887662842));
#38430=CARTESIAN_POINT('Ctrl Pts',(-0.000489181886471275,0.662426928647814,
1.40628224674316));
#38431=CARTESIAN_POINT('Ctrl Pts',(-0.317691101625711,0.581276215790976,
1.4182056168579));
#38432=CARTESIAN_POINT('Ctrl Pts',(-0.557280149519581,0.358118011342924,
1.43012898697264));
#38433=CARTESIAN_POINT('Ctrl Pts',(-0.660724015489144,0.0474705219321574,
1.44205235708738));
#38434=CARTESIAN_POINT('Ctrl Pts',(-0.602751058397144,-0.274774155802465,
1.45397572720212));
#38435=CARTESIAN_POINT('Ctrl Pts',(-0.39752424241369,-0.529890697967634,
1.46589909731686));
#38436=CARTESIAN_POINT('Ctrl Pts',(-0.0951810831513113,-0.655553381884837,
1.4778224674316));
#38437=CARTESIAN_POINT('Ctrl Pts',(0.230415095066762,-0.621062443779154,
1.48974583754634));
#38438=CARTESIAN_POINT('Ctrl Pts',(0.499720186905616,-0.434844121360108,
1.50166920766108));
#38439=CARTESIAN_POINT('Ctrl Pts',(0.646942165215064,-0.142392099392831,
1.51359257777582));
#38440=CARTESIAN_POINT('Ctrl Pts',(0.636114267091785,0.18484673200762,1.52551594789056));
#38441=CARTESIAN_POINT('Ctrl Pts',(0.469881779897605,0.466926962029817,
1.5374393180053));
#38442=CARTESIAN_POINT('Ctrl Pts',(0.188855789953788,0.634935560565594,
1.54936268812004));
#38443=CARTESIAN_POINT('Ctrl Pts',(-0.138308225836652,0.647827530318408,
1.56128605823478));
#38444=CARTESIAN_POINT('Ctrl Pts',(-0.431683134466003,0.502453328743748,
1.57320942834952));
#38445=CARTESIAN_POINT('Ctrl Pts',(-0.619596582316783,0.234328294222587,
1.58513279846426));
#38446=CARTESIAN_POINT('Ctrl Pts',(-0.656140759292581,-0.0910438231558368,
1.597056168579));
#38447=CARTESIAN_POINT('Ctrl Pts',(-0.532387817934254,-0.394173685508301,
1.60897953869374));
#38448=CARTESIAN_POINT('Ctrl Pts',(-0.278570961111662,-0.601005717407574,
1.62090290880848));
#38449=CARTESIAN_POINT('Ctrl Pts',(0.0433015951080595,-0.661010358228473,
1.63282627892322));
#38450=CARTESIAN_POINT('Ctrl Pts',(0.354595457839793,-0.559528070517414,
1.64474964903796));
#38451=CARTESIAN_POINT('Ctrl Pts',(0.579260578450012,-0.321351728074295,
1.6566730191527));
#38452=CARTESIAN_POINT('Ctrl Pts',(0.662410688088217,-0.00466761268340117,
1.66859638926744));
#38453=CARTESIAN_POINT('Ctrl Pts',(0.583731807080909,0.313155620747522,
1.68051975938218));
#38454=CARTESIAN_POINT('Ctrl Pts',(0.362445742382341,0.554476390548393,
1.69244312949692));
#38455=CARTESIAN_POINT('Ctrl Pts',(0.0526126849023013,0.660332211267524,
1.70436649961166));
#38456=CARTESIAN_POINT('Ctrl Pts',(-0.270072948853399,0.604876356454159,
1.7162898697264));
#38457=CARTESIAN_POINT('Ctrl Pts',(-0.526780679935092,0.401628633446949,
1.72821323984114));
#38458=CARTESIAN_POINT('Ctrl Pts',(-0.654790844579946,0.10029947576388,
1.74013660995588));
#38459=CARTESIAN_POINT('Ctrl Pts',(-0.622841569211623,-0.225610446189846,
1.75205998007062));
#38460=CARTESIAN_POINT('Ctrl Pts',(-0.500078323413074,-0.406010782584359,
1.76000889348045));
#38461=CARTESIAN_POINT('Ctrl Pts',(-0.420821431081829,-0.476069830111341,
1.76398335018536));
#38462=CARTESIAN_POINT('Ctrl Pts',(-0.289439395491341,0.597540324026427,
0.683516649814636));
#38463=CARTESIAN_POINT('Ctrl Pts',(-0.388918896458382,0.549353974978614,
0.68749110651955));
#38464=CARTESIAN_POINT('Ctrl Pts',(-0.563243237793303,0.402380628008027,
0.695440019929377));
#38465=CARTESIAN_POINT('Ctrl Pts',(-0.687148081664549,0.0834150561605762,
0.707363390044116));
#38466=CARTESIAN_POINT('Ctrl Pts',(-0.643166802361696,-0.255849044461509,
0.719286760158857));
#38467=CARTESIAN_POINT('Ctrl Pts',(-0.442065054379141,-0.532647313970372,
0.731210130273597));
#38468=CARTESIAN_POINT('Ctrl Pts',(-0.132961945764642,-0.679298882268699,
0.743133500388337));
#38469=CARTESIAN_POINT('Ctrl Pts',(0.208622366360101,-0.660005462210415,
0.755056870503077));
#38470=CARTESIAN_POINT('Ctrl Pts',(0.499240519528978,-0.479465879092654,
0.766980240617817));
#38471=CARTESIAN_POINT('Ctrl Pts',(0.667892291602407,-0.181793822174949,
0.778903610732558));
#38472=CARTESIAN_POINT('Ctrl Pts',(0.673376236470223,0.160292232491944,
0.790826980847297));
#38473=CARTESIAN_POINT('Ctrl Pts',(0.51435226953176,0.463217804253349,0.802750350962038));
#38474=CARTESIAN_POINT('Ctrl Pts',(0.229670585377363,0.652978212595296,
0.814673721076777));
#38475=CARTESIAN_POINT('Ctrl Pts',(-0.111120327965797,0.683213964423316,
0.826597091191518));
#38476=CARTESIAN_POINT('Ctrl Pts',(-0.424764203477302,0.546538610712372,
0.838520461306258));
#38477=CARTESIAN_POINT('Ctrl Pts',(-0.634636940231293,0.27634222533494,
0.850443831420998));
#38478=CARTESIAN_POINT('Ctrl Pts',(-0.689465999610088,-0.0613653598834067,
0.862367201535738));
#38479=CARTESIAN_POINT('Ctrl Pts',(-0.575856486376446,-0.384081216849825,
0.874290571650478));
#38480=CARTESIAN_POINT('Ctrl Pts',(-0.321563536493444,-0.612964896301427,
0.886213941765218));
#38481=CARTESIAN_POINT('Ctrl Pts',(0.0112883320185645,-0.692099448676514,
0.898137311879959));
#38482=CARTESIAN_POINT('Ctrl Pts',(0.341382428001217,-0.602152065995511,
0.910060681994698));
#38483=CARTESIAN_POINT('Ctrl Pts',(0.58807579120923,-0.365097160660638,
0.921984052109439));
#38484=CARTESIAN_POINT('Ctrl Pts',(0.691100506581725,-0.0388479433134198,
0.933907422224178));
#38485=CARTESIAN_POINT('Ctrl Pts',(0.625287332619665,0.296891940848016,
0.94583079233892));
#38486=CARTESIAN_POINT('Ctrl Pts',(0.406714621610146,0.560100249483138,
0.957754162453659));
#38487=CARTESIAN_POINT('Ctrl Pts',(0.0887803306084458,0.686474417426454,
0.969677532568399));
#38488=CARTESIAN_POINT('Ctrl Pts',(-0.250843256648201,0.645140863290769,
0.98160090268314));
#38489=CARTESIAN_POINT('Ctrl Pts',(-0.529185097481107,0.44619749606387,
0.993524272797879));
#38490=CARTESIAN_POINT('Ctrl Pts',(-0.678245460352009,0.13824676633648,
1.00544764291262));
#38491=CARTESIAN_POINT('Ctrl Pts',(-0.661608459574888,-0.203478055597473,
1.01737101302736));
#38492=CARTESIAN_POINT('Ctrl Pts',(-0.483338563441022,-0.495492589229323,
1.0292943831421));
#38493=CARTESIAN_POINT('Ctrl Pts',(-0.186987632647257,-0.666456823903595,
1.04121775325684));
#38494=CARTESIAN_POINT('Ctrl Pts',(0.155044927550243,-0.674603693535307,
1.05314112337158));
#38495=CARTESIAN_POINT('Ctrl Pts',(0.459199555282356,-0.517942893878359,
1.06506449348632));
#38496=CARTESIAN_POINT('Ctrl Pts',(0.651170379145961,-0.234747119712876,
1.07698786360106));
#38497=CARTESIAN_POINT('Ctrl Pts',(0.684058361445857,0.105798067215779,
1.0889112337158));
#38498=CARTESIAN_POINT('Ctrl Pts',(0.549828871238885,0.420496474709079,
1.10083460383054));
#38499=CARTESIAN_POINT('Ctrl Pts',(0.281274568338247,0.632466354912828,
1.11275797394528));
#38500=CARTESIAN_POINT('Ctrl Pts',(-0.0559959400653758,0.689922841763325,
1.12468134406002));
#38501=CARTESIAN_POINT('Ctrl Pts',(-0.37958647538221,0.578829146292321,
1.13660471417476));
#38502=CARTESIAN_POINT('Ctrl Pts',(-0.61044291674018,0.326325785515531,
1.1485280842895));
#38503=CARTESIAN_POINT('Ctrl Pts',(-0.692166355557669,-0.00589992581320304,
1.16045145440424));
#38504=CARTESIAN_POINT('Ctrl Pts',(-0.60479151502572,-0.336684267888303,
1.17237482451898));
#38505=CARTESIAN_POINT('Ctrl Pts',(-0.369664326037605,-0.585215651658216,
1.18429819463372));
#38506=CARTESIAN_POINT('Ctrl Pts',(-0.0442270533999247,-0.690777128050826,
1.19622156474846));
#38507=CARTESIAN_POINT('Ctrl Pts',(0.292015018648436,-0.62757971746571,
1.2081449348632));
#38508=CARTESIAN_POINT('Ctrl Pts',(0.556916961548422,-0.411062733448631,
1.22006830497794));
#38509=CARTESIAN_POINT('Ctrl Pts',(0.68576245041507,-0.0941219129178041,
1.23199167509268));
#38510=CARTESIAN_POINT('Ctrl Pts',(0.647074152820491,0.245813168162796,
1.24391504520742));
#38511=CARTESIAN_POINT('Ctrl Pts',(0.450303733818432,0.52569536825025,1.25583841532216));
#38512=CARTESIAN_POINT('Ctrl Pts',(0.143522786332977,0.677148641506285,
1.2677617854369));
#38513=CARTESIAN_POINT('Ctrl Pts',(-0.198321200581474,0.66317250718837,
1.27968515555164));
#38514=CARTESIAN_POINT('Ctrl Pts',(-0.491714734064362,0.487181376075277,
1.29160852566638));
#38515=CARTESIAN_POINT('Ctrl Pts',(-0.664980909733015,0.192170399857104,
1.30353189578112));
#38516=CARTESIAN_POINT('Ctrl Pts',(-0.675790290538415,-0.149788371059279,
1.31545526589586));
#38517=CARTESIAN_POINT('Ctrl Pts',(-0.521502112912168,-0.455153401743555,
1.3273786360106));
#38518=CARTESIAN_POINT('Ctrl Pts',(-0.23980943308429,-0.649323115786262,
1.33930200612534));
#38519=CARTESIAN_POINT('Ctrl Pts',(0.100469397573829,-0.684861280144919,
1.35122537624008));
#38520=CARTESIAN_POINT('Ctrl Pts',(0.416203258485012,-0.553085816593635,
1.36314874635482));
#38521=CARTESIAN_POINT('Ctrl Pts',(0.630257437475308,-0.286189859005598,
1.37507211646956));
#38522=CARTESIAN_POINT('Ctrl Pts',(0.690337868148412,0.050623124072793,
1.3869954865843));
#38523=CARTESIAN_POINT('Ctrl Pts',(0.581766724331738,0.375068728836361,
1.39891885669904));
#38524=CARTESIAN_POINT('Ctrl Pts',(0.33106825624198,0.607883938428571,1.41084222681378));
#38525=CARTESIAN_POINT('Ctrl Pts',(-0.000511161966512498,0.692191311419132,
1.42276559692852));
#38526=CARTESIAN_POINT('Ctrl Pts',(-0.331965701801056,0.607394308269466,
1.43468896704327));
#38527=CARTESIAN_POINT('Ctrl Pts',(-0.582320042923395,0.374209086608647,
1.446612337158));
#38528=CARTESIAN_POINT('Ctrl Pts',(-0.690411882411108,0.0496034829034569,
1.45853570727274));
#38529=CARTESIAN_POINT('Ctrl Pts',(-0.629834065506428,-0.287120397773129,
1.47045907738748));
#38530=CARTESIAN_POINT('Ctrl Pts',(-0.415385931304013,-0.553699919602786,
1.48238244750222));
#38531=CARTESIAN_POINT('Ctrl Pts',(-0.0994577906174278,-0.68500892021158,
1.49430581761697));
#38532=CARTESIAN_POINT('Ctrl Pts',(0.240768181255235,-0.648968224027652,
1.5062291877317));
#38533=CARTESIAN_POINT('Ctrl Pts',(0.522173777299313,-0.454382679221032,
1.51815255784645));
#38534=CARTESIAN_POINT('Ctrl Pts',(0.676010781546336,-0.148790107635931,
1.53007592796118));
#38535=CARTESIAN_POINT('Ctrl Pts',(0.664696360773671,0.193152325647559,
1.54199929807593));
#38536=CARTESIAN_POINT('Ctrl Pts',(0.490994661257499,0.487907076549728,
1.55392266819067));
#38537=CARTESIAN_POINT('Ctrl Pts',(0.197341519892694,0.663464692221476,
1.56584603830541));
#38538=CARTESIAN_POINT('Ctrl Pts',(-0.144522736141398,0.676935928163215,
1.57776940842015));
#38539=CARTESIAN_POINT('Ctrl Pts',(-0.451079661833022,0.525029725557777,
1.58969277853489));
#38540=CARTESIAN_POINT('Ctrl Pts',(-0.647436498000044,0.2448572095516,1.60161614864963));
#38541=CARTESIAN_POINT('Ctrl Pts',(-0.685622689852549,-0.0951346339067004,
1.61353951876436));
#38542=CARTESIAN_POINT('Ctrl Pts',(-0.556309240978042,-0.411884826083155,
1.62546288887911));
#38543=CARTESIAN_POINT('Ctrl Pts',(-0.291087802376595,-0.628010302286368,
1.63738625899384));
#38544=CARTESIAN_POINT('Ctrl Pts',(0.0452472364998361,-0.690711091195774,
1.64930962910859));
#38545=CARTESIAN_POINT('Ctrl Pts',(0.37052825658283,-0.584668968240537,
1.66123299922332));
#38546=CARTESIAN_POINT('Ctrl Pts',(0.605288103654211,-0.335790808710935,
1.67315636933807));
#38547=CARTESIAN_POINT('Ctrl Pts',(0.692174341133415,-0.00487733937857217,
1.6850797394528));
#38548=CARTESIAN_POINT('Ctrl Pts',(0.609960234987991,0.327226431217055,
1.69700310956755));
#38549=CARTESIAN_POINT('Ctrl Pts',(0.378731272670374,0.579390304539825,
1.70892647968229));
#38550=CARTESIAN_POINT('Ctrl Pts',(0.0549766952170021,0.690002473514437,
1.72084984979703));
#38551=CARTESIAN_POINT('Ctrl Pts',(-0.282207954660393,0.632054858148786,
1.73277321991177));
#38552=CARTESIAN_POINT('Ctrl Pts',(-0.550450161225849,0.419674742173595,
1.74469659002651));
#38553=CARTESIAN_POINT('Ctrl Pts',(-0.684212120331845,0.104806164515941,
1.75661996014125));
#38554=CARTESIAN_POINT('Ctrl Pts',(-0.650827289704214,-0.235747648328215,
1.76854333025599));
#38555=CARTESIAN_POINT('Ctrl Pts',(-0.522548005713111,-0.424253791465037,
1.77649224366581));
#38556=CARTESIAN_POINT('Ctrl Pts',(-0.439729916850458,-0.497460754961323,
1.78046670037073));
#38557=CARTESIAN_POINT('Ctrl Pts',(-0.301885354887798,0.623234692956248,
0.7));
#38558=CARTESIAN_POINT('Ctrl Pts',(-0.405642496870893,0.572976320013089,
0.703974456704914));
#38559=CARTESIAN_POINT('Ctrl Pts',(-0.58746282426668,0.419683085918456,
0.711923370114741));
#38560=CARTESIAN_POINT('Ctrl Pts',(-0.71669560441705,0.0870019224206636,
0.72384674022948));
#38561=CARTESIAN_POINT('Ctrl Pts',(-0.670823120167895,-0.26685061117493,
0.735770110344222));
#38562=CARTESIAN_POINT('Ctrl Pts',(-0.461073951589059,-0.555551268807112,
0.747693480458959));
#38563=CARTESIAN_POINT('Ctrl Pts',(-0.138679339471368,-0.708508887673882,
0.759616850573702));
#38564=CARTESIAN_POINT('Ctrl Pts',(0.21759317524568,-0.688385846194311,
0.77154022068844));
#38565=CARTESIAN_POINT('Ctrl Pts',(0.520707974657454,-0.50008302021487,
0.783463590803181));
#38566=CARTESIAN_POINT('Ctrl Pts',(0.696611811031955,-0.189610997599447,
0.795386960917921));
#38567=CARTESIAN_POINT('Ctrl Pts',(0.702331566768025,0.167184834702419,
0.807310331032661));
#38568=CARTESIAN_POINT('Ctrl Pts',(0.536469533324413,0.483136274486699,
0.819233701147402));
#38569=CARTESIAN_POINT('Ctrl Pts',(0.239546472435912,0.681056423258141,
0.831157071262141));
#38570=CARTESIAN_POINT('Ctrl Pts',(-0.1158985271727,0.712592319245645,0.843080441376882));
#38571=CARTESIAN_POINT('Ctrl Pts',(-0.443029160189821,0.57003989444735,
0.855003811491621));
#38572=CARTESIAN_POINT('Ctrl Pts',(-0.661926472038813,0.288225003455751,
0.866927181606362));
#38573=CARTESIAN_POINT('Ctrl Pts',(-0.719113193357913,-0.0640040842220929,
0.878850551721102));
#38574=CARTESIAN_POINT('Ctrl Pts',(-0.600618445388491,-0.400596795946236,
0.890773921835841));
#38575=CARTESIAN_POINT('Ctrl Pts',(-0.335390841210499,-0.639322525323802,
0.902697291950582));
#38576=CARTESIAN_POINT('Ctrl Pts',(0.0117737328456294,-0.721859881329144,
0.914620662065322));
#38577=CARTESIAN_POINT('Ctrl Pts',(0.356061949530601,-0.62804474087189,
0.926544032180063));
#38578=CARTESIAN_POINT('Ctrl Pts',(0.613363183089679,-0.380796421052026,
0.938467402294802));
#38579=CARTESIAN_POINT('Ctrl Pts',(0.720817984498598,-0.0405184136524491,
0.950390772409543));
#38580=CARTESIAN_POINT('Ctrl Pts',(0.652174829187617,0.309658361378493,
0.962314142524283));
#38581=CARTESIAN_POINT('Ctrl Pts',(0.424203442224605,0.584184686749112,
0.974237512639022));
#38582=CARTESIAN_POINT('Ctrl Pts',(0.0925979048819177,0.715992972464522,
0.986160882753764));
#38583=CARTESIAN_POINT('Ctrl Pts',(-0.26162957335474,0.672882066162899,
0.998084252868503));
#38584=CARTESIAN_POINT('Ctrl Pts',(-0.551940176226622,0.465384089199835,
1.01000762298324));
#38585=CARTESIAN_POINT('Ctrl Pts',(-0.707410168376785,0.144191408521745,
1.02193099309798));
#38586=CARTESIAN_POINT('Ctrl Pts',(-0.690057772807605,-0.212227657958053,
1.03385436321272));
#38587=CARTESIAN_POINT('Ctrl Pts',(-0.504122230865138,-0.51679888250818,
1.04577773332746));
#38588=CARTESIAN_POINT('Ctrl Pts',(-0.195028143095452,-0.695114617897793,
1.0577011034422));
#38589=CARTESIAN_POINT('Ctrl Pts',(0.161711894462749,-0.703611804764214,
1.06962447355694));
#38590=CARTESIAN_POINT('Ctrl Pts',(0.478945239902149,-0.540214555329112,
1.08154784367168));
#38591=CARTESIAN_POINT('Ctrl Pts',(0.679170852562056,-0.244841298894746,
1.09347121378642));
#38592=CARTESIAN_POINT('Ctrl Pts',(0.713473025530922,0.110347408008022,
1.10539458390116));
#38593=CARTESIAN_POINT('Ctrl Pts',(0.57347163691984,0.438577918120396,1.1173179540159));
#38594=CARTESIAN_POINT('Ctrl Pts',(0.293369438322519,0.659662551061274,
1.12924132413064));
#38595=CARTESIAN_POINT('Ctrl Pts',(-0.0584037781388241,0.719589679826949,
1.14116469424538));
#38596=CARTESIAN_POINT('Ctrl Pts',(-0.395908779580059,0.603718930352334,
1.15308806436013));
#38597=CARTESIAN_POINT('Ctrl Pts',(-0.636692100071654,0.340357868016426,
1.16501143447486));
#38598=CARTESIAN_POINT('Ctrl Pts',(-0.721929665221305,-0.00615362395608558,
1.17693480458961));
#38599=CARTESIAN_POINT('Ctrl Pts',(-0.630797686806703,-0.35116176747142,
1.18885817470434));
#38600=CARTESIAN_POINT('Ctrl Pts',(-0.385559975572019,-0.610380056891805,
1.20078154481909));
#38601=CARTESIAN_POINT('Ctrl Pts',(-0.0461288266879255,-0.720480700617813,
1.21270491493383));
#38602=CARTESIAN_POINT('Ctrl Pts',(0.304571730422535,-0.654565787099938,
1.22462828504857));
#38603=CARTESIAN_POINT('Ctrl Pts',(0.580864516714032,-0.428738523854473,
1.2365516551633));
#38604=CARTESIAN_POINT('Ctrl Pts',(0.7152503907108,-0.0981691764373513,
1.24847502527805));
#38605=CARTESIAN_POINT('Ctrl Pts',(0.674898487579171,0.25638318992806,1.26039839539278));
#38606=CARTESIAN_POINT('Ctrl Pts',(0.469666896105526,0.548300387850438,
1.27232176550753));
#38607=CARTESIAN_POINT('Ctrl Pts',(0.149694298570053,0.706266186072899,
1.28424513562226));
#38608=CARTESIAN_POINT('Ctrl Pts',(-0.206849057011327,0.691689074821819,
1.29616850573701));
#38609=CARTESIAN_POINT('Ctrl Pts',(-0.51285857871763,0.508130285310836,
1.30809187585175));
#38610=CARTESIAN_POINT('Ctrl Pts',(-0.693575239084438,0.200433770466217,
1.32001524596649));
#38611=CARTESIAN_POINT('Ctrl Pts',(-0.704849425706532,-0.15622930485511,
1.33193861608123));
#38612=CARTESIAN_POINT('Ctrl Pts',(-0.543926821585475,-0.474725100847069,
1.34386198619597));
#38613=CARTESIAN_POINT('Ctrl Pts',(-0.250121292884812,-0.677244156460556,
1.35578535631071));
#38614=CARTESIAN_POINT('Ctrl Pts',(0.104789604367612,-0.71431046991544,
1.36770872642545));
#38615=CARTESIAN_POINT('Ctrl Pts',(0.434100092628769,-0.576868631660655,
1.37963209654019));
#38616=CARTESIAN_POINT('Ctrl Pts',(0.6573586496749,-0.298496087599031,1.39155546665493));
#38617=CARTESIAN_POINT('Ctrl Pts',(0.720022552440358,0.0527999298447306,
1.40347883676967));
#38618=CARTESIAN_POINT('Ctrl Pts',(0.606782824911105,0.391196768912086,
1.41540220688441));
#38619=CARTESIAN_POINT('Ctrl Pts',(0.345304266055534,0.634023085114521,
1.42732557699915));
#38620=CARTESIAN_POINT('Ctrl Pts',(-0.000533142046554097,0.721955694190449,
1.43924894711389));
#38621=CARTESIAN_POINT('Ctrl Pts',(-0.3462403019764,0.633512400747956,1.45117231722863));
#38622=CARTESIAN_POINT('Ctrl Pts',(-0.60735993632721,0.390300161874371,
1.46309568734337));
#38623=CARTESIAN_POINT('Ctrl Pts',(-0.72009974933307,0.0517364438747562,
1.47501905745811));
#38624=CARTESIAN_POINT('Ctrl Pts',(-0.656917072615711,-0.299466639743793,
1.48694242757285));
#38625=CARTESIAN_POINT('Ctrl Pts',(-0.433247620194335,-0.577509141237938,
1.49886579768759));
#38626=CARTESIAN_POINT('Ctrl Pts',(-0.103734498083544,-0.714464458538322,
1.51078916780233));
#38627=CARTESIAN_POINT('Ctrl Pts',(0.251121267443708,-0.676874004276149,
1.52271253791707));
#38628=CARTESIAN_POINT('Ctrl Pts',(0.54462736769301,-0.473921237081957,
1.53463590803181));
#38629=CARTESIAN_POINT('Ctrl Pts',(0.705079397877607,-0.155188115879031,
1.54655927814655));
#38630=CARTESIAN_POINT('Ctrl Pts',(0.693278454455557,0.201457919287497,
1.55848264826129));
#38631=CARTESIAN_POINT('Ctrl Pts',(0.512107542617394,0.508887191069639,
1.57040601837603));
#38632=CARTESIAN_POINT('Ctrl Pts',(0.2058272498316,0.691993823877357,1.58232938849077));
#38633=CARTESIAN_POINT('Ctrl Pts',(-0.150737246446145,0.706044326008023,
1.59425275860551));
#38634=CARTESIAN_POINT('Ctrl Pts',(-0.470476189200041,0.547606122371807,
1.60617612872025));
#38635=CARTESIAN_POINT('Ctrl Pts',(-0.675276413683305,0.255386124880614,
1.61809949883499));
#38636=CARTESIAN_POINT('Ctrl Pts',(-0.715104620412515,-0.0992254446575641,
1.63002286894973));
#38637=CARTESIAN_POINT('Ctrl Pts',(-0.580230664021831,-0.429595966658007,
1.64194623906447));
#38638=CARTESIAN_POINT('Ctrl Pts',(-0.303604643641527,-0.655014887165163,
1.65386960917921));
#38639=CARTESIAN_POINT('Ctrl Pts',(0.0471928778916124,-0.720411824163075,
1.66579297929395));
#38640=CARTESIAN_POINT('Ctrl Pts',(0.386461055325867,-0.60980986596366,
1.67771634940869));
#38641=CARTESIAN_POINT('Ctrl Pts',(0.631315628858409,-0.350229889347576,
1.68963971952343));
#38642=CARTESIAN_POINT('Ctrl Pts',(0.721937994178612,-0.00508706607374287,
1.70156308963817));
#38643=CARTESIAN_POINT('Ctrl Pts',(0.636188662895073,0.341297241686589,
1.71348645975291));
#38644=CARTESIAN_POINT('Ctrl Pts',(0.395016802958407,0.604304218531258,
1.72540982986765));
#38645=CARTESIAN_POINT('Ctrl Pts',(0.0573407055317036,0.719672735761348,
1.73733319998239));
#38646=CARTESIAN_POINT('Ctrl Pts',(-0.294342960467388,0.659233359843414,
1.74925657009713));
#38647=CARTESIAN_POINT('Ctrl Pts',(-0.574119642516605,0.437720850900241,
1.76117994021187));
#38648=CARTESIAN_POINT('Ctrl Pts',(-0.713633396083747,0.109312853268001,
1.77310331032661));
#38649=CARTESIAN_POINT('Ctrl Pts',(-0.678813010196804,-0.245884850466584,
1.78502668044135));
#38650=CARTESIAN_POINT('Ctrl Pts',(-0.545017688013148,-0.442496800345716,
1.79297559385118));
#38651=CARTESIAN_POINT('Ctrl Pts',(-0.458638402619086,-0.518851679811305,
1.79695005055609));
#38652=CARTESIAN_POINT('Ctrl Pts',(-0.692483926679543,-1.76726015421153E-5,
1.62673131746348));
#38653=CARTESIAN_POINT('Ctrl Pts',(-0.692514701573625,-0.0318455918606296,
1.62782850129223));
#38654=CARTESIAN_POINT('Ctrl Pts',(-0.690360629478052,-0.0636693787307131,
1.62892568512098));
#38655=CARTESIAN_POINT('Ctrl Pts',(-0.685987593225867,-0.0951852700679401,
1.63002286894973));
#38656=CARTESIAN_POINT('Ctrl Pts',(-0.670146634948955,-0.209348951991043,
1.63399732565464));
#38657=CARTESIAN_POINT('Ctrl Pts',(-0.625188649485394,-0.319472459324523,
1.63797178235956));
#38658=CARTESIAN_POINT('Ctrl Pts',(-0.556605320023564,-0.412104033075788,
1.64194623906447));
#38659=CARTESIAN_POINT('Ctrl Pts',(-0.488021990561732,-0.504735606827057,
1.64592069576938));
#38660=CARTESIAN_POINT('Ctrl Pts',(-0.39581331710163,-0.57987524699611,
1.6498951524743));
#38661=CARTESIAN_POINT('Ctrl Pts',(-0.291242726782721,-0.628344556580289,
1.65386960917921));
#38662=CARTESIAN_POINT('Ctrl Pts',(-0.186672136463813,-0.676813866164467,
1.65784406588412));
#38663=CARTESIAN_POINT('Ctrl Pts',(-0.0697396292860975,-0.698612845163772,
1.66181852258904));
#38664=CARTESIAN_POINT('Ctrl Pts',(0.0452713205418031,-0.69107867496352,
1.66579297929395));
#38665=CARTESIAN_POINT('Ctrl Pts',(0.160282270369701,-0.683544504763269,
1.66976743599886));
#38666=CARTESIAN_POINT('Ctrl Pts',(0.273371662847784,-0.646677185363464,
1.67374189270378));
#38667=CARTESIAN_POINT('Ctrl Pts',(0.370725454675582,-0.584980196227548,
1.67771634940869));
#38668=CARTESIAN_POINT('Ctrl Pts',(0.468079246503381,-0.523283207091632,
1.6816908061136));
#38669=CARTESIAN_POINT('Ctrl Pts',(0.549697437680895,-0.436756548219604,
1.68566526281852));
#38670=CARTESIAN_POINT('Ctrl Pts',(0.605610260823019,-0.335969414904618,
1.68963971952343));
#38671=CARTESIAN_POINT('Ctrl Pts',(0.661523083965143,-0.235182281589633,
1.69361417622834));
#38672=CARTESIAN_POINT('Ctrl Pts',(0.691730539071877,-0.120134673831689,
1.69758863293326));
#38673=CARTESIAN_POINT('Ctrl Pts',(0.692542711411322,-0.00488015199266319,
1.70156308963817));
#38674=CARTESIAN_POINT('Ctrl Pts',(0.693354883750767,0.110374369846365,
1.70553754634308));
#38675=CARTESIAN_POINT('Ctrl Pts',(0.664771773322921,0.225835805766476,
1.709512003048));
#38676=CARTESIAN_POINT('Ctrl Pts',(0.610284908119553,0.32740101986731,1.71348645975291));
#38677=CARTESIAN_POINT('Ctrl Pts',(0.555798042916185,0.428966233968145,
1.71746091645782));
#38678=CARTESIAN_POINT('Ctrl Pts',(0.475407422937294,0.516635226249703,
1.72143537316274));
#38679=CARTESIAN_POINT('Ctrl Pts',(0.37893276337673,0.579697808595497,1.72540982986765));
#38680=CARTESIAN_POINT('Ctrl Pts',(0.282458103816171,0.642760390941288,
1.72938428657257));
#38681=CARTESIAN_POINT('Ctrl Pts',(0.16989940467394,0.681216563351317,1.73335874327748));
#38682=CARTESIAN_POINT('Ctrl Pts',(0.0550061107696439,0.690371420236677,
1.73733319998239));
#38683=CARTESIAN_POINT('Ctrl Pts',(-0.0429609179519917,0.698177568854695,
1.74072213332159));
#38684=CARTESIAN_POINT('Ctrl Pts',(-0.142625338155946,0.684679890273028,
1.7441110666608));
#38685=CARTESIAN_POINT('Ctrl Pts',(-0.235110047033021,0.651400850437653,
1.7475));
#38686=CARTESIAN_POINT('',(-0.352210602859808,-0.494214587872355,0.7));
#38687=CARTESIAN_POINT('Ctrl Pts',(-0.352210602859807,-0.494214587872356,
0.7));
#38688=CARTESIAN_POINT('Ctrl Pts',(-0.36497036554318,-0.486388617262107,
0.7));
#38689=CARTESIAN_POINT('Ctrl Pts',(-0.377422115114145,-0.478097231538959,
0.7));
#38690=CARTESIAN_POINT('Ctrl Pts',(-0.389538285381734,-0.469355126779466,
0.7));
#38691=CARTESIAN_POINT('Ctrl Pts',(-0.410503962208501,-0.454227892750445,
0.7));
#38692=CARTESIAN_POINT('Ctrl Pts',(-0.430465714824907,-0.437752457865635,
0.7));
#38693=CARTESIAN_POINT('Ctrl Pts',(-0.449338856342161,-0.420064848170144,
0.7));
#38694=CARTESIAN_POINT('Ctrl Pts',(-0.457610580625059,-0.412312719013964,
0.7));
#38695=CARTESIAN_POINT('Ctrl Pts',(-0.465673023775416,-0.404327425803387,
0.7));
#38696=CARTESIAN_POINT('Ctrl Pts',(-0.473518124711072,-0.396119066458196,
0.7));
#38697=CARTESIAN_POINT('Ctrl Pts',(-0.479686699886945,-0.389664862477052,
0.7));
#38698=CARTESIAN_POINT('Ctrl Pts',(-0.485715597961141,-0.383078107397374,
0.7));
#38699=CARTESIAN_POINT('Ctrl Pts',(-0.491596494353867,-0.376370061034681,
0.7));
#38700=CARTESIAN_POINT('Ctrl Pts',(-0.510513872818444,-0.354791947201907,
0.7));
#38701=CARTESIAN_POINT('Ctrl Pts',(-0.52791835675801,-0.331943614932878,
0.7));
#38702=CARTESIAN_POINT('Ctrl Pts',(-0.543691212400513,-0.30799896208282,
0.7));
#38703=CARTESIAN_POINT('Ctrl Pts',(-0.550562789889049,-0.297567272271884,
0.7));
#38704=CARTESIAN_POINT('Ctrl Pts',(-0.557124381433215,-0.286927116134095,
0.7));
#38705=CARTESIAN_POINT('Ctrl Pts',(-0.563364546006299,-0.276091296564536,
0.7));
#38706=CARTESIAN_POINT('Ctrl Pts',(-0.568428809706163,-0.267297386233855,
0.7));
#38707=CARTESIAN_POINT('Ctrl Pts',(-0.573283304388212,-0.258370224031322,
0.7));
#38708=CARTESIAN_POINT('Ctrl Pts',(-0.577908406198614,-0.249343210279803,
0.7));
#38709=CARTESIAN_POINT('Ctrl Pts',(-0.580665693855551,-0.243961691209221,
0.7));
#38710=CARTESIAN_POINT('Ctrl Pts',(-0.58334242566026,-0.238543142886124,
0.7));
#38711=CARTESIAN_POINT('Ctrl Pts',(-0.585937631284055,-0.233089224075231,
0.7));
#38712=CARTESIAN_POINT('Ctrl Pts',(-0.599348617917031,-0.204905548916861,
0.7));
#38713=CARTESIAN_POINT('Ctrl Pts',(-0.610585988612837,-0.175780088337437,
0.7));
#38714=CARTESIAN_POINT('Ctrl Pts',(-0.619650220520174,-0.145982170082658,
0.7));
#38715=CARTESIAN_POINT('Ctrl Pts',(-0.625666313261402,-0.126204759095282,
0.7));
#38716=CARTESIAN_POINT('Ctrl Pts',(-0.630724246458381,-0.106130286941727,
0.7));
#38717=CARTESIAN_POINT('Ctrl Pts',(-0.634813159904227,-0.0858312982855508,
0.7));
#38718=CARTESIAN_POINT('Ctrl Pts',(-0.638007544190021,-0.0699731072918824,
0.7));
#38719=CARTESIAN_POINT('Ctrl Pts',(-0.64061034690479,-0.0539777735229824,
0.7));
#38720=CARTESIAN_POINT('Ctrl Pts',(-0.642612357401729,-0.0378788650432131,
0.7));
#38721=CARTESIAN_POINT('Ctrl Pts',(-0.643611959428883,-0.0298406946260486,
0.7));
#38722=CARTESIAN_POINT('Ctrl Pts',(-0.644461654683445,-0.0217750894774087,
0.7));
#38723=CARTESIAN_POINT('Ctrl Pts',(-0.64515871908081,-0.013707778299405,
0.7));
#38724=CARTESIAN_POINT('Ctrl Pts',(-0.647813160179314,0.0170127726658416,
0.7));
#38725=CARTESIAN_POINT('Ctrl Pts',(-0.648267403763968,0.047826312089933,
0.7));
#38726=CARTESIAN_POINT('Ctrl Pts',(-0.646505170576517,0.0784946399697625,
0.7));
#38727=CARTESIAN_POINT('Ctrl Pts',(-0.644925352961593,0.105988370623497,
0.7));
#38728=CARTESIAN_POINT('Ctrl Pts',(-0.641563835892215,0.133366243242613,
0.7));
#38729=CARTESIAN_POINT('Ctrl Pts',(-0.636488118893852,0.160474361536191,
0.7));
#38730=CARTESIAN_POINT('Ctrl Pts',(-0.633437102007,0.176769069596382,0.7));
#38731=CARTESIAN_POINT('Ctrl Pts',(-0.629766130645052,0.192966361518495,
0.7));
#38732=CARTESIAN_POINT('Ctrl Pts',(-0.625484875914611,0.209032279224361,
0.7));
#38733=CARTESIAN_POINT('Ctrl Pts',(-0.62304510995881,0.218187791226195,
0.7));
#38734=CARTESIAN_POINT('Ctrl Pts',(-0.620405409729918,0.227305241293198,
0.7));
#38735=CARTESIAN_POINT('Ctrl Pts',(-0.617576713553974,0.236349483890122,
0.7));
#38736=CARTESIAN_POINT('Ctrl Pts',(-0.607811223479739,0.26757286590631,
0.7));
#38737=CARTESIAN_POINT('Ctrl Pts',(-0.595783965556306,0.297983461557127,
0.7));
#38738=CARTESIAN_POINT('Ctrl Pts',(-0.581617391728963,0.327334207529254,
0.7));
#38739=CARTESIAN_POINT('Ctrl Pts',(-0.57115026730193,0.349020319772111,
0.7));
#38740=CARTESIAN_POINT('Ctrl Pts',(-0.559514084397962,0.370128096695649,
0.7));
#38741=CARTESIAN_POINT('Ctrl Pts',(-0.546740333913183,0.39055431750125,
0.7));
#38742=CARTESIAN_POINT('Ctrl Pts',(-0.538417752622244,0.403862772470983,
0.7));
#38743=CARTESIAN_POINT('Ctrl Pts',(-0.529611960051848,0.416881820243619,
0.7));
#38744=CARTESIAN_POINT('Ctrl Pts',(-0.520343957444037,0.429592821067772,
0.7));
#38745=CARTESIAN_POINT('Ctrl Pts',(-0.514967230973053,0.436966963857323,
0.7));
#38746=CARTESIAN_POINT('Ctrl Pts',(-0.509434897530512,0.444237402262534,
0.7));
#38747=CARTESIAN_POINT('Ctrl Pts',(-0.503750712659283,0.451400231561865,
0.7));
#38748=CARTESIAN_POINT('Ctrl Pts',(-0.499397667086255,0.456885648218461,
0.7));
#38749=CARTESIAN_POINT('Ctrl Pts',(-0.494961350852985,0.462300618792668,
0.7));
#38750=CARTESIAN_POINT('Ctrl Pts',(-0.490445443674977,0.467642281239387,
0.7));
#38751=CARTESIAN_POINT('Ctrl Pts',(-0.469115242788121,0.492872811577385,
0.7));
#38752=CARTESIAN_POINT('Ctrl Pts',(-0.446004140490849,0.516481055544471,
0.7));
#38753=CARTESIAN_POINT('Ctrl Pts',(-0.421338470315635,0.538318276477707,
0.7));
#38754=CARTESIAN_POINT('Ctrl Pts',(-0.396566506146609,0.560249602513714,
0.7));
#38755=CARTESIAN_POINT('Ctrl Pts',(-0.370225710165849,0.580395556122258,
0.7));
#38756=CARTESIAN_POINT('Ctrl Pts',(-0.342503869424491,0.598574832510096,
0.7));
#38757=CARTESIAN_POINT('Ctrl Pts',(-0.32927347105657,0.607250990449811,
0.7));
#38758=CARTESIAN_POINT('Ctrl Pts',(-0.315727980106861,0.615478656494124,
0.7));
#38759=CARTESIAN_POINT('Ctrl Pts',(-0.301885354887798,0.623234692956248,
0.7));
#38760=CARTESIAN_POINT('Ctrl Pts',(-0.352210602859808,-0.494214587872355,
0.7));
#38761=CARTESIAN_POINT('Ctrl Pts',(-0.282018959374219,-0.544135188072469,
0.703388933339203));
#38762=CARTESIAN_POINT('Ctrl Pts',(-0.106195501050124,-0.620012906324691,
0.71075232338332));
#38763=CARTESIAN_POINT('Ctrl Pts',(0.190680748588941,-0.603244694242624,
0.72209017013235));
#38764=CARTESIAN_POINT('Ctrl Pts',(0.456305609272025,-0.438231596848221,
0.734013540247088));
#38765=CARTESIAN_POINT('Ctrl Pts',(0.61045325274331,-0.166159471325954,
0.74593691036183));
#38766=CARTESIAN_POINT('Ctrl Pts',(0.615465575874622,0.146507028070995,
0.75786028047657));
#38767=CARTESIAN_POINT('Ctrl Pts',(0.470117741946454,0.423380863786649,
0.76978365059131));
#38768=CARTESIAN_POINT('Ctrl Pts',(0.209918811260263,0.596821791269607,
0.78170702070605));
#38769=CARTESIAN_POINT('Ctrl Pts',(-0.101563929551992,0.624457254778657,
0.79363039082079));
#38770=CARTESIAN_POINT('Ctrl Pts',(-0.388234290052265,0.499536043242417,
0.805553760935531));
#38771=CARTESIAN_POINT('Ctrl Pts',(-0.568693105522331,0.267208012438397,
0.816770719631062));
#38772=CARTESIAN_POINT('Ctrl Pts',(-0.606782841646979,0.0830496507577644,
0.824013221621682));
#38773=CARTESIAN_POINT('Ctrl Pts',(-0.606867041669442,-1.46440865504086E-5,
0.827281266907388));
#38774=CARTESIAN_POINT('Origin',(0.,0.,0.422718733092612));
#38775=CARTESIAN_POINT('',(0.352184336898731,-0.494199469185471,0.7));
#38776=CARTESIAN_POINT('Origin',(0.,0.,0.7));
#38777=CARTESIAN_POINT('Ctrl Pts',(0.352184336898731,-0.494199469185471,
0.7));
#38778=CARTESIAN_POINT('Ctrl Pts',(0.434459481514031,-0.435567238565425,
0.703974456704914));
#38779=CARTESIAN_POINT('Ctrl Pts',(0.569074170603496,-0.276472369691842,
0.71192337011474));
#38780=CARTESIAN_POINT('Ctrl Pts',(0.63195675641648,0.0298991715734713,
0.72384674022948));
#38781=CARTESIAN_POINT('Ctrl Pts',(0.540450411763527,0.328891738414737,
0.73577011034422));
#38782=CARTESIAN_POINT('Ctrl Pts',(0.316910788923287,0.547571327639118,
0.747693480458961));
#38783=CARTESIAN_POINT('Ctrl Pts',(0.0159487222523762,0.632459517004967,
0.759616850573701));
#38784=CARTESIAN_POINT('Ctrl Pts',(-0.288909559125321,0.562845076658027,
0.771540220688441));
#38785=CARTESIAN_POINT('Ctrl Pts',(-0.523186437261898,0.355721357715825,
0.783463590803182));
#38786=CARTESIAN_POINT('Ctrl Pts',(-0.601100288213809,0.140537724272643,
0.792189761604571));
#38787=CARTESIAN_POINT('Ctrl Pts',(-0.606881754382541,0.0197715030368324,
0.796941475701048));
#38788=CARTESIAN_POINT('Ctrl Pts',(-0.606861373480359,1.53279143725385E-5,
0.797718733092612));
#38789=CARTESIAN_POINT('Ctrl Pts',(0.401891164706881,-0.563950123442266,
0.650549949443909));
#38790=CARTESIAN_POINT('Ctrl Pts',(0.495778513551069,-0.497042617955932,
0.654524406148822));
#38791=CARTESIAN_POINT('Ctrl Pts',(0.649392540401945,-0.31549331138107,
0.662473319558649));
#38792=CARTESIAN_POINT('Ctrl Pts',(0.721150290546943,0.034119100790357,
0.674396689673389));
#38793=CARTESIAN_POINT('Ctrl Pts',(0.616728862398028,0.375311079924535,
0.686320059788129));
#38794=CARTESIAN_POINT('Ctrl Pts',(0.361639155193832,0.624854814847309,
0.698243429902869));
#38795=CARTESIAN_POINT('Ctrl Pts',(0.0181997036496196,0.721724010094651,
0.710166800017609));
#38796=CARTESIAN_POINT('Ctrl Pts',(-0.329685869150999,0.642284280441105,
0.72209017013235));
#38797=CARTESIAN_POINT('Ctrl Pts',(-0.597028273550075,0.405927395926852,
0.734013540247089));
#38798=CARTESIAN_POINT('Ctrl Pts',(-0.718514881844642,0.0704038725978844,
0.745936910361831));
#38799=CARTESIAN_POINT('Ctrl Pts',(-0.664466203491914,-0.282320840499199,
0.757860280476569));
#38800=CARTESIAN_POINT('Ctrl Pts',(-0.448086466848367,-0.566073079281933,
0.769783650591311));
#38801=CARTESIAN_POINT('Ctrl Pts',(-0.122237890431146,-0.711532329868227,
0.781707020706049));
#38802=CARTESIAN_POINT('Ctrl Pts',(0.233473764593078,-0.683161969529758,
0.79363039082079));
#38803=CARTESIAN_POINT('Ctrl Pts',(0.532147090286164,-0.487893211791223,
0.80555376093553));
#38804=CARTESIAN_POINT('Ctrl Pts',(0.700815314941263,-0.17343066321587,
0.81747713105027));
#38805=CARTESIAN_POINT('Ctrl Pts',(0.698272293749139,0.183401486010904,
0.829400501165011));
#38806=CARTESIAN_POINT('Ctrl Pts',(0.525139294646749,0.495428122667492,
0.841323871279751));
#38807=CARTESIAN_POINT('Ctrl Pts',(0.223713219070008,0.686420204386435,
0.853247241394491));
#38808=CARTESIAN_POINT('Ctrl Pts',(-0.132366654812752,0.70971781110012,
0.865170611509231));
#38809=CARTESIAN_POINT('Ctrl Pts',(-0.456108965071534,0.559629264828852,
0.877093981623971));
#38810=CARTESIAN_POINT('Ctrl Pts',(-0.668422511745348,0.272821641522934,
0.889017351738711));
#38811=CARTESIAN_POINT('Ctrl Pts',(-0.717438470051463,-0.0806371127090915,
0.900940721853451));
#38812=CARTESIAN_POINT('Ctrl Pts',(-0.591182096999562,-0.414395982628671,
0.912864091968191));
#38813=CARTESIAN_POINT('Ctrl Pts',(-0.320498196401073,-0.646916693528293,
0.924787462082932));
#38814=CARTESIAN_POINT('Ctrl Pts',(0.0284843575647898,-0.721393750746014,
0.936710832197671));
#38815=CARTESIAN_POINT('Ctrl Pts',(0.370508099080321,-0.619632189906009,
0.948634202312412));
#38816=CARTESIAN_POINT('Ctrl Pts',(0.622015620706852,-0.366492660014364,
0.960557572427151));
#38817=CARTESIAN_POINT('Ctrl Pts',(0.721562894127873,-0.0238178938298552,
0.972480942541893));
#38818=CARTESIAN_POINT('Ctrl Pts',(0.644830227243077,0.324675653972579,
0.984404312656631));
#38819=CARTESIAN_POINT('Ctrl Pts',(0.410563636578539,0.593849983217877,
0.996327682771373));
#38820=CARTESIAN_POINT('Ctrl Pts',(0.0759951402356486,0.717945012455233,
1.00825105288611));
#38821=CARTESIAN_POINT('Ctrl Pts',(-0.277139192700696,0.666643960535019,
1.02017442300085));
#38822=CARTESIAN_POINT('Ctrl Pts',(-0.562567604582521,0.452479825542494,
1.03209779311559));
#38823=CARTESIAN_POINT('Ctrl Pts',(-0.710559093694536,0.127773536448902,
1.04402116323033));
#38824=CARTESIAN_POINT('Ctrl Pts',(-0.68495890335684,-0.228148203939579,
1.05594453334507));
#38825=CARTESIAN_POINT('Ctrl Pts',(-0.492021235470988,-0.528332666124543,
1.06786790345981));
#38826=CARTESIAN_POINT('Ctrl Pts',(-0.178881330574504,-0.699443901839566,
1.07979127357455));
#38827=CARTESIAN_POINT('Ctrl Pts',(0.177959810253215,-0.699678932213415,
1.09171464368929));
#38828=CARTESIAN_POINT('Ctrl Pts',(0.49132484527841,-0.528980338633497,
1.10363801380403));
#38829=CARTESIAN_POINT('Ctrl Pts',(0.684657773468146,-0.229050290282077,
1.11556138391877));
#38830=CARTESIAN_POINT('Ctrl Pts',(0.710726791028474,0.126837418623334,
1.12748475403351));
#38831=CARTESIAN_POINT('Ctrl Pts',(0.563163160186478,0.451738372575811,
1.13940812414825));
#38832=CARTESIAN_POINT('Ctrl Pts',(0.278017110586494,0.666278311570923,
1.15133149426299));
#38833=CARTESIAN_POINT('Ctrl Pts',(-0.0750493379933025,0.718044496612453,
1.16325486437773));
#38834=CARTESIAN_POINT('Ctrl Pts',(-0.409781012253192,0.594390296224132,
1.17517823449247));
#38835=CARTESIAN_POINT('Ctrl Pts',(-0.644401978262523,0.325524795768324,
1.18710160460721));
#38836=CARTESIAN_POINT('Ctrl Pts',(-0.721593642979431,-0.0228673710849739,
1.19902497472196));
#38837=CARTESIAN_POINT('Ctrl Pts',(-0.622497855355482,-0.365672971829322,
1.21094834483669));
#38838=CARTESIAN_POINT('Ctrl Pts',(-0.371324008181069,-0.619143588513205,
1.22287171495144));
#38839=CARTESIAN_POINT('Ctrl Pts',(-0.0294346121210613,-0.72135560291575,
1.23479508506617));
#38840=CARTESIAN_POINT('Ctrl Pts',(0.319645746375974,-0.647338318866116,
1.24671845518092));
#38841=CARTESIAN_POINT('Ctrl Pts',(0.590635707558052,-0.41517437686599,
1.25864182529565));
#38842=CARTESIAN_POINT('Ctrl Pts',(0.717331625742423,-0.0815821117549382,
1.2705651954104));
#38843=CARTESIAN_POINT('Ctrl Pts',(0.668781314950164,0.271940903547428,
1.28248856552513));
#38844=CARTESIAN_POINT('Ctrl Pts',(0.456845759106501,0.559027955146312,
1.29441193563988));
#38845=CARTESIAN_POINT('Ctrl Pts',(0.133301438732876,0.709542830758235,
1.30633530575461));
#38846=CARTESIAN_POINT('Ctrl Pts',(-0.222808815745382,0.686714302949052,
1.31825867586936));
#38847=CARTESIAN_POINT('Ctrl Pts',(-0.524486220282421,0.496119448301036,
1.33018204598409));
#38848=CARTESIAN_POINT('Ctrl Pts',(-0.698030096397969,0.18432115117724,
1.34210541609884));
#38849=CARTESIAN_POINT('Ctrl Pts',(-0.701043164005901,-0.172507346073306,
1.35402878621357));
#38850=CARTESIAN_POINT('Ctrl Pts',(-0.532789321814994,-0.487191790580056,
1.36595215632832));
#38851=CARTESIAN_POINT('Ctrl Pts',(-0.23437347904248,-0.682853845687445,
1.37787552644306));
#38852=CARTESIAN_POINT('Ctrl Pts',(0.12130049497697,-0.711692695035662,
1.3897988965578));
#38853=CARTESIAN_POINT('Ctrl Pts',(0.44734040079856,-0.566662922787304,
1.40172226667254));
#38854=CARTESIAN_POINT('Ctrl Pts',(0.664093729121677,-0.283195729470173,
1.41364563678728));
#38855=CARTESIAN_POINT('Ctrl Pts',(0.718607003417866,0.0694570146743853,
1.42556900690202));
#38856=CARTESIAN_POINT('Ctrl Pts',(0.597562470215061,0.405141205554568,
1.43749237701676));
#38857=CARTESIAN_POINT('Ctrl Pts',(0.330531665495144,0.641848206632094,
1.4494157471315));
#38858=CARTESIAN_POINT('Ctrl Pts',(-0.0172489986427966,0.721749800337417,
1.46133911724624));
#38859=CARTESIAN_POINT('Ctrl Pts',(-0.360815681609231,0.625325792021076,
1.47326248736098));
#38860=CARTESIAN_POINT('Ctrl Pts',(-0.616234030819248,0.376132850854382,
1.48518585747572));
#38861=CARTESIAN_POINT('Ctrl Pts',(-0.72110459126874,0.0350495464590682,
1.49710922759046));
#38862=CARTESIAN_POINT('Ctrl Pts',(-0.649807176137898,-0.314596465541046,
1.5090325977052));
#38863=CARTESIAN_POINT('Ctrl Pts',(-0.419759953978916,-0.587385634066009,
1.52095596781994));
#38864=CARTESIAN_POINT('Ctrl Pts',(-0.0871641386632488,-0.716674762797015,
1.53287933793468));
#38865=CARTESIAN_POINT('Ctrl Pts',(0.266726132357388,-0.670878134756418,
1.54480270804942));
#38866=CARTESIAN_POINT('Ctrl Pts',(0.555454423837073,-0.461184005090966,
1.55672607816416));
#38867=CARTESIAN_POINT('Ctrl Pts',(0.70848356315327,-0.138821259288117,
1.5686494482789));
#38868=CARTESIAN_POINT('Ctrl Pts',(0.688428082041725,0.217455918420426,
1.58057281839364));
#38869=CARTESIAN_POINT('Ctrl Pts',(0.500187591224132,0.520607995902278,
1.59249618850838));
#38870=CARTESIAN_POINT('Ctrl Pts',(0.189749801791051,0.696573964547411,
1.60441955862312));
#38871=CARTESIAN_POINT('Ctrl Pts',(-0.167044429389013,0.702364945676295,
1.61634292873786));
#38872=CARTESIAN_POINT('Ctrl Pts',(-0.483029201952088,0.536565935297714,
1.6282662988526));
#38873=CARTESIAN_POINT('Ctrl Pts',(-0.681008542672965,0.239682617996334,
1.64018966896734));
#38874=CARTESIAN_POINT('Ctrl Pts',(-0.712615441052988,-0.115756528463215,
1.65211303908208));
#38875=CARTESIAN_POINT('Ctrl Pts',(-0.570128386861848,-0.442914701355064,
1.66403640919682));
#38876=CARTESIAN_POINT('Ctrl Pts',(-0.288357092310038,-0.66187012059323,
1.67595977931156));
#38877=CARTESIAN_POINT('Ctrl Pts',(0.0638602987601055,-0.719123520824002,
1.6878831494263));
#38878=CARTESIAN_POINT('Ctrl Pts',(0.400477207465661,-0.600703274926714,
1.69980651954104));
#38879=CARTESIAN_POINT('Ctrl Pts',(0.639254813111137,-0.335508837950853,
1.71172988965578));
#38880=CARTESIAN_POINT('Ctrl Pts',(0.721863601446102,0.0116101465083443,
1.72365325977052));
#38881=CARTESIAN_POINT('Ctrl Pts',(0.628113563405619,0.355977601151784,
1.73557662988526));
#38882=CARTESIAN_POINT('Ctrl Pts',(0.463312679049696,0.527436308946575,
1.74352554329509));
#38883=CARTESIAN_POINT('Ctrl Pts',(0.365377360036757,0.58826493586867,1.7475));
#38884=CARTESIAN_POINT('Ctrl Pts',(0.385322222104164,-0.540699905356667,
0.667033299629272));
#38885=CARTESIAN_POINT('Ctrl Pts',(0.475338836205389,-0.476550824825763,
0.671007756334186));
#38886=CARTESIAN_POINT('Ctrl Pts',(0.622619750469128,-0.302486330817994,
0.678956669744013));
#38887=CARTESIAN_POINT('Ctrl Pts',(0.691419112503455,0.0327124577180616,
0.690880039858753));
#38888=CARTESIAN_POINT('Ctrl Pts',(0.591302712186528,0.359837966087936,
0.702803409973493));
#38889=CARTESIAN_POINT('Ctrl Pts',(0.346729699770317,0.599093652444579,
0.714726780088233));
#38890=CARTESIAN_POINT('Ctrl Pts',(0.0174493765172051,0.691969179064757,
0.726650150202973));
#38891=CARTESIAN_POINT('Ctrl Pts',(-0.316093765809106,0.615804545846745,
0.738573520317714));
#38892=CARTESIAN_POINT('Ctrl Pts',(-0.572414328120683,0.38919204985651,
0.750496890432453));
#38893=CARTESIAN_POINT('Ctrl Pts',(-0.688892354946931,0.0675013013882525,
0.762420260547194));
#38894=CARTESIAN_POINT('Ctrl Pts',(-0.637071965066363,-0.270681475883673,
0.774343630661933));
#38895=CARTESIAN_POINT('Ctrl Pts',(-0.429613010345087,-0.542735337168578,
0.786267000776674));
#38896=CARTESIAN_POINT('Ctrl Pts',(-0.117198335526006,-0.682197675690988,
0.798190370891414));
#38897=CARTESIAN_POINT('Ctrl Pts',(0.223848239713465,-0.654996952591022,
0.810113741006154));
#38898=CARTESIAN_POINT('Ctrl Pts',(0.510208029740792,-0.467778625225678,
0.822037111120894));
#38899=CARTESIAN_POINT('Ctrl Pts',(0.671922495819859,-0.166280561504948,
0.833960481235634));
#38900=CARTESIAN_POINT('Ctrl Pts',(0.669484316873271,0.175840312833126,
0.845883851350375));
#38901=CARTESIAN_POINT('Ctrl Pts',(0.503489147553371,0.475002891039828,
0.857807221465114));
#38902=CARTESIAN_POINT('Ctrl Pts',(0.214490096464305,0.658120858775991,
0.869730591579855));
#38903=CARTESIAN_POINT('Ctrl Pts',(-0.126909516913974,0.680457964880758,
0.881653961694594));
#38904=CARTESIAN_POINT('Ctrl Pts',(-0.437304761529596,0.53655718466876,
0.893577331809335));
#38905=CARTESIAN_POINT('Ctrl Pts',(-0.640865164871226,0.261573904533071,
0.905500701924074));
#38906=CARTESIAN_POINT('Ctrl Pts',(-0.687860320852951,-0.0773126512392803,
0.917424072038815));
#38907=CARTESIAN_POINT('Ctrl Pts',(-0.566809174444562,-0.3973114984351,
0.929347442153555));
#38908=CARTESIAN_POINT('Ctrl Pts',(-0.307284877257029,-0.620245976416043,
0.941270812268296));
#38909=CARTESIAN_POINT('Ctrl Pts',(0.0273100205128412,-0.69165253546255,
0.953194182383035));
#38910=CARTESIAN_POINT('Ctrl Pts',(0.355232999833039,-0.594086342943096,
0.965117552497776));
#38911=CARTESIAN_POINT('Ctrl Pts',(0.596371511001176,-0.35138310702749,
0.977040922612515));
#38912=CARTESIAN_POINT('Ctrl Pts',(0.691814705496321,-0.0228359431167249,
0.988964292727256));
#38913=CARTESIAN_POINT('Ctrl Pts',(0.618245529787783,0.311290108960425,
1.000887662842));
#38914=CARTESIAN_POINT('Ctrl Pts',(0.393637150189633,0.56936707055236,1.01281103295674));
#38915=CARTESIAN_POINT('Ctrl Pts',(0.0728620553927195,0.688345979811773,
1.02473440307148));
#38916=CARTESIAN_POINT('Ctrl Pts',(-0.265713454142422,0.639159938768556,
1.03665777318622));
#38917=CARTESIAN_POINT('Ctrl Pts',(-0.53937438420587,0.433825242121212,
1.04858114330096));
#38918=CARTESIAN_POINT('Ctrl Pts',(-0.681264563550163,0.122505761047289,
1.0605045134157));
#38919=CARTESIAN_POINT('Ctrl Pts',(-0.656719803442273,-0.218742238275356,
1.07242788353044));
#38920=CARTESIAN_POINT('Ctrl Pts',(-0.471736461069982,-0.506550864510311,
1.08435125364518));
#38921=CARTESIAN_POINT('Ctrl Pts',(-0.17150651181941,-0.67060762256517,
1.09627462375992));
#38922=CARTESIAN_POINT('Ctrl Pts',(0.170622983418949,-0.670832963239128,
1.10819799387466));
#38923=CARTESIAN_POINT('Ctrl Pts',(0.471068781260073,-0.50717183514182,
1.1201213639894));
#38924=CARTESIAN_POINT('Ctrl Pts',(0.656431088367041,-0.219607133910158,
1.13204473410414));
#38925=CARTESIAN_POINT('Ctrl Pts',(0.681425347152859,0.121608236960235,
1.14396810421888));
#38926=CARTESIAN_POINT('Ctrl Pts',(0.53994538657879,0.43311435735987,1.15589147433362));
#38927=CARTESIAN_POINT('Ctrl Pts',(0.266555177724046,0.638809364574028,
1.16781484444836));
#38928=CARTESIAN_POINT('Ctrl Pts',(-0.0719552461525682,0.688441362492184,
1.1797382145631));
#38929=CARTESIAN_POINT('Ctrl Pts',(-0.392886791459217,0.569885107838286,
1.19166158467784));
#38930=CARTESIAN_POINT('Ctrl Pts',(-0.617834936415022,0.312104242816431,
1.20358495479258));
#38931=CARTESIAN_POINT('Ctrl Pts',(-0.691844186651542,-0.0219246079882583,
1.21550832490732));
#38932=CARTESIAN_POINT('Ctrl Pts',(-0.596833864351296,-0.350597212485312,
1.22743169502206));
#38933=CARTESIAN_POINT('Ctrl Pts',(-0.356015271092881,-0.593617885333347,
1.2393550651368));
#38934=CARTESIAN_POINT('Ctrl Pts',(-0.0282210985094273,-0.691615960369548,
1.25127843525154));
#38935=CARTESIAN_POINT('Ctrl Pts',(0.306467571561485,-0.620650219221889,
1.26320180536628));
#38936=CARTESIAN_POINT('Ctrl Pts',(0.566285311239232,-0.398057801473175,
1.27512517548102));
#38937=CARTESIAN_POINT('Ctrl Pts',(0.687757881460913,-0.0782186903966656,
1.28704854559576));
#38938=CARTESIAN_POINT('Ctrl Pts',(0.641209175539583,0.260729477126809,
1.2989719157105));
#38939=CARTESIAN_POINT('Ctrl Pts',(0.438011179435034,0.535980665443169,
1.31089528582524));
#38940=CARTESIAN_POINT('Ctrl Pts',(0.127805762089087,0.680290198529863,
1.32281865593998));
#38941=CARTESIAN_POINT('Ctrl Pts',(-0.213622979370609,0.658402832408697,
1.33474202605472));
#38942=CARTESIAN_POINT('Ctrl Pts',(-0.502862997771139,0.475665715089492,
1.34666539616946));
#38943=CARTESIAN_POINT('Ctrl Pts',(-0.669252104698097,0.176722062561917,
1.3585887662842));
#38944=CARTESIAN_POINT('Ctrl Pts',(-0.672140951251578,-0.165395310361548,
1.37051213639894));
#38945=CARTESIAN_POINT('Ctrl Pts',(-0.510823783709841,-0.467106121813182,
1.38243550651368));
#38946=CARTESIAN_POINT('Ctrl Pts',(-0.224710861242244,-0.654701531904951,
1.39435887662842));
#38947=CARTESIAN_POINT('Ctrl Pts',(0.116299586483697,-0.682351429413614,
1.40628224674316));
#38948=CARTESIAN_POINT('Ctrl Pts',(0.428897702686216,-0.543300862938094,
1.4182056168579));
#38949=CARTESIAN_POINT('Ctrl Pts',(0.636714846859693,-0.271520295424869,
1.43012898697264));
#38950=CARTESIAN_POINT('Ctrl Pts',(0.688980678583815,0.0665934799899764,
1.44205235708738));
#38951=CARTESIAN_POINT('Ctrl Pts',(0.572926501226411,0.388438272098131,
1.45397572720212));
#38952=CARTESIAN_POINT('Ctrl Pts',(0.316904692137907,0.615386450243146,
1.46589909731686));
#38953=CARTESIAN_POINT('Ctrl Pts',(-0.0165378666409895,0.691993906041918,
1.4778224674316));
#38954=CARTESIAN_POINT('Ctrl Pts',(-0.345940175890901,0.599545212436668,
1.48974583754634));
#38955=CARTESIAN_POINT('Ctrl Pts',(-0.5908282812454,0.360625857508688,1.50166920766108));
#38956=CARTESIAN_POINT('Ctrl Pts',(-0.691375297289357,0.0336045434967476,
1.51359257777582));
#38957=CARTESIAN_POINT('Ctrl Pts',(-0.623017291836473,-0.301626459633181,
1.52551594789056));
#38958=CARTESIAN_POINT('Ctrl Pts',(-0.402454326995381,-0.563169229946753,
1.5374393180053));
#38959=CARTESIAN_POINT('Ctrl Pts',(-0.0835705846432688,-0.687128099291087,
1.54936268812004));
#38960=CARTESIAN_POINT('Ctrl Pts',(0.255729697586553,-0.643219548839746,
1.56128605823478));
#38961=CARTESIAN_POINT('Ctrl Pts',(0.532554461670217,-0.442170570657251,
1.57320942834952));
#38962=CARTESIAN_POINT('Ctrl Pts',(0.67927460181316,-0.133098014591112,
1.58513279846426));
#38963=CARTESIAN_POINT('Ctrl Pts',(0.660045956782098,0.208490768281939,
1.597056168579));
#38964=CARTESIAN_POINT('Ctrl Pts',(0.479566138907238,0.499144662641613,
1.60897953869374));
#38965=CARTESIAN_POINT('Ctrl Pts',(0.181926903825513,0.667856005431414,
1.62090290880848));
#38966=CARTESIAN_POINT('Ctrl Pts',(-0.160157615729726,0.673408239251661,
1.63282627892322));
#38967=CARTESIAN_POINT('Ctrl Pts',(-0.463115146044895,0.514444697098797,
1.64474964903796));
#38968=CARTESIAN_POINT('Ctrl Pts',(-0.652932306003921,0.229801118005293,
1.6566730191527));
#38969=CARTESIAN_POINT('Ctrl Pts',(-0.683236132977807,-0.110984183499136,
1.66859638926744));
#38970=CARTESIAN_POINT('Ctrl Pts',(-0.546623454811443,-0.424654463486924,
1.68051975938218));
#38971=CARTESIAN_POINT('Ctrl Pts',(-0.276468868504331,-0.634582912011373,
1.69244312949692));
#38972=CARTESIAN_POINT('Ctrl Pts',(0.0612275023274693,-0.689475901301222,
1.70436649961166));
#38973=CARTESIAN_POINT('Ctrl Pts',(0.383966558695777,-0.575937818610241,
1.7162898697264));
#38974=CARTESIAN_POINT('Ctrl Pts',(0.612899975689733,-0.321676668530641,
1.72821323984114));
#38975=CARTESIAN_POINT('Ctrl Pts',(0.692103015422583,0.0111314899266652,
1.74013660995588));
#38976=CARTESIAN_POINT('Ctrl Pts',(0.602218051152578,0.341301557089859,
1.75205998007063));
#38977=CARTESIAN_POINT('Ctrl Pts',(0.444211484844831,0.505691461841269,
1.76000889348045));
#38978=CARTESIAN_POINT('Ctrl Pts',(0.350313788009248,0.564012280389897,
1.76398335018536));
#38979=CARTESIAN_POINT('Ctrl Pts',(0.368753279501448,-0.517449687271069,
0.683516649814636));
#38980=CARTESIAN_POINT('Ctrl Pts',(0.45489915885971,-0.456059031695594,
0.68749110651955));
#38981=CARTESIAN_POINT('Ctrl Pts',(0.595846960536312,-0.289479350254918,
0.695440019929377));
#38982=CARTESIAN_POINT('Ctrl Pts',(0.661687934459967,0.0313058146457665,
0.707363390044116));
#38983=CARTESIAN_POINT('Ctrl Pts',(0.565876561975028,0.344364852251337,
0.719286760158857));
#38984=CARTESIAN_POINT('Ctrl Pts',(0.331820244346802,0.573332490041849,
0.731210130273597));
#38985=CARTESIAN_POINT('Ctrl Pts',(0.0166990493847907,0.662214348034862,
0.743133500388337));
#38986=CARTESIAN_POINT('Ctrl Pts',(-0.302501662467213,0.589324811252386,
0.755056870503077));
#38987=CARTESIAN_POINT('Ctrl Pts',(-0.54780038269129,0.372456703786168,
0.766980240617817));
#38988=CARTESIAN_POINT('Ctrl Pts',(-0.659269828049221,0.0645987301786208,
0.778903610732558));
#38989=CARTESIAN_POINT('Ctrl Pts',(-0.609677726640811,-0.259042111268147,
0.790826980847297));
#38990=CARTESIAN_POINT('Ctrl Pts',(-0.411139553841808,-0.519397595055222,
0.802750350962038));
#38991=CARTESIAN_POINT('Ctrl Pts',(-0.112158780620866,-0.65286302151375,
0.814673721076777));
#38992=CARTESIAN_POINT('Ctrl Pts',(0.214222714833852,-0.626831935652286,
0.826597091191518));
#38993=CARTESIAN_POINT('Ctrl Pts',(0.48826896919542,-0.447664038660134,
0.838520461306257));
#38994=CARTESIAN_POINT('Ctrl Pts',(0.643029676698454,-0.159130459794026,
0.850443831420999));
#38995=CARTESIAN_POINT('Ctrl Pts',(0.640696339997405,0.168279139655349,
0.862367201535737));
#38996=CARTESIAN_POINT('Ctrl Pts',(0.481839000459992,0.454577659412166,
0.874290571650479));
#38997=CARTESIAN_POINT('Ctrl Pts',(0.205266973858603,0.629821513165547,
0.886213941765218));
#38998=CARTESIAN_POINT('Ctrl Pts',(-0.121452379015197,0.651198118661396,
0.898137311879959));
#38999=CARTESIAN_POINT('Ctrl Pts',(-0.418500557987658,0.513485104508667,
0.910060681994699));
#39000=CARTESIAN_POINT('Ctrl Pts',(-0.613307817997104,0.250326167543209,
0.921984052109438));
#39001=CARTESIAN_POINT('Ctrl Pts',(-0.658282171654439,-0.0739881897694695,
0.933907422224179));
#39002=CARTESIAN_POINT('Ctrl Pts',(-0.542436251889562,-0.380227014241528,
0.945830792338918));
#39003=CARTESIAN_POINT('Ctrl Pts',(-0.294071558112983,-0.593575259303795,
0.957754162453659));
#39004=CARTESIAN_POINT('Ctrl Pts',(0.0261356834608925,-0.661911320179086,
0.969677532568399));
#39005=CARTESIAN_POINT('Ctrl Pts',(0.339957900585757,-0.568540495980184,
0.981600902683139));
#39006=CARTESIAN_POINT('Ctrl Pts',(0.5707274012955,-0.336273554040615,0.993524272797879));
#39007=CARTESIAN_POINT('Ctrl Pts',(0.662066516864767,-0.0218539924035951,
1.00544764291262));
#39008=CARTESIAN_POINT('Ctrl Pts',(0.591660832332492,0.297904563948271,
1.01737101302736));
#39009=CARTESIAN_POINT('Ctrl Pts',(0.376710663800726,0.544884157886843,
1.0292943831421));
#39010=CARTESIAN_POINT('Ctrl Pts',(0.0697289705497912,0.658746947168312,
1.04121775325684));
#39011=CARTESIAN_POINT('Ctrl Pts',(-0.254287715584149,0.611675917002094,
1.05314112337158));
#39012=CARTESIAN_POINT('Ctrl Pts',(-0.516181163829219,0.415170658699929,
1.06506449348632));
#39013=CARTESIAN_POINT('Ctrl Pts',(-0.651970033405789,0.117237985645677,
1.07698786360106));
#39014=CARTESIAN_POINT('Ctrl Pts',(-0.628480703527705,-0.209336272611132,
1.0889112337158));
#39015=CARTESIAN_POINT('Ctrl Pts',(-0.451451686668976,-0.484769062896079,
1.10083460383054));
#39016=CARTESIAN_POINT('Ctrl Pts',(-0.164131693064316,-0.641771343290773,
1.11275797394528));
#39017=CARTESIAN_POINT('Ctrl Pts',(0.163286156584683,-0.641986994264843,
1.12468134406002));
#39018=CARTESIAN_POINT('Ctrl Pts',(0.450812717241737,-0.485363331650142,
1.13660471417476));
#39019=CARTESIAN_POINT('Ctrl Pts',(0.628204403265935,-0.210163977538239,
1.1485280842895));
#39020=CARTESIAN_POINT('Ctrl Pts',(0.652123903277245,0.116379055297137,
1.16045145440424));
#39021=CARTESIAN_POINT('Ctrl Pts',(0.516727612971101,0.414490342143929,
1.17237482451898));
#39022=CARTESIAN_POINT('Ctrl Pts',(0.2550932448616,0.611340417577134,1.18429819463372));
#39023=CARTESIAN_POINT('Ctrl Pts',(-0.0688611543118346,0.658838228371917,
1.19622156474846));
#39024=CARTESIAN_POINT('Ctrl Pts',(-0.37599257066524,0.545379919452438,
1.2081449348632));
#39025=CARTESIAN_POINT('Ctrl Pts',(-0.591267894567521,0.298683689864538,
1.22006830497794));
#39026=CARTESIAN_POINT('Ctrl Pts',(-0.662094730323653,-0.0209818448915428,
1.23199167509268));
#39027=CARTESIAN_POINT('Ctrl Pts',(-0.57116987334711,-0.335521453141302,
1.24391504520742));
#39028=CARTESIAN_POINT('Ctrl Pts',(-0.340706534004693,-0.568092182153489,
1.25583841532216));
#39029=CARTESIAN_POINT('Ctrl Pts',(-0.0270075848977933,-0.661876317823347,
1.2677617854369));
#39030=CARTESIAN_POINT('Ctrl Pts',(0.293289396746996,-0.59396211957766,
1.27968515555164));
#39031=CARTESIAN_POINT('Ctrl Pts',(0.541934914920413,-0.38094122608036,
1.29160852566638));
#39032=CARTESIAN_POINT('Ctrl Pts',(0.658184137179402,-0.0748552690383927,
1.30353189578112));
#39033=CARTESIAN_POINT('Ctrl Pts',(0.613637036129002,0.24951805070619,1.31545526589586));
#39034=CARTESIAN_POINT('Ctrl Pts',(0.419176599763568,0.512933375740025,
1.3273786360106));
#39035=CARTESIAN_POINT('Ctrl Pts',(0.122310085445297,0.651037566301491,
1.33930200612534));
#39036=CARTESIAN_POINT('Ctrl Pts',(-0.204437142995836,0.630091361868343,
1.35122537624008));
#39037=CARTESIAN_POINT('Ctrl Pts',(-0.481239775259857,0.455211981877947,
1.36314874635482));
#39038=CARTESIAN_POINT('Ctrl Pts',(-0.640474112998224,0.169122973946595,
1.37507211646956));
#39039=CARTESIAN_POINT('Ctrl Pts',(-0.643238738497255,-0.15828327464979,
1.3869954865843));
#39040=CARTESIAN_POINT('Ctrl Pts',(-0.488858245604688,-0.447020453046308,
1.39891885669904));
#39041=CARTESIAN_POINT('Ctrl Pts',(-0.215048243442008,-0.626549218122459,
1.41084222681378));
#39042=CARTESIAN_POINT('Ctrl Pts',(0.111298677990423,-0.653010163791566,
1.42276559692852));
#39043=CARTESIAN_POINT('Ctrl Pts',(0.410455004573871,-0.519938803088884,
1.43468896704326));
#39044=CARTESIAN_POINT('Ctrl Pts',(0.60933596459771,-0.259844861379564,
1.44661233715801));
#39045=CARTESIAN_POINT('Ctrl Pts',(0.659354353749764,0.0637299453055676,
1.45853570727274));
#39046=CARTESIAN_POINT('Ctrl Pts',(0.548290532237762,0.371735338641693,
1.47045907738748));
#39047=CARTESIAN_POINT('Ctrl Pts',(0.303277718780669,0.5889246938542,1.48238244750222));
#39048=CARTESIAN_POINT('Ctrl Pts',(-0.0158267346391821,0.662238011746418,
1.49430581761697));
#39049=CARTESIAN_POINT('Ctrl Pts',(-0.331064670172572,0.573764632852262,
1.5062291877317));
#39050=CARTESIAN_POINT('Ctrl Pts',(-0.565422531671553,0.345118864162994,
1.51815255784645));
#39051=CARTESIAN_POINT('Ctrl Pts',(-0.661646003309974,0.032159540534428,
1.53007592796118));
#39052=CARTESIAN_POINT('Ctrl Pts',(-0.596227407535047,-0.288656453725316,
1.54199929807593));
#39053=CARTESIAN_POINT('Ctrl Pts',(-0.385148700011845,-0.538952825827497,
1.55392266819066));
#39054=CARTESIAN_POINT('Ctrl Pts',(-0.0799770306232885,-0.657581435785161,
1.56584603830541));
#39055=CARTESIAN_POINT('Ctrl Pts',(0.244733262815717,-0.615560962923072,
1.57776940842015));
#39056=CARTESIAN_POINT('Ctrl Pts',(0.509654499503361,-0.423157136223537,
1.58969277853489));
#39057=CARTESIAN_POINT('Ctrl Pts',(0.65006564047305,-0.127374769894107,
1.60161614864963));
#39058=CARTESIAN_POINT('Ctrl Pts',(0.631663831522472,0.199525618143451,
1.61353951876437));
#39059=CARTESIAN_POINT('Ctrl Pts',(0.458944686590344,0.477681329380949,
1.62546288887911));
#39060=CARTESIAN_POINT('Ctrl Pts',(0.174104005859975,0.639138046315416,
1.63738625899385));
#39061=CARTESIAN_POINT('Ctrl Pts',(-0.15327080207044,0.644451532827028,
1.64930962910859));
#39062=CARTESIAN_POINT('Ctrl Pts',(-0.4432010901377,0.49232345889988,1.66123299922333));
#39063=CARTESIAN_POINT('Ctrl Pts',(-0.624856069334877,0.219919618014252,
1.67315636933807));
#39064=CARTESIAN_POINT('Ctrl Pts',(-0.653856824902625,-0.106211838535058,
1.68507973945281));
#39065=CARTESIAN_POINT('Ctrl Pts',(-0.523118522761037,-0.406394225618784,
1.69700310956755));
#39066=CARTESIAN_POINT('Ctrl Pts',(-0.264580644698625,-0.607295703429515,
1.70892647968229));
#39067=CARTESIAN_POINT('Ctrl Pts',(0.058594705894833,-0.659828281778441,
1.72084984979703));
#39068=CARTESIAN_POINT('Ctrl Pts',(0.367455909925893,-0.551172362293768,
1.73277321991177));
#39069=CARTESIAN_POINT('Ctrl Pts',(0.586545138268328,-0.307844499110428,
1.74469659002651));
#39070=CARTESIAN_POINT('Ctrl Pts',(0.662342429399066,0.0106528333449858,
1.75661996014125));
#39071=CARTESIAN_POINT('Ctrl Pts',(0.576322538899538,0.326625513027934,
1.76854333025599));
#39072=CARTESIAN_POINT('Ctrl Pts',(0.425110290639966,0.483946614735963,
1.77649224366581));
#39073=CARTESIAN_POINT('Ctrl Pts',(0.33525021598174,0.539759624911124,1.78046670037073));
#39074=CARTESIAN_POINT('Ctrl Pts',(0.352184336898731,-0.494199469185471,
0.7));
#39075=CARTESIAN_POINT('Ctrl Pts',(0.434459481514031,-0.435567238565425,
0.703974456704914));
#39076=CARTESIAN_POINT('Ctrl Pts',(0.569074170603496,-0.276472369691842,
0.71192337011474));
#39077=CARTESIAN_POINT('Ctrl Pts',(0.63195675641648,0.0298991715734713,
0.72384674022948));
#39078=CARTESIAN_POINT('Ctrl Pts',(0.540450411763527,0.328891738414737,
0.73577011034422));
#39079=CARTESIAN_POINT('Ctrl Pts',(0.316910788923287,0.547571327639118,
0.747693480458961));
#39080=CARTESIAN_POINT('Ctrl Pts',(0.0159487222523762,0.632459517004967,
0.759616850573701));
#39081=CARTESIAN_POINT('Ctrl Pts',(-0.288909559125321,0.562845076658027,
0.771540220688441));
#39082=CARTESIAN_POINT('Ctrl Pts',(-0.523186437261898,0.355721357715825,
0.783463590803182));
#39083=CARTESIAN_POINT('Ctrl Pts',(-0.629647301151511,0.0616961589689892,
0.795386960917921));
#39084=CARTESIAN_POINT('Ctrl Pts',(-0.58228348821526,-0.247402746652621,
0.807310331032662));
#39085=CARTESIAN_POINT('Ctrl Pts',(-0.392666097338528,-0.496059852941866,
0.819233701147401));
#39086=CARTESIAN_POINT('Ctrl Pts',(-0.107119225715726,-0.623528367336511,
0.831157071262142));
#39087=CARTESIAN_POINT('Ctrl Pts',(0.204597189954239,-0.59866691871355,
0.843080441376881));
#39088=CARTESIAN_POINT('Ctrl Pts',(0.466329908650049,-0.427549452094589,
0.855003811491622));
#39089=CARTESIAN_POINT('Ctrl Pts',(0.614136857577049,-0.151980358083104,
0.866927181606362));
#39090=CARTESIAN_POINT('Ctrl Pts',(0.611908363121538,0.160717966477571,
0.878850551721102));
#39091=CARTESIAN_POINT('Ctrl Pts',(0.460188853366613,0.434152427784503,
0.890773921835841));
#39092=CARTESIAN_POINT('Ctrl Pts',(0.1960438512529,0.601522167555102,0.902697291950583));
#39093=CARTESIAN_POINT('Ctrl Pts',(-0.115995241116418,0.621938272442033,
0.914620662065322));
#39094=CARTESIAN_POINT('Ctrl Pts',(-0.399696354445721,0.490413024348575,
0.926544032180063));
#39095=CARTESIAN_POINT('Ctrl Pts',(-0.585750471122982,0.239078430553345,
0.938467402294802));
#39096=CARTESIAN_POINT('Ctrl Pts',(-0.628704022455928,-0.070663728299658,
0.950390772409543));
#39097=CARTESIAN_POINT('Ctrl Pts',(-0.518063329334561,-0.363142530047957,
0.962314142524282));
#39098=CARTESIAN_POINT('Ctrl Pts',(-0.280858238968939,-0.566904542191545,
0.974237512639023));
#39099=CARTESIAN_POINT('Ctrl Pts',(0.0249613464089441,-0.632170104895623,
0.986160882753763));
#39100=CARTESIAN_POINT('Ctrl Pts',(0.324682801338475,-0.542994649017271,
0.998084252868503));
#39101=CARTESIAN_POINT('Ctrl Pts',(0.545083291589825,-0.321164001053741,
1.01000762298324));
#39102=CARTESIAN_POINT('Ctrl Pts',(0.632318328233213,-0.0208720416904643,
1.02193099309798));
#39103=CARTESIAN_POINT('Ctrl Pts',(0.565076134877199,0.284519018936116,
1.03385436321272));
#39104=CARTESIAN_POINT('Ctrl Pts',(0.35978417741182,0.520401245221327,1.04577773332746));
#39105=CARTESIAN_POINT('Ctrl Pts',(0.0665958857068623,0.62914791452485,
1.0577011034422));
#39106=CARTESIAN_POINT('Ctrl Pts',(-0.242861977025874,0.584191895235632,
1.06962447355694));
#39107=CARTESIAN_POINT('Ctrl Pts',(-0.492987943452569,0.396516075278645,
1.08154784367169));
#39108=CARTESIAN_POINT('Ctrl Pts',(-0.622675503261414,0.111970210244065,
1.09347121378642));
#39109=CARTESIAN_POINT('Ctrl Pts',(-0.600241603613138,-0.199930306946909,
1.10539458390116));
#39110=CARTESIAN_POINT('Ctrl Pts',(-0.431166912267969,-0.462987261281848,
1.1173179540159));
#39111=CARTESIAN_POINT('Ctrl Pts',(-0.156756874309222,-0.612935064016377,
1.12924132413064));
#39112=CARTESIAN_POINT('Ctrl Pts',(0.155949329750418,-0.613141025290557,
1.14116469424539));
#39113=CARTESIAN_POINT('Ctrl Pts',(0.4305566532234,-0.463554828158465,1.15308806436012));
#39114=CARTESIAN_POINT('Ctrl Pts',(0.59997771816483,-0.200720821166321,
1.16501143447486));
#39115=CARTESIAN_POINT('Ctrl Pts',(0.622822459401631,0.111149873634038,
1.17693480458961));
#39116=CARTESIAN_POINT('Ctrl Pts',(0.493509839363413,0.395866326927988,
1.18885817470434));
#39117=CARTESIAN_POINT('Ctrl Pts',(0.243631311999152,0.583871470580239,
1.20078154481908));
#39118=CARTESIAN_POINT('Ctrl Pts',(-0.0657670624710998,0.629235094251649,
1.21270491493383));
#39119=CARTESIAN_POINT('Ctrl Pts',(-0.359098349871265,0.520874731066591,
1.22462828504856));
#39120=CARTESIAN_POINT('Ctrl Pts',(-0.564700852720018,0.285263136912645,
1.23655165516331));
#39121=CARTESIAN_POINT('Ctrl Pts',(-0.632345273995765,-0.020039081794827,
1.24847502527805));
#39122=CARTESIAN_POINT('Ctrl Pts',(-0.545505882342923,-0.320445693797292,
1.26039839539279));
#39123=CARTESIAN_POINT('Ctrl Pts',(-0.325397796916506,-0.542566478973631,
1.27232176550753));
#39124=CARTESIAN_POINT('Ctrl Pts',(-0.0257940712861588,-0.632136675277145,
1.28424513562227));
#39125=CARTESIAN_POINT('Ctrl Pts',(0.280111221932506,-0.567274019933433,
1.29616850573701));
#39126=CARTESIAN_POINT('Ctrl Pts',(0.517584518601595,-0.363824650687545,
1.30809187585175));
#39127=CARTESIAN_POINT('Ctrl Pts',(0.628610392897891,-0.0714918476801203,
1.32001524596649));
#39128=CARTESIAN_POINT('Ctrl Pts',(0.586064896718421,0.238306624285571,
1.33193861608123));
#39129=CARTESIAN_POINT('Ctrl Pts',(0.4003420200921,0.489886086036881,1.34386198619597));
#39130=CARTESIAN_POINT('Ctrl Pts',(0.116814408801508,0.621784934073119,
1.35578535631071));
#39131=CARTESIAN_POINT('Ctrl Pts',(-0.195251306621063,0.601779891327988,
1.36770872642545));
#39132=CARTESIAN_POINT('Ctrl Pts',(-0.459616552748575,0.434758248666402,
1.37963209654019));
#39133=CARTESIAN_POINT('Ctrl Pts',(-0.611696121298351,0.161523885331273,
1.39155546665493));
#39134=CARTESIAN_POINT('Ctrl Pts',(-0.614336525742933,-0.151171238938032,
1.40347883676967));
#39135=CARTESIAN_POINT('Ctrl Pts',(-0.466892707499535,-0.426934784279433,
1.41540220688441));
#39136=CARTESIAN_POINT('Ctrl Pts',(-0.205385625641773,-0.598396904339966,
1.42732557699915));
#39137=CARTESIAN_POINT('Ctrl Pts',(0.106297769497149,-0.623668898169518,
1.43924894711389));
#39138=CARTESIAN_POINT('Ctrl Pts',(0.392012306461527,-0.496576743239674,
1.45117231722863));
#39139=CARTESIAN_POINT('Ctrl Pts',(0.581957082335726,-0.248169427334259,
1.46309568734337));
#39140=CARTESIAN_POINT('Ctrl Pts',(0.629728028915714,0.0608664106211582,
1.47501905745811));
#39141=CARTESIAN_POINT('Ctrl Pts',(0.523654563249111,0.355032405185257,
1.48694242757285));
#39142=CARTESIAN_POINT('Ctrl Pts',(0.289650745423433,0.562462937465252,
1.49886579768759));
#39143=CARTESIAN_POINT('Ctrl Pts',(-0.0151156026373754,0.632482117450919,
1.51078916780233));
#39144=CARTESIAN_POINT('Ctrl Pts',(-0.316189164454242,0.547984053267855,
1.52271253791707));
#39145=CARTESIAN_POINT('Ctrl Pts',(-0.540016782097706,0.329611870817301,
1.53463590803181));
#39146=CARTESIAN_POINT('Ctrl Pts',(-0.631916709330591,0.0307145375721074,
1.54655927814655));
#39147=CARTESIAN_POINT('Ctrl Pts',(-0.569437523233623,-0.275686447817451,
1.55848264826129));
#39148=CARTESIAN_POINT('Ctrl Pts',(-0.367843073028309,-0.514736421708243,
1.57040601837603));
#39149=CARTESIAN_POINT('Ctrl Pts',(-0.0763834766033089,-0.628034772279233,
1.58232938849077));
#39150=CARTESIAN_POINT('Ctrl Pts',(0.233736828044883,-0.5879023770064,1.59425275860551));
#39151=CARTESIAN_POINT('Ctrl Pts',(0.486754537336504,-0.404143701789823,
1.60617612872025));
#39152=CARTESIAN_POINT('Ctrl Pts',(0.620856679132942,-0.121651525197101,
1.61809949883499));
#39153=CARTESIAN_POINT('Ctrl Pts',(0.603281706262845,0.190560468004963,
1.63002286894973));
#39154=CARTESIAN_POINT('Ctrl Pts',(0.43832323427345,0.456217996120286,1.64194623906447));
#39155=CARTESIAN_POINT('Ctrl Pts',(0.166281107894437,0.610420087199418,
1.65386960917921));
#39156=CARTESIAN_POINT('Ctrl Pts',(-0.146383988411153,0.615494826402396,
1.66579297929395));
#39157=CARTESIAN_POINT('Ctrl Pts',(-0.423287034230507,0.470202220700963,
1.67771634940869));
#39158=CARTESIAN_POINT('Ctrl Pts',(-0.596779832665833,0.210038118023212,
1.68963971952343));
#39159=CARTESIAN_POINT('Ctrl Pts',(-0.624477516827445,-0.101439493570979,
1.70156308963817));
#39160=CARTESIAN_POINT('Ctrl Pts',(-0.499613590710631,-0.388133987750645,
1.71348645975291));
#39161=CARTESIAN_POINT('Ctrl Pts',(-0.252692420892918,-0.580008494847657,
1.72540982986765));
#39162=CARTESIAN_POINT('Ctrl Pts',(0.0559619094621963,-0.630180662255662,
1.73733319998239));
#39163=CARTESIAN_POINT('Ctrl Pts',(0.350945261156011,-0.526406905977294,
1.74925657009713));
#39164=CARTESIAN_POINT('Ctrl Pts',(0.560190300846922,-0.294012329690215,
1.76117994021187));
#39165=CARTESIAN_POINT('Ctrl Pts',(0.632581843375548,0.0101741767633066,
1.77310331032661));
#39166=CARTESIAN_POINT('Ctrl Pts',(0.550427026646497,0.311949468966009,
1.78502668044135));
#39167=CARTESIAN_POINT('Ctrl Pts',(0.406009096435101,0.462201767630657,
1.79297559385118));
#39168=CARTESIAN_POINT('Ctrl Pts',(0.320186643954231,0.515506969432351,
1.79695005055609));
#39169=CARTESIAN_POINT('Ctrl Pts',(0.301912013981581,0.623256720988311,
0.7));
#39170=CARTESIAN_POINT('Ctrl Pts',(0.316742913732564,0.614965173301012,
0.7));
#39171=CARTESIAN_POINT('Ctrl Pts',(0.3312465938099,0.606134971871919,0.7));
#39172=CARTESIAN_POINT('Ctrl Pts',(0.345390045352,0.596775580586543,0.7));
#39173=CARTESIAN_POINT('Ctrl Pts',(0.368996263743943,0.581154228610288,
0.7));
#39174=CARTESIAN_POINT('Ctrl Pts',(0.391600130077927,0.564059572920914,
0.7));
#39175=CARTESIAN_POINT('Ctrl Pts',(0.413087355494181,0.545611767070564,
0.7));
#39176=CARTESIAN_POINT('Ctrl Pts',(0.421816954375618,0.538116990886276,
0.7));
#39177=CARTESIAN_POINT('Ctrl Pts',(0.430362017243965,0.530398662168233,
0.7));
#39178=CARTESIAN_POINT('Ctrl Pts',(0.438713852739663,0.522464087423267,
0.7));
#39179=CARTESIAN_POINT('Ctrl Pts',(0.445012055142894,0.51648054551166,0.7));
#39180=CARTESIAN_POINT('Ctrl Pts',(0.451200223788741,0.510373897616862,
0.7));
#39181=CARTESIAN_POINT('Ctrl Pts',(0.457264688892812,0.504157868673923,
0.7));
#39182=CARTESIAN_POINT('Ctrl Pts',(0.479903218716829,0.480953553998711,
0.7));
#39183=CARTESIAN_POINT('Ctrl Pts',(0.500858312621123,0.456192563010338,
0.7));
#39184=CARTESIAN_POINT('Ctrl Pts',(0.519950046261114,0.430052281971842,
0.7));
#39185=CARTESIAN_POINT('Ctrl Pts',(0.532066948364594,0.413461896191609,
0.7));
#39186=CARTESIAN_POINT('Ctrl Pts',(0.543432537348295,0.396315311298811,
0.7));
#39187=CARTESIAN_POINT('Ctrl Pts',(0.553991354258157,0.378653559125833,
0.7));
#39188=CARTESIAN_POINT('Ctrl Pts',(0.557760895560471,0.372348240560731,
0.7));
#39189=CARTESIAN_POINT('Ctrl Pts',(0.561422494384538,0.365985667439434,
0.7));
#39190=CARTESIAN_POINT('Ctrl Pts',(0.564974116622367,0.359568344749639,
0.7));
#39191=CARTESIAN_POINT('Ctrl Pts',(0.567149078484655,0.355638469562003,
0.7));
#39192=CARTESIAN_POINT('Ctrl Pts',(0.569282819078203,0.351688020934708,
0.7));
#39193=CARTESIAN_POINT('Ctrl Pts',(0.571374893992065,0.347717486836035,
0.7));
#39194=CARTESIAN_POINT('Ctrl Pts',(0.586516887221463,0.318979605586734,
0.7));
#39195=CARTESIAN_POINT('Ctrl Pts',(0.599480260131589,0.289191109124012,
0.7));
#39196=CARTESIAN_POINT('Ctrl Pts',(0.610215113049288,0.258612759249907,
0.7));
#39197=CARTESIAN_POINT('Ctrl Pts',(0.620862381399234,0.228283895007034,
0.7));
#39198=CARTESIAN_POINT('Ctrl Pts',(0.62931749648762,0.197176730970088,0.7));
#39199=CARTESIAN_POINT('Ctrl Pts',(0.635481674913492,0.165538333607963,
0.7));
#39200=CARTESIAN_POINT('Ctrl Pts',(0.637058860844219,0.157443234514,0.7));
#39201=CARTESIAN_POINT('Ctrl Pts',(0.638485804480818,0.149313374621512,
0.7));
#39202=CARTESIAN_POINT('Ctrl Pts',(0.639760298594453,0.141152968773294,
0.7));
#39203=CARTESIAN_POINT('Ctrl Pts',(0.640724273662108,0.134980772530509,
0.7));
#39204=CARTESIAN_POINT('Ctrl Pts',(0.641600510210609,0.128793923527105,
0.7));
#39205=CARTESIAN_POINT('Ctrl Pts',(0.642387398557739,0.122602557207706,
0.7));
#39206=CARTESIAN_POINT('Ctrl Pts',(0.646272029071298,0.0920376484596141,
0.7));
#39207=CARTESIAN_POINT('Ctrl Pts',(0.647992252287009,0.0613038392021154,
0.7));
#39208=CARTESIAN_POINT('Ctrl Pts',(0.647486512817817,0.0306206514007389,
0.7));
#39209=CARTESIAN_POINT('Ctrl Pts',(0.647048570692616,0.00405072500145474,
0.7));
#39210=CARTESIAN_POINT('Ctrl Pts',(0.644940626982976,-0.022481795837132,
0.7));
#39211=CARTESIAN_POINT('Ctrl Pts',(0.641195095628098,-0.0488246644619669,
0.7));
#39212=CARTESIAN_POINT('Ctrl Pts',(0.639088886165721,-0.0636379429815907,
0.7));
#39213=CARTESIAN_POINT('Ctrl Pts',(0.636464411497198,-0.0783911345254818,
0.7));
#39214=CARTESIAN_POINT('Ctrl Pts',(0.633324220155005,-0.0930556586801398,
0.7));
#39215=CARTESIAN_POINT('Ctrl Pts',(0.631822561842711,-0.100068321984061,
0.7));
#39216=CARTESIAN_POINT('Ctrl Pts',(0.630202465201574,-0.107062563306399,
0.7));
#39217=CARTESIAN_POINT('Ctrl Pts',(0.628465525090794,-0.114029195569243,
0.7));
#39218=CARTESIAN_POINT('Ctrl Pts',(0.620900031829999,-0.144373367546085,
0.7));
#39219=CARTESIAN_POINT('Ctrl Pts',(0.61115833403686,-0.174053594627863,
0.7));
#39220=CARTESIAN_POINT('Ctrl Pts',(0.599311626004954,-0.202827697227785,
0.7));
#39221=CARTESIAN_POINT('Ctrl Pts',(0.589222460913586,-0.227332958158054,
0.7));
#39222=CARTESIAN_POINT('Ctrl Pts',(0.577605524722755,-0.251181291846326,
0.7));
#39223=CARTESIAN_POINT('Ctrl Pts',(0.564478637188341,-0.274208720129379,
0.7));
#39224=CARTESIAN_POINT('Ctrl Pts',(0.556929094299622,-0.28745226754182,
0.7));
#39225=CARTESIAN_POINT('Ctrl Pts',(0.548879654511669,-0.300423975832763,
0.7));
#39226=CARTESIAN_POINT('Ctrl Pts',(0.540348752462322,-0.313098885409112,
0.7));
#39227=CARTESIAN_POINT('Ctrl Pts',(0.536443758105698,-0.318900786553921,
0.7));
#39228=CARTESIAN_POINT('Ctrl Pts',(0.532437857208379,-0.324640465844469,
0.7));
#39229=CARTESIAN_POINT('Ctrl Pts',(0.528332704252445,-0.330315351774545,
0.7));
#39230=CARTESIAN_POINT('Ctrl Pts',(0.524569485757922,-0.335517553961799,
0.7));
#39231=CARTESIAN_POINT('Ctrl Pts',(0.520725138073348,-0.340662013706015,
0.7));
#39232=CARTESIAN_POINT('Ctrl Pts',(0.516806355023409,-0.345740598709291,
0.7));
#39233=CARTESIAN_POINT('Ctrl Pts',(0.498042718044497,-0.37005751652629,
0.7));
#39234=CARTESIAN_POINT('Ctrl Pts',(0.477542558449122,-0.392913064495779,
0.7));
#39235=CARTESIAN_POINT('Ctrl Pts',(0.455486881988334,-0.414130436631542,
0.7));
#39236=CARTESIAN_POINT('Ctrl Pts',(0.433826821014111,-0.434967230052523,
0.7));
#39237=CARTESIAN_POINT('Ctrl Pts',(0.410665525050054,-0.454224782213852,
0.7));
#39238=CARTESIAN_POINT('Ctrl Pts',(0.386146686004952,-0.471694960933986,
0.7));
#39239=CARTESIAN_POINT('Ctrl Pts',(0.375097833815722,-0.479567496091263,
0.7));
#39240=CARTESIAN_POINT('Ctrl Pts',(0.363773025729378,-0.487076461755432,
0.7));
#39241=CARTESIAN_POINT('Ctrl Pts',(0.352184336898733,-0.494199469185469,
0.7));
#39242=CARTESIAN_POINT('Ctrl Pts',(0.365377360036757,0.58826493586867,1.7475));
#39243=CARTESIAN_POINT('Ctrl Pts',(0.463312679049696,0.527436308946575,
1.74352554329509));
#39244=CARTESIAN_POINT('Ctrl Pts',(0.545713121227658,0.441706955049179,
1.73955108659017));
#39245=CARTESIAN_POINT('Ctrl Pts',(0.602538348656719,0.341447702326575,
1.73557662988526));
#39246=CARTESIAN_POINT('Ctrl Pts',(0.65936357608578,0.241188449603971,1.73160217318035));
#39247=CARTESIAN_POINT('Ctrl Pts',(0.690613588765941,0.126399298056159,
1.72762771647543));
#39248=CARTESIAN_POINT('Ctrl Pts',(0.69247046371686,0.0111515582057199,
1.72365325977052));
#39249=CARTESIAN_POINT('Ctrl Pts',(0.69432733866778,-0.10409618164472,1.71967880306561));
#39250=CARTESIAN_POINT('Ctrl Pts',(0.666791075889459,-0.219802509797787,
1.71570434636069));
#39251=CARTESIAN_POINT('Ctrl Pts',(0.613226676892718,-0.32185474670363,
1.71172988965578));
#39252=CARTESIAN_POINT('Ctrl Pts',(0.559662277895978,-0.423906983609474,
1.70775543295087));
#39253=CARTESIAN_POINT('Ctrl Pts',(0.480069742680819,-0.512305129268094,
1.70378097624595));
#39254=CARTESIAN_POINT('Ctrl Pts',(0.384170656955648,-0.576240909746952,
1.69980651954104));
#39255=CARTESIAN_POINT('Ctrl Pts',(0.288271571230476,-0.64017669022581,
1.69583206283613));
#39256=CARTESIAN_POINT('Ctrl Pts',(0.176065934995291,-0.679650105524906,
1.69185760613121));
#39257=CARTESIAN_POINT('Ctrl Pts',(0.0612602183660074,-0.689844579802659,
1.6878831494263));
#39258=CARTESIAN_POINT('Ctrl Pts',(-0.0535454982632758,-0.700039054080412,
1.68390869272139));
#39259=CARTESIAN_POINT('Ctrl Pts',(-0.170951295286657,-0.680954587336821,
1.67993423601647));
#39260=CARTESIAN_POINT('Ctrl Pts',(-0.276616076223649,-0.634919784091998,
1.67595977931156));
#39261=CARTESIAN_POINT('Ctrl Pts',(-0.382280857160642,-0.588884980847175,
1.67198532260665));
#39262=CARTESIAN_POINT('Ctrl Pts',(-0.476204622011245,-0.515899841101119,
1.66801086590173));
#39263=CARTESIAN_POINT('Ctrl Pts',(-0.546914346801737,-0.42488090907945,
1.66403640919682));
#39264=CARTESIAN_POINT('Ctrl Pts',(-0.617624071592228,-0.333861977057781,
1.66006195249191));
#39265=CARTESIAN_POINT('Ctrl Pts',(-0.665119756322608,-0.224809252760498,
1.65608749578699));
#39266=CARTESIAN_POINT('Ctrl Pts',(-0.683599782291128,-0.111043032868598,
1.65211303908208));
#39267=CARTESIAN_POINT('Ctrl Pts',(-0.689558148768936,-0.0743623035197568,
1.65083158690023));
#39268=CARTESIAN_POINT('Ctrl Pts',(-0.692500165449594,-0.0371915783518519,
1.64955013471837));
#39269=CARTESIAN_POINT('Ctrl Pts',(-0.692468966846601,-1.59520066716212E-5,
1.64826868253652));
#39270=CARTESIAN_POINT('Origin',(0.,0.,0.895));
#39271=CARTESIAN_POINT('Origin',(0.,0.,1.7475));
#39272=CARTESIAN_POINT('Ctrl Pts',(0.6516,1.70379184550113E-15,-0.72625));
#39273=CARTESIAN_POINT('Ctrl Pts',(0.6516,0.10591743302354,-0.722791509249761));
#39274=CARTESIAN_POINT('Ctrl Pts',(0.598993916001074,0.317654812761972,
-0.715874527749282));
#39275=CARTESIAN_POINT('Ctrl Pts',(0.380287460438119,0.561300167265437,
-0.705499055498563));
#39276=CARTESIAN_POINT('Ctrl Pts',(0.0729856334338192,0.674050219639796,
-0.695123583247845));
#39277=CARTESIAN_POINT('Ctrl Pts',(-0.251359967211615,0.629681615150501,
-0.684748110997127));
#39278=CARTESIAN_POINT('Ctrl Pts',(-0.517092446119555,0.438507275576915,
-0.674372638746409));
#39279=CARTESIAN_POINT('Ctrl Pts',(-0.662284183342424,0.145110368978899,
-0.66399716649569));
#39280=CARTESIAN_POINT('Ctrl Pts',(-0.653076224636751,-0.182118205164697,
-0.653621694244972));
#39281=CARTESIAN_POINT('Ctrl Pts',(-0.491620673403516,-0.4668888850725,
-0.643246221994254));
#39282=CARTESIAN_POINT('Ctrl Pts',(-0.215554351760434,-0.64281600898939,
-0.632870749743535));
#39283=CARTESIAN_POINT('Ctrl Pts',(0.110762954559402,-0.668885305138704,
-0.622495277492817));
#39284=CARTESIAN_POINT('Ctrl Pts',(0.411258705600379,-0.539019822036371,
-0.612119805242099));
#39285=CARTESIAN_POINT('Ctrl Pts',(0.615879002840427,-0.283494407102116,
-0.60174433299138));
#39286=CARTESIAN_POINT('Ctrl Pts',(0.676921592558105,0.0381210480060534,
-0.591368860740662));
#39287=CARTESIAN_POINT('Ctrl Pts',(0.580155735567945,0.350849494573475,
-0.580993388489943));
#39288=CARTESIAN_POINT('Ctrl Pts',(0.348140170063391,0.581785587179681,
-0.570617916239225));
#39289=CARTESIAN_POINT('Ctrl Pts',(0.0349638692286564,0.677091999899065,
-0.560242443988507));
#39290=CARTESIAN_POINT('Ctrl Pts',(-0.286363435133131,0.614550266504086,
-0.549866971737789));
#39291=CARTESIAN_POINT('Ctrl Pts',(-0.540931812645454,0.408740531547555,
-0.53949149948707));
#39292=CARTESIAN_POINT('Ctrl Pts',(-0.669394604785241,0.107642512990995,
-0.529116027236352));
#39293=CARTESIAN_POINT('Ctrl Pts',(-0.641803721387148,-0.218549836322835,
-0.518740554985634));
#39294=CARTESIAN_POINT('Ctrl Pts',(-0.464591330058565,-0.493792409536047,
-0.508365082734915));
#39295=CARTESIAN_POINT('Ctrl Pts',(-0.179070350189228,-0.653918846159451,
-0.497989610484197));
#39296=CARTESIAN_POINT('Ctrl Pts',(0.148196688364544,-0.661599417513598,
-0.487614138233479));
#39297=CARTESIAN_POINT('Ctrl Pts',(0.440915139510084,-0.51504357818782,
-0.477238665982761));
#39298=CARTESIAN_POINT('Ctrl Pts',(0.630844551378487,-0.248417390064856,
-0.466863193732042));
#39299=CARTESIAN_POINT('Ctrl Pts',(0.673707329393678,0.0761214950437051,
-0.456487721481324));
#39300=CARTESIAN_POINT('Ctrl Pts',(0.559511020646667,0.382914436216214,
-0.446112249230605));
#39301=CARTESIAN_POINT('Ctrl Pts',(0.31487782023221,0.600439843792433,-0.435736776979887));
#39302=CARTESIAN_POINT('Ctrl Pts',(-0.00316177006436105,0.677986763069525,
-0.425361304729169));
#39303=CARTESIAN_POINT('Ctrl Pts',(-0.320464267714219,0.597476945836541,
-0.414985832478451));
#39304=CARTESIAN_POINT('Ctrl Pts',(-0.56305802607539,0.377679370577104,
-0.404610360227732));
#39305=CARTESIAN_POINT('Ctrl Pts',(-0.674387991520381,0.0698346946780471,
-0.394234887977014));
#39306=CARTESIAN_POINT('Ctrl Pts',(-0.628500189764246,-0.254290304876461,
-0.383859415726295));
#39307=CARTESIAN_POINT('Ctrl Pts',(-0.436092287172216,-0.519133474893842,
-0.373483943475578));
#39308=CARTESIAN_POINT('Ctrl Pts',(-0.142019680366899,-0.662952832469283,
-0.363108471224859));
#39309=CARTESIAN_POINT('Ctrl Pts',(0.185161489055837,-0.652220262374863,
-0.352732998974141));
#39310=CARTESIAN_POINT('Ctrl Pts',(0.469176593473532,-0.489437812018158,
-0.342357526723422));
#39311=CARTESIAN_POINT('Ctrl Pts',(0.643814162441103,-0.212554397554274,
-0.331982054472704));
#39312=CARTESIAN_POINT('Ctrl Pts',(0.668361536472565,0.113881096960973,
-0.321606582221986));
#39313=CARTESIAN_POINT('Ctrl Pts',(0.537096070163569,0.413767880771309,
-0.311231109971268));
#39314=CARTESIAN_POINT('Ctrl Pts',(0.280619232983065,0.617194372623894,
-0.300855637720549));
#39315=CARTESIAN_POINT('Ctrl Pts',(-0.0412774067590903,0.676736450734642,
-0.290480165469831));
#39316=CARTESIAN_POINT('Ctrl Pts',(-0.353551185726935,0.578513272200878,
-0.280104693219112));
#39317=CARTESIAN_POINT('Ctrl Pts',(-0.583402785381157,0.345423274387037,
-0.269729220968394));
#39318=CARTESIAN_POINT('Ctrl Pts',(-0.677247687787472,0.031805924735722,
-0.259353748717676));
#39319=CARTESIAN_POINT('Ctrl Pts',(-0.613208152053947,-0.289226222202328,
-0.248978276466957));
#39320=CARTESIAN_POINT('Ctrl Pts',(-0.406213495413166,-0.542832066956897,
-0.238602804216239));
#39321=CARTESIAN_POINT('Ctrl Pts',(-0.104519676240231,-0.669889291059751,
-0.228227331965521));
#39322=CARTESIAN_POINT('Ctrl Pts',(0.221540459947147,-0.640777587066391,
-0.217851859714803));
#39323=CARTESIAN_POINT('Ctrl Pts',(0.49595362168121,-0.462283450573905,
-0.207476387464084));
#39324=CARTESIAN_POINT('Ctrl Pts',(0.654746819495382,-0.176019039699093,
-0.197100915213366));
#39325=CARTESIAN_POINT('Ctrl Pts',(0.66090111234246,0.151280657145806,-0.186725442962648));
#39326=CARTESIAN_POINT('Ctrl Pts',(0.51298182194067,0.443311680645382,-0.176349970711929));
#39327=CARTESIAN_POINT('Ctrl Pts',(0.245472765512694,0.631997215248837,
-0.165974498461211));
#39328=CARTESIAN_POINT('Ctrl Pts',(-0.0792623836862046,0.673342931276607,
-0.155599026210492));
#39329=CARTESIAN_POINT('Ctrl Pts',(-0.385519630244667,0.557723394050477,
-0.145223553959774));
#39330=CARTESIAN_POINT('Ctrl Pts',(-0.601901478794571,0.312066036455591,
-0.134848081709056));
#39331=CARTESIAN_POINT('Ctrl Pts',(-0.677965082858782,-0.00630688219070944,
-0.124472609458338));
#39332=CARTESIAN_POINT('Ctrl Pts',(-0.595975637420361,-0.323282123041996,
-0.114097137207619));
#39333=CARTESIAN_POINT('Ctrl Pts',(-0.448685015420264,-0.484234261030354,
-0.10718015570714));
#39334=CARTESIAN_POINT('Ctrl Pts',(-0.360448909728228,-0.542825150002956,
-0.103721664956901));
#39335=CARTESIAN_POINT('Ctrl Pts',(0.6516,1.70379184550113E-15,-0.729109831226506));
#39336=CARTESIAN_POINT('Ctrl Pts',(0.6516,0.105917843960459,-0.725651340476266));
#39337=CARTESIAN_POINT('Ctrl Pts',(0.598993966183392,0.317654580582479,
-0.718734358975788));
#39338=CARTESIAN_POINT('Ctrl Pts',(0.380287471156537,0.561300312828727,
-0.708358886725069));
#39339=CARTESIAN_POINT('Ctrl Pts',(0.0729856416697512,0.674050196632246,
-0.697983414474351));
#39340=CARTESIAN_POINT('Ctrl Pts',(-0.251359982464231,0.629681676831451,
-0.687607942223633));
#39341=CARTESIAN_POINT('Ctrl Pts',(-0.517092471768115,0.438507283657801,
-0.677232469972914));
#39342=CARTESIAN_POINT('Ctrl Pts',(-0.662284218200291,0.145110383849344,
-0.666856997722196));
#39343=CARTESIAN_POINT('Ctrl Pts',(-0.653076258166858,-0.182118218295592,
-0.656481525471477));
#39344=CARTESIAN_POINT('Ctrl Pts',(-0.491620699001913,-0.466888907385001,
-0.64610605322076));
#39345=CARTESIAN_POINT('Ctrl Pts',(-0.215554362849302,-0.642816043209853,
-0.635730580970041));
#39346=CARTESIAN_POINT('Ctrl Pts',(0.11076296025821,-0.668885339300916,
-0.625355108719322));
#39347=CARTESIAN_POINT('Ctrl Pts',(0.411258726912751,-0.539019850182803,
-0.614979636468604));
#39348=CARTESIAN_POINT('Ctrl Pts',(0.615879034720188,-0.283494421661586,
-0.604604164217886));
#39349=CARTESIAN_POINT('Ctrl Pts',(0.676921627612323,0.0381210499198712,
-0.594228691967168));
#39350=CARTESIAN_POINT('Ctrl Pts',(0.580155765604886,0.350849512769928,
-0.583853219716449));
#39351=CARTESIAN_POINT('Ctrl Pts',(0.348140188090538,0.581785617288146,
-0.573477747465732));
#39352=CARTESIAN_POINT('Ctrl Pts',(0.0349638710384253,0.677092034965131,
-0.563102275215012));
#39353=CARTESIAN_POINT('Ctrl Pts',(-0.286363449960142,0.614550298320383,
-0.552726802964295));
#39354=CARTESIAN_POINT('Ctrl Pts',(-0.540931840653934,0.408740552713229,
-0.542351330713575));
#39355=CARTESIAN_POINT('Ctrl Pts',(-0.669394639445035,0.107642518563529,
-0.531975858462859));
#39356=CARTESIAN_POINT('Ctrl Pts',(-0.641803754618455,-0.218549847638404,
-0.521600386212139));
#39357=CARTESIAN_POINT('Ctrl Pts',(-0.464591354114125,-0.493792435103844,
-0.511224913961421));
#39358=CARTESIAN_POINT('Ctrl Pts',(-0.17907035946113,-0.653918880017893,
-0.500849441710703));
#39359=CARTESIAN_POINT('Ctrl Pts',(0.148196696037867,-0.66159945176991,
-0.490473969459984));
#39360=CARTESIAN_POINT('Ctrl Pts',(0.440915162339756,-0.51504360485568,
-0.480098497209267));
#39361=CARTESIAN_POINT('Ctrl Pts',(0.630844584042316,-0.248417402927411,
-0.469723024958547));
#39362=CARTESIAN_POINT('Ctrl Pts',(0.67370736427685,0.0761214989851266,
-0.45934755270783));
#39363=CARTESIAN_POINT('Ctrl Pts',(0.559511049616991,0.382914456042728,
-0.448972080457111));
#39364=CARTESIAN_POINT('Ctrl Pts',(0.314877836535932,0.600439874881969,
-0.438596608206393));
#39365=CARTESIAN_POINT('Ctrl Pts',(-0.00316177022807097,0.677986798174277,
-0.428221135955674));
#39366=CARTESIAN_POINT('Ctrl Pts',(-0.320464284307196,0.597476976772663,
-0.417845663704957));
#39367=CARTESIAN_POINT('Ctrl Pts',(-0.563058055229369,0.37767939013256,
-0.407470191454237));
#39368=CARTESIAN_POINT('Ctrl Pts',(-0.674388026438798,0.0698346982939447,
-0.39709471920352));
#39369=CARTESIAN_POINT('Ctrl Pts',(-0.628500222306683,-0.25429031804309,
-0.386719246952801));
#39370=CARTESIAN_POINT('Ctrl Pts',(-0.436092309752179,-0.519133501773496,
-0.376343774702083));
#39371=CARTESIAN_POINT('Ctrl Pts',(-0.142019687720371,-0.662952866795619,
-0.365968302451365));
#39372=CARTESIAN_POINT('Ctrl Pts',(0.185161498643091,-0.652220296145461,
-0.355592830200646));
#39373=CARTESIAN_POINT('Ctrl Pts',(0.469176617766576,-0.489437837360274,
-0.345217357949928));
#39374=CARTESIAN_POINT('Ctrl Pts',(0.643814195776372,-0.212554408559825,
-0.33484188569921));
#39375=CARTESIAN_POINT('Ctrl Pts',(0.668361571079138,0.113881102857349,
-0.324466413448491));
#39376=CARTESIAN_POINT('Ctrl Pts',(0.537096097972906,0.413767902195657,
-0.314090941197774));
#39377=CARTESIAN_POINT('Ctrl Pts',(0.280619247513718,0.617194404580342,
-0.303715468947054));
#39378=CARTESIAN_POINT('Ctrl Pts',(-0.0412774088978781,0.67673648577585,
-0.293339996696337));
#39379=CARTESIAN_POINT('Ctrl Pts',(-0.353551204030045,0.578513302152726,
-0.282964524445618));
#39380=CARTESIAN_POINT('Ctrl Pts',(-0.583402815594588,0.345423292277057,
-0.2725890521949));
#39381=CARTESIAN_POINT('Ctrl Pts',(-0.67724772284195,0.0318059263731912,
-0.262213579944181));
#39382=CARTESIAN_POINT('Ctrl Pts',(-0.613208183828464,-0.289226237159228,
-0.251838107693463));
#39383=CARTESIAN_POINT('Ctrl Pts',(-0.406213516398622,-0.542832095100663,
-0.241462635442745));
#39384=CARTESIAN_POINT('Ctrl Pts',(-0.104519681746337,-0.669889325671602,
-0.231087163192027));
#39385=CARTESIAN_POINT('Ctrl Pts',(0.221540471605481,-0.640777620390888,
-0.220711690941308));
#39386=CARTESIAN_POINT('Ctrl Pts',(0.495953646988114,-0.462283474219069,
-0.21033621869059));
#39387=CARTESIAN_POINT('Ctrl Pts',(0.654746854137338,-0.176019049391254,
-0.199960746439871));
#39388=CARTESIAN_POINT('Ctrl Pts',(0.66090114509062,0.151280666128215,-0.189585274189154));
#39389=CARTESIAN_POINT('Ctrl Pts',(0.51298185142758,0.443311701314457,-0.179209801938435));
#39390=CARTESIAN_POINT('Ctrl Pts',(0.245472772407152,0.631997252513665,
-0.168834329687717));
#39391=CARTESIAN_POINT('Ctrl Pts',(-0.0792623762299619,0.67334295711367,
-0.158458857436998));
#39392=CARTESIAN_POINT('Ctrl Pts',(-0.38551967319154,0.557723440877264,
-0.14808338518628));
#39393=CARTESIAN_POINT('Ctrl Pts',(-0.601901464183699,0.31206601686732,
-0.137707912935562));
#39394=CARTESIAN_POINT('Ctrl Pts',(-0.677965210051624,-0.00630681059785788,
-0.127332440684844));
#39395=CARTESIAN_POINT('Ctrl Pts',(-0.595975471759363,-0.323282293283048,
-0.116956968434125));
#39396=CARTESIAN_POINT('Ctrl Pts',(-0.448685357757425,-0.484234033710274,
-0.110039986933646));
#39397=CARTESIAN_POINT('Ctrl Pts',(-0.360448909728228,-0.542825150002956,
-0.106581496183407));
#39398=CARTESIAN_POINT('Ctrl Pts',(0.650016727545913,1.69965193344392E-15,
-0.735787069985478));
#39399=CARTESIAN_POINT('Ctrl Pts',(0.650016727545912,0.10565929404003,-0.732328579235239));
#39400=CARTESIAN_POINT('Ctrl Pts',(0.597538371946512,0.316883407693635,
-0.72541159773476));
#39401=CARTESIAN_POINT('Ctrl Pts',(0.379363409041282,0.559936031664057,
-0.715036125484042));
#39402=CARTESIAN_POINT('Ctrl Pts',(0.0728082756862247,0.672412440714268,
-0.704660653233323));
#39403=CARTESIAN_POINT('Ctrl Pts',(-0.250749178172313,0.628151483647856,
-0.694285180982604));
#39404=CARTESIAN_POINT('Ctrl Pts',(-0.515835954585742,0.437441765349259,
-0.683909708731887));
#39405=CARTESIAN_POINT('Ctrl Pts',(-0.660674884189079,0.144757748346355,
-0.673534236481169));
#39406=CARTESIAN_POINT('Ctrl Pts',(-0.651489301705309,-0.181675665347773,
-0.66315876423045));
#39407=CARTESIAN_POINT('Ctrl Pts',(-0.490426073855602,-0.465754385608829,
-0.652783291979732));
#39408=CARTESIAN_POINT('Ctrl Pts',(-0.215030571904435,-0.64125401525488,
-0.642407819729013));
#39409=CARTESIAN_POINT('Ctrl Pts',(0.110493809426251,-0.66725996774767,
-0.632032347478296));
#39410=CARTESIAN_POINT('Ctrl Pts',(0.410259379502582,-0.537710046135872,
-0.621656875227576));
#39411=CARTESIAN_POINT('Ctrl Pts',(0.614382465688009,-0.282805538385134,
-0.611281402976859));
#39412=CARTESIAN_POINT('Ctrl Pts',(0.675276726724032,0.0380284169940838,
-0.60090593072614));
#39413=CARTESIAN_POINT('Ctrl Pts',(0.57874600311102,0.349996958048548,-0.590530458475422));
#39414=CARTESIAN_POINT('Ctrl Pts',(0.347294217037289,0.580371894336871,
-0.580154986224702));
#39415=CARTESIAN_POINT('Ctrl Pts',(0.0348789097983566,0.675446719982932,
-0.569779513973986));
#39416=CARTESIAN_POINT('Ctrl Pts',(-0.285667594680009,0.613056958065561,
-0.559404041723266));
#39417=CARTESIAN_POINT('Ctrl Pts',(-0.539617391208136,0.407747324444045,
-0.549028569472549));
#39418=CARTESIAN_POINT('Ctrl Pts',(-0.667768028943849,0.10738095021671,
-0.538653097221829));
#39419=CARTESIAN_POINT('Ctrl Pts',(-0.640244189205681,-0.218018777541106,
-0.528277624971112));
#39420=CARTESIAN_POINT('Ctrl Pts',(-0.463462409944431,-0.492592533112403,
-0.517902152720393));
#39421=CARTESIAN_POINT('Ctrl Pts',(-0.178635223429194,-0.652329875185191,
-0.507526680469676));
#39422=CARTESIAN_POINT('Ctrl Pts',(0.14783658215608,-0.659991783359264,
-0.497151208218956));
#39423=CARTESIAN_POINT('Ctrl Pts',(0.439843750662663,-0.513792063108988,
-0.486775735968239));
#39424=CARTESIAN_POINT('Ctrl Pts',(0.629311649111721,-0.247813755493517,
-0.476400263717519));
#39425=CARTESIAN_POINT('Ctrl Pts',(0.672070273973121,0.0759365258431999,
-0.466024791466803));
#39426=CARTESIAN_POINT('Ctrl Pts',(0.55815145320655,0.381983984481368,-0.455649319216083));
#39427=CARTESIAN_POINT('Ctrl Pts',(0.314112692082441,0.59898082255559,-0.445273846965366));
#39428=CARTESIAN_POINT('Ctrl Pts',(-0.00315408721366853,0.676339308964272,
-0.434898374714647));
#39429=CARTESIAN_POINT('Ctrl Pts',(-0.319685564939782,0.59602512420693,
-0.424522902463929));
#39430=CARTESIAN_POINT('Ctrl Pts',(-0.561689839693175,0.376761639636888,
-0.41414743021321));
#39431=CARTESIAN_POINT('Ctrl Pts',(-0.672749282144793,0.0696650019042273,
-0.403771957962492));
#39432=CARTESIAN_POINT('Ctrl Pts',(-0.626972984110423,-0.25367239958757,
-0.393396485711774));
#39433=CARTESIAN_POINT('Ctrl Pts',(-0.435032617473759,-0.51787202169008,
-0.383021013461055));
#39434=CARTESIAN_POINT('Ctrl Pts',(-0.141674583798387,-0.661341909623961,
-0.372645541210337));
#39435=CARTESIAN_POINT('Ctrl Pts',(0.184711561311131,-0.650635418824393,
-0.362270068959619));
#39436=CARTESIAN_POINT('Ctrl Pts',(0.468036531532543,-0.488248516921783,
-0.3518945967089));
#39437=CARTESIAN_POINT('Ctrl Pts',(0.642249745047455,-0.212037907212844,
-0.341519124458182));
#39438=CARTESIAN_POINT('Ctrl Pts',(0.666737470904793,0.113604374920479,
-0.331143652207463));
#39439=CARTESIAN_POINT('Ctrl Pts',(0.535790969277522,0.412762457610684,
-0.320768179956746));
#39440=CARTESIAN_POINT('Ctrl Pts',(0.279937350483935,0.615694639210893,
-0.310392707706027));
#39441=CARTESIAN_POINT('Ctrl Pts',(-0.0411771059289157,0.675092034787015,
-0.300017235455309));
#39442=CARTESIAN_POINT('Ctrl Pts',(-0.352692084369553,0.577107530799868,
-0.28964176320459));
#39443=CARTESIAN_POINT('Ctrl Pts',(-0.581985162834664,0.344583923195399,
-0.279266290953873));
#39444=CARTESIAN_POINT('Ctrl Pts',(-0.675602029599326,0.0317286388769256,
-0.268890818703154));
#39445=CARTESIAN_POINT('Ctrl Pts',(-0.611718104794686,-0.288523425438239,
-0.258515346452436));
#39446=CARTESIAN_POINT('Ctrl Pts',(-0.405226428900723,-0.541513027982306,
-0.248139874201717));
#39447=CARTESIAN_POINT('Ctrl Pts',(-0.104265701531316,-0.668261513309247,
-0.237764401950999));
#39448=CARTESIAN_POINT('Ctrl Pts',(0.221002133831056,-0.639220548032841,
-0.22738892970028));
#39449=CARTESIAN_POINT('Ctrl Pts',(0.49474849438948,-0.46116013897505,-0.217013457449562));
#39450=CARTESIAN_POINT('Ctrl Pts',(0.653155835208594,-0.175591326286409,
-0.206637985198844));
#39451=CARTESIAN_POINT('Ctrl Pts',(0.659295177802631,0.150913054960382,
-0.196262512948126));
#39452=CARTESIAN_POINT('Ctrl Pts',(0.511735311224025,0.44223447272061,-0.185887040697407));
#39453=CARTESIAN_POINT('Ctrl Pts',(0.24487629716172,0.630461503497974,-0.175511568446689));
#39454=CARTESIAN_POINT('Ctrl Pts',(-0.0790698042728978,0.671706778414142,
-0.165136096195971));
#39455=CARTESIAN_POINT('Ctrl Pts',(-0.384582804555352,0.556368136401998,
-0.154760623945252));
#39456=CARTESIAN_POINT('Ctrl Pts',(-0.600438992610296,0.31130780842898,
-0.144385151694534));
#39457=CARTESIAN_POINT('Ctrl Pts',(-0.676317506997876,-0.00629169319767802,
-0.134009679443816));
#39458=CARTESIAN_POINT('Ctrl Pts',(-0.594527836101359,-0.322496282336175,
-0.123634207193097));
#39459=CARTESIAN_POINT('Ctrl Pts',(-0.447594141936034,-0.483058088236891,
-0.116717225692618));
#39460=CARTESIAN_POINT('Ctrl Pts',(-0.359573082794713,-0.541506181145704,
-0.113258734942379));
#39461=CARTESIAN_POINT('Ctrl Pts',(0.64510433218061,1.6868070912627E-15,
-0.740767637572532));
#39462=CARTESIAN_POINT('Ctrl Pts',(0.64510433218061,0.104863177208467,-0.737309146822293));
#39463=CARTESIAN_POINT('Ctrl Pts',(0.593022864567773,0.31448726492509,-0.730392165321814));
#39464=CARTESIAN_POINT('Ctrl Pts',(0.376496494207187,0.555705251652495,
-0.720016693071096));
#39465=CARTESIAN_POINT('Ctrl Pts',(0.0722580868424411,0.667330659810722,
-0.709641220820377));
#39466=CARTESIAN_POINT('Ctrl Pts',(-0.248854270731179,0.623404689437203,
-0.699265748569659));
#39467=CARTESIAN_POINT('Ctrl Pts',(-0.511937757444461,0.434135917498669,
-0.688890276318941));
#39468=CARTESIAN_POINT('Ctrl Pts',(-0.655682143940912,0.143663851624133,
-0.678514804068223));
#39469=CARTESIAN_POINT('Ctrl Pts',(-0.646565972288657,-0.180302757390696,
-0.668139331817503));
#39470=CARTESIAN_POINT('Ctrl Pts',(-0.486719907450942,-0.462234652383724,
-0.657763859566787));
#39471=CARTESIAN_POINT('Ctrl Pts',(-0.213405577826331,-0.636408041354094,
-0.647388387316067));
#39472=CARTESIAN_POINT('Ctrl Pts',(0.109658803578356,-0.662217457765674,
-0.637012915065349));
#39473=CARTESIAN_POINT('Ctrl Pts',(0.407159034924769,-0.533646553620086,
-0.626637442814631));
#39474=CARTESIAN_POINT('Ctrl Pts',(0.609739555547925,-0.28066836620718,
-0.616261970563912));
#39475=CARTESIAN_POINT('Ctrl Pts',(0.670173636573352,0.0377410345494586,
-0.605886498313194));
#39476=CARTESIAN_POINT('Ctrl Pts',(0.574372399022548,0.347352018796665,
-0.595511026062475));
#39477=CARTESIAN_POINT('Ctrl Pts',(0.344669702326589,0.57598600325603,-0.585135553811758));
#39478=CARTESIAN_POINT('Ctrl Pts',(0.0346153286363597,0.670342345204718,
-0.574760081561039));
#39479=CARTESIAN_POINT('Ctrl Pts',(-0.283508794531998,0.608424064864576,
-0.564384609310321));
#39480=CARTESIAN_POINT('Ctrl Pts',(-0.535539483442152,0.404665963460704,
-0.554009137059603));
#39481=CARTESIAN_POINT('Ctrl Pts',(-0.662721682261395,0.106569468561219,
-0.543633664808884));
#39482=CARTESIAN_POINT('Ctrl Pts',(-0.635405841157117,-0.21637120190275,
-0.533258192558166));
#39483=CARTESIAN_POINT('Ctrl Pts',(-0.459960008072277,-0.488869993867697,
-0.522882720307447));
#39484=CARTESIAN_POINT('Ctrl Pts',(-0.177285270709187,-0.647400195178034,
-0.512507248056729));
#39485=CARTESIAN_POINT('Ctrl Pts',(0.146719375860646,-0.655004202041331,
-0.502131775806011));
#39486=CARTESIAN_POINT('Ctrl Pts',(0.436519835836607,-0.509909318262488,
-0.491756303555293));
#39487=CARTESIAN_POINT('Ctrl Pts',(0.624555918656237,-0.245941018152811,
-0.481380831304573));
#39488=CARTESIAN_POINT('Ctrl Pts',(0.666991415072802,0.0753626708238029,
-0.471005359053856));
#39489=CARTESIAN_POINT('Ctrl Pts',(0.553933482875735,0.379097317960756,
-0.460629886803137));
#39490=CARTESIAN_POINT('Ctrl Pts',(0.311738931326063,0.594454303232302,
-0.450254414552419));
#39491=CARTESIAN_POINT('Ctrl Pts',(-0.00313025166471084,0.671228188815089,
-0.439878942301701));
#39492=CARTESIAN_POINT('Ctrl Pts',(-0.317269689785541,0.591520941200901,
-0.429503470050982));
#39493=CARTESIAN_POINT('Ctrl Pts',(-0.55744512965016,0.373914438561531,
-0.419127997800264));
#39494=CARTESIAN_POINT('Ctrl Pts',(-0.667665291955647,0.0691385410136651,
-0.408752525549546));
#39495=CARTESIAN_POINT('Ctrl Pts',(-0.622234927029288,-0.25175538826555,
-0.398377053298828));
#39496=CARTESIAN_POINT('Ctrl Pts',(-0.431745060551924,-0.513958444452011,
-0.388001581048109));
#39497=CARTESIAN_POINT('Ctrl Pts',(-0.140603943943023,-0.656344125353648,
-0.377626108797391));
#39498=CARTESIAN_POINT('Ctrl Pts',(0.183315689490009,-0.645718543884668,
-0.367250636546673));
#39499=CARTESIAN_POINT('Ctrl Pts',(0.464499562861689,-0.484558805560314,
-0.356875164295954));
#39500=CARTESIAN_POINT('Ctrl Pts',(0.637396240941466,-0.210435529226114,
-0.346499692045237));
#39501=CARTESIAN_POINT('Ctrl Pts',(0.661698912187562,0.112745862628511,
-0.336124219794517));
#39502=CARTESIAN_POINT('Ctrl Pts',(0.531741977914689,0.409643197078627,
-0.3257487475438));
#39503=CARTESIAN_POINT('Ctrl Pts',(0.277821854000763,0.611041812978763,
-0.315373275293081));
#39504=CARTESIAN_POINT('Ctrl Pts',(-0.0408659290876403,0.669990340339972,
-0.304997803042363));
#39505=CARTESIAN_POINT('Ctrl Pts',(-0.350026777759515,0.572746308704483,
-0.294622330791644));
#39506=CARTESIAN_POINT('Ctrl Pts',(-0.577587080349824,0.341979890292003,
-0.284246858540926));
#39507=CARTESIAN_POINT('Ctrl Pts',(-0.670496481026748,0.0314888643730044,
-0.273871386290208));
#39508=CARTESIAN_POINT('Ctrl Pts',(-0.607095329516257,-0.286343043569393,
-0.263495914039489));
#39509=CARTESIAN_POINT('Ctrl Pts',(-0.40216411812775,-0.537420795036202,
-0.253120441788771));
#39510=CARTESIAN_POINT('Ctrl Pts',(-0.103477762473797,-0.663211436920841,
-0.242744969538053));
#39511=CARTESIAN_POINT('Ctrl Pts',(0.219332013954502,-0.634389936526523,
-0.232369497287335));
#39512=CARTESIAN_POINT('Ctrl Pts',(0.491009660304339,-0.457675133757216,
-0.221994025036616));
#39513=CARTESIAN_POINT('Ctrl Pts',(0.648219917692676,-0.174264379762606,
-0.211618552785898));
#39514=CARTESIAN_POINT('Ctrl Pts',(0.654312852210673,0.149772606324681,
-0.20124308053518));
#39515=CARTESIAN_POINT('Ctrl Pts',(0.507868126312722,0.43889247785747,-0.190867608284461));
#39516=CARTESIAN_POINT('Ctrl Pts',(0.243025724530227,0.625697109920598,
-0.180492136033743));
#39517=CARTESIAN_POINT('Ctrl Pts',(-0.078472203834126,0.666630614047307,
-0.170116663783025));
#39518=CARTESIAN_POINT('Ctrl Pts',(-0.381676632120979,0.552163746877889,
-0.159741191532307));
#39519=CARTESIAN_POINT('Ctrl Pts',(-0.595901188052075,0.308955036721638,
-0.149365719281588));
#39520=CARTESIAN_POINT('Ctrl Pts',(-0.671207086309358,-0.00624372905956324,
-0.13899024703087));
#39521=CARTESIAN_POINT('Ctrl Pts',(-0.590033827093839,-0.32006005777858,
-0.128614774780151));
#39522=CARTESIAN_POINT('Ctrl Pts',(-0.444213509965361,-0.47940613564774,
-0.121697793279673));
#39523=CARTESIAN_POINT('Ctrl Pts',(-0.356855667887442,-0.537413836530842,
-0.118239302529433));
#39524=CARTESIAN_POINT('Ctrl Pts',(0.641722063808648,1.67796319735318E-15,
-0.742528335043099));
#39525=CARTESIAN_POINT('Ctrl Pts',(0.641722063808647,0.104311776723727,
-0.73906984429286));
#39526=CARTESIAN_POINT('Ctrl Pts',(0.589913462223807,0.312839321707124,
-0.73215286279238));
#39527=CARTESIAN_POINT('Ctrl Pts',(0.374522489184928,0.552791132218716,
-0.721777390541664));
#39528=CARTESIAN_POINT('Ctrl Pts',(0.0718792070526885,0.663831949137389,
-0.711401918290943));
#39529=CARTESIAN_POINT('Ctrl Pts',(-0.247549473477458,0.62013595091581,
-0.701026446040226));
#39530=CARTESIAN_POINT('Ctrl Pts',(-0.509253578428028,0.431859720500806,
-0.690650973789508));
#39531=CARTESIAN_POINT('Ctrl Pts',(-0.652244280175453,0.142910567006098,
-0.680275501538789));
#39532=CARTESIAN_POINT('Ctrl Pts',(-0.643175909604444,-0.179357382558957,
-0.669900029288072));
#39533=CARTESIAN_POINT('Ctrl Pts',(-0.484167945284686,-0.459811078726279,
-0.659524557037352));
#39534=CARTESIAN_POINT('Ctrl Pts',(-0.212286653582936,-0.633071233790531,
-0.649149084786634));
#39535=CARTESIAN_POINT('Ctrl Pts',(0.109083842531312,-0.658745332205166,
-0.638773612535916));
#39536=CARTESIAN_POINT('Ctrl Pts',(0.405024225471376,-0.530848546088013,
-0.628398140285198));
#39537=CARTESIAN_POINT('Ctrl Pts',(0.606542579433963,-0.279196771030968,
-0.618022668034478));
#39538=CARTESIAN_POINT('Ctrl Pts',(0.66665979345154,0.0375431516282889,
-0.607647195783762));
#39539=CARTESIAN_POINT('Ctrl Pts',(0.571360859360168,0.345530788434487,
-0.597271723533042));
#39540=CARTESIAN_POINT('Ctrl Pts',(0.342862535954226,0.572966003221409,
-0.586896251282324));
#39541=CARTESIAN_POINT('Ctrl Pts',(0.0344338341315972,0.666827617500848,
-0.576520779031606));
#39542=CARTESIAN_POINT('Ctrl Pts',(-0.282022306005166,0.60523398608833,
-0.566145306780888));
#39543=CARTESIAN_POINT('Ctrl Pts',(-0.532731551857879,0.40254422570126,
-0.555769834530169));
#39544=CARTESIAN_POINT('Ctrl Pts',(-0.659246911119028,0.106010705325554,
-0.545394362279451));
#39545=CARTESIAN_POINT('Ctrl Pts',(-0.632074291971503,-0.21523672806957,
-0.535018890028733));
#39546=CARTESIAN_POINT('Ctrl Pts',(-0.457548353518703,-0.486306758963348,
-0.524643417778014));
#39547=CARTESIAN_POINT('Ctrl Pts',(-0.176355731569013,-0.644005757398423,
-0.514267945527297));
#39548=CARTESIAN_POINT('Ctrl Pts',(0.145950099304638,-0.651569895060505,
-0.503892473276577));
#39549=CARTESIAN_POINT('Ctrl Pts',(0.43423108239854,-0.507235770328543,
-0.493517001025861));
#39550=CARTESIAN_POINT('Ctrl Pts',(0.621281257601356,-0.244651504356012,
-0.48314152877514));
#39551=CARTESIAN_POINT('Ctrl Pts',(0.663494256939109,0.0749675305396655,
-0.472766056524424));
#39552=CARTESIAN_POINT('Ctrl Pts',(0.551029108184565,0.377109641299561,
-0.462390584273704));
#39553=CARTESIAN_POINT('Ctrl Pts',(0.310104427021151,0.591337470459519,
-0.452015112022986));
#39554=CARTESIAN_POINT('Ctrl Pts',(-0.00311383918199809,0.667708816500798,
-0.441639639772268));
#39555=CARTESIAN_POINT('Ctrl Pts',(-0.31560618670119,0.588419488582432,
-0.431264167521549));
#39556=CARTESIAN_POINT('Ctrl Pts',(-0.554522342751875,0.371953936686142,
-0.420888695270832));
#39557=CARTESIAN_POINT('Ctrl Pts',(-0.664164600562044,0.0687760349819571,
-0.410513223020113));
#39558=CARTESIAN_POINT('Ctrl Pts',(-0.61897243535856,-0.25043538866153,
-0.400137750769395));
#39559=CARTESIAN_POINT('Ctrl Pts',(-0.429481342135034,-0.511263666207844,
-0.389762278518676));
#39560=CARTESIAN_POINT('Ctrl Pts',(-0.139866731716529,-0.652902792909725,
-0.379386806267958));
#39561=CARTESIAN_POINT('Ctrl Pts',(0.182354531759966,-0.642332923310336,
-0.369011334017239));
#39562=CARTESIAN_POINT('Ctrl Pts',(0.462064106590771,-0.48201817500657,
-0.358635861766521));
#39563=CARTESIAN_POINT('Ctrl Pts',(0.634054255725814,-0.209332177210148,
-0.348260389515803));
#39564=CARTESIAN_POINT('Ctrl Pts',(0.658229503614937,0.112154715424475,
-0.337884917265084));
#39565=CARTESIAN_POINT('Ctrl Pts',(0.528953957349416,0.407495362778231,
-0.327509445014367));
#39566=CARTESIAN_POINT('Ctrl Pts',(0.276365183140412,0.607838008857103,
-0.317133972763648));
#39567=CARTESIAN_POINT('Ctrl Pts',(-0.040651661531787,0.666477458287253,
-0.30675850051293));
#39568=CARTESIAN_POINT('Ctrl Pts',(-0.348191523276064,0.569743294931616,
-0.296383028262211));
#39569=CARTESIAN_POINT('Ctrl Pts',(-0.574558685491881,0.340186827082857,
-0.286007556011493));
#39570=CARTESIAN_POINT('Ctrl Pts',(-0.666980945237279,0.0313237625272405,
-0.275632083760775));
#39571=CARTESIAN_POINT('Ctrl Pts',(-0.60391221743454,-0.284841694627466,
-0.265256611510056));
#39572=CARTESIAN_POINT('Ctrl Pts',(-0.400055498194385,-0.534602999246615,
-0.254881139259338));
#39573=CARTESIAN_POINT('Ctrl Pts',(-0.102935209247226,-0.659734098192411,
-0.24450566700862));
#39574=CARTESIAN_POINT('Ctrl Pts',(0.218182015307551,-0.631063713343416,
-0.234130194757901));
#39575=CARTESIAN_POINT('Ctrl Pts',(0.488435208193123,-0.455275460354312,
-0.223754722507183));
#39576=CARTESIAN_POINT('Ctrl Pts',(0.644821179064956,-0.173350677448309,
-0.213379250256465));
#39577=CARTESIAN_POINT('Ctrl Pts',(0.65088217585303,0.148987316632804,-0.203003778005747));
#39578=CARTESIAN_POINT('Ctrl Pts',(0.505205269294179,0.436591293146462,
-0.192628305755028));
#39579=CARTESIAN_POINT('Ctrl Pts',(0.241751518866823,0.622416447653164,
-0.18225283350431));
#39580=CARTESIAN_POINT('Ctrl Pts',(-0.0780608048519096,0.663135382918645,
-0.171877361253591));
#39581=CARTESIAN_POINT('Ctrl Pts',(-0.379675341865185,0.549268581130195,
-0.161501889002874));
#39582=CARTESIAN_POINT('Ctrl Pts',(-0.592776947792401,0.307335268506549,
-0.151126416752155));
#39583=CARTESIAN_POINT('Ctrl Pts',(-0.667687464951409,-0.00621127295214926,
-0.140750944501437));
#39584=CARTESIAN_POINT('Ctrl Pts',(-0.586940939264991,-0.318381324725216,
-0.130375472250718));
#39585=CARTESIAN_POINT('Ctrl Pts',(-0.441883170803417,-0.476893507297812,
-0.12345849075024));
#39586=CARTESIAN_POINT('Ctrl Pts',(-0.354984681166936,-0.5345961871503,
-0.12));
#39587=CARTESIAN_POINT('',(-0.635960060745576,-0.14190617018468,-0.12));
#39588=CARTESIAN_POINT('',(-0.354984681166936,-0.5345961871503,-0.12));
#39589=CARTESIAN_POINT('Ctrl Pts',(-0.635960060745577,-0.141906170184675,
-0.12));
#39590=CARTESIAN_POINT('Ctrl Pts',(-0.618732434913983,-0.219112693030753,
-0.12));
#39591=CARTESIAN_POINT('Ctrl Pts',(-0.587040279218795,-0.292493231368224,
-0.12));
#39592=CARTESIAN_POINT('Ctrl Pts',(-0.514176950918451,-0.399397075481082,
-0.12));
#39593=CARTESIAN_POINT('Ctrl Pts',(-0.480780442117076,-0.437485150144931,
-0.12));
#39594=CARTESIAN_POINT('Ctrl Pts',(-0.411075652466351,-0.499087766122273,
-0.12));
#39595=CARTESIAN_POINT('Ctrl Pts',(-0.380549980087873,-0.519871240387648,
-0.12));
#39596=CARTESIAN_POINT('Ctrl Pts',(-0.354984681166936,-0.5345961871503,
-0.12));
#39597=CARTESIAN_POINT('',(0.651577129589243,7.55905383458807E-9,-0.726249999720643));
#39598=CARTESIAN_POINT('Ctrl Pts',(0.6516,1.70379184550113E-15,-0.72625));
#39599=CARTESIAN_POINT('Ctrl Pts',(0.6516,0.10591743302354,-0.722791509249761));
#39600=CARTESIAN_POINT('Ctrl Pts',(0.625296958000537,0.211786122892756,
-0.719333018499521));
#39601=CARTESIAN_POINT('Ctrl Pts',(0.575694361073646,0.305328026911275,
-0.715874527749282));
#39602=CARTESIAN_POINT('Ctrl Pts',(0.526091764146756,0.398869930929794,
-0.712416036999042));
#39603=CARTESIAN_POINT('Ctrl Pts',(0.453189612292437,0.480085049097615,
-0.708957546248803));
#39604=CARTESIAN_POINT('Ctrl Pts',(0.365521565197895,0.539484283577253,
-0.705499055498563));
#39605=CARTESIAN_POINT('Ctrl Pts',(0.277853518103352,0.59888351805689,-0.702040564748324));
#39606=CARTESIAN_POINT('Ctrl Pts',(0.175419575768586,0.636466868848343,
-0.698582073998084));
#39607=CARTESIAN_POINT('Ctrl Pts',(0.0701450044936301,0.647863776829187,
-0.695123583247845));
#39608=CARTESIAN_POINT('Ctrl Pts',(-0.0351295667813255,0.659260684810031,
-0.691665092497606));
#39609=CARTESIAN_POINT('Ctrl Pts',(-0.14324476699647,0.644471149980266,
-0.688206601747366));
#39610=CARTESIAN_POINT('Ctrl Pts',(-0.241591113588699,0.605213992636453,
-0.684748110997127));
#39611=CARTESIAN_POINT('Ctrl Pts',(-0.339937460180928,0.565956835292639,
-0.681289620246888));
#39612=CARTESIAN_POINT('Ctrl Pts',(-0.428514953150241,0.502232055434778,
-0.677831129496648));
#39613=CARTESIAN_POINT('Ctrl Pts',(-0.497002322505376,0.421470181072845,
-0.674372638746409));
#39614=CARTESIAN_POINT('Ctrl Pts',(-0.565489691860511,0.340708306710911,
-0.670914147996169));
#39615=CARTESIAN_POINT('Ctrl Pts',(-0.613886937601468,0.242909337844905,
-0.667455657245929));
#39616=CARTESIAN_POINT('Ctrl Pts',(-0.636550900687667,0.139471757721302,
-0.66399716649569));
#39617=CARTESIAN_POINT('Ctrl Pts',(-0.659214863773866,0.0360341775977008,
-0.660538675745451));
#39618=CARTESIAN_POINT('Ctrl Pts',(-0.656145544205308,-0.0730420137834978,
-0.657080184995211));
#39619=CARTESIAN_POINT('Ctrl Pts',(-0.627701625882157,-0.175041889458731,
-0.653621694244972));
#39620=CARTESIAN_POINT('Ctrl Pts',(-0.599257707559006,-0.277041765133964,
-0.650163203494733));
#39621=CARTESIAN_POINT('Ctrl Pts',(-0.545439190481261,-0.371965325103232,
-0.646704712744493));
#39622=CARTESIAN_POINT('Ctrl Pts',(-0.472518878335208,-0.448748292407348,
-0.643246221994254));
#39623=CARTESIAN_POINT('Ctrl Pts',(-0.399598566189156,-0.525531259711463,
-0.639787731244014));
#39624=CARTESIAN_POINT('Ctrl Pts',(-0.307576458974796,-0.584173634350426,
-0.636329240493775));
#39625=CARTESIAN_POINT('Ctrl Pts',(-0.207179187647643,-0.617839704361461,
-0.632870749743535));
#39626=CARTESIAN_POINT('Ctrl Pts',(-0.10678191632049,-0.651505774372495,
-0.629412258993296));
#39627=CARTESIAN_POINT('Ctrl Pts',(0.00199051911945597,-0.6601955397556,
-0.625953768243056));
#39628=CARTESIAN_POINT('Ctrl Pts',(0.106459362012925,-0.64289617526343,
-0.622495277492817));
#39629=CARTESIAN_POINT('Ctrl Pts',(0.210928204906394,-0.62559681077126,
-0.619036786742578));
#39630=CARTESIAN_POINT('Ctrl Pts',(0.311093455253387,-0.582308316403815,
-0.615578295992338));
#39631=CARTESIAN_POINT('Ctrl Pts',(0.395279463300225,-0.518076500064383,
-0.612119805242099));
#39632=CARTESIAN_POINT('Ctrl Pts',(0.479465471347062,-0.453844683724952,
-0.608661314491859));
#39633=CARTESIAN_POINT('Ctrl Pts',(0.547672237093744,-0.368669545413534,
-0.60520282374162));
#39634=CARTESIAN_POINT('Ctrl Pts',(0.591949384920031,-0.272479400406464,
-0.60174433299138));
#39635=CARTESIAN_POINT('Ctrl Pts',(0.636226532746319,-0.176289255399394,
-0.598285842241141));
#39636=CARTESIAN_POINT('Ctrl Pts',(0.656574062652212,-0.0690841036966703,
-0.594827351490901));
#39637=CARTESIAN_POINT('Ctrl Pts',(0.650620184773465,0.0366398799159285,
-0.591368860740662));
#39638=CARTESIAN_POINT('Ctrl Pts',(0.644666306894718,0.142363863528527,
-0.587910369990422));
#39639=CARTESIAN_POINT('Ctrl Pts',(0.612411021231331,0.246606679051001,
-0.584451879240183));
#39640=CARTESIAN_POINT('Ctrl Pts',(0.557614117482213,0.337217435579939,
-0.580993388489944));
#39641=CARTESIAN_POINT('Ctrl Pts',(0.502817213733094,0.427828192108876,
-0.577534897739704));
#39642=CARTESIAN_POINT('Ctrl Pts',(0.425478691898243,0.504806889644278,
-0.574076406989465));
#39643=CARTESIAN_POINT('Ctrl Pts',(0.334613380841695,0.559180640531877,
-0.570617916239225));
#39644=CARTESIAN_POINT('Ctrl Pts',(0.243748069785148,0.613554391419475,
-0.567159425488986));
#39645=CARTESIAN_POINT('Ctrl Pts',(0.139355969506901,0.64532319565927,-0.563700934738746));
#39646=CARTESIAN_POINT('Ctrl Pts',(0.0336053686408143,0.650783975546671,
-0.560242443988507));
#39647=CARTESIAN_POINT('Ctrl Pts',(-0.0721452322252732,0.656244755434072,
-0.556783953238268));
#39648=CARTESIAN_POINT('Ctrl Pts',(-0.179254333679203,0.635397510969078,
-0.553325462488028));
#39649=CARTESIAN_POINT('Ctrl Pts',(-0.275236947324888,0.590672266243827,
-0.549866971737789));
#39650=CARTESIAN_POINT('Ctrl Pts',(-0.371219560970573,0.545947021518575,
-0.546408480987549));
#39651=CARTESIAN_POINT('Ctrl Pts',(-0.456075686808014,0.477343776533065,
-0.54294999023731));
#39652=CARTESIAN_POINT('Ctrl Pts',(-0.519914215083365,0.39285915094755,
-0.53949149948707));
#39653=CARTESIAN_POINT('Ctrl Pts',(-0.583752743358716,0.308374525362036,
-0.536033008736831));
#39654=CARTESIAN_POINT('Ctrl Pts',(-0.626573674071979,0.208008519176516,
-0.532574517986592));
#39655=CARTESIAN_POINT('Ctrl Pts',(-0.643385658862261,0.103460124531451,
-0.529116027236352));
#39656=CARTESIAN_POINT('Ctrl Pts',(-0.660197643652543,-0.00108827011361441,
-0.525657536486113));
#39657=CARTESIAN_POINT('Ctrl Pts',(-0.651000682519846,-0.109819053218224,
-0.522199045735874));
#39658=CARTESIAN_POINT('Ctrl Pts',(-0.616866803398733,-0.210058206972732,
-0.518740554985634));
#39659=CARTESIAN_POINT('Ctrl Pts',(-0.58273292427762,-0.310297360727239,
-0.515282064235395));
#39660=CARTESIAN_POINT('Ctrl Pts',(-0.523662127168093,-0.402044885131643,
-0.511823573485155));
#39661=CARTESIAN_POINT('Ctrl Pts',(-0.446539898635107,-0.474606386771079,
-0.508365082734915));
#39662=CARTESIAN_POINT('Ctrl Pts',(-0.36941767010212,-0.547167888410515,
-0.504906591984676));
#39663=CARTESIAN_POINT('Ctrl Pts',(-0.274244010145674,-0.600543367284983,
-0.501448101234437));
#39664=CARTESIAN_POINT('Ctrl Pts',(-0.172112673741822,-0.628511201947908,
-0.497989610484197));
#39665=CARTESIAN_POINT('Ctrl Pts',(-0.0699813373379707,-0.656479036610833,
-0.494531119733958));
#39666=CARTESIAN_POINT('Ctrl Pts',(0.039107675513287,-0.659039227062215,
-0.491072628983718));
#39667=CARTESIAN_POINT('Ctrl Pts',(0.142438590463173,-0.635893349066943,
-0.487614138233479));
#39668=CARTESIAN_POINT('Ctrl Pts',(0.245769505413058,-0.612747471071672,
-0.484155647483239));
#39669=CARTESIAN_POINT('Ctrl Pts',(0.343342322461571,-0.563895524629746,
-0.480697156733));
#39670=CARTESIAN_POINT('Ctrl Pts',(0.423783632963894,-0.495031853388289,
-0.477238665982761));
#39671=CARTESIAN_POINT('Ctrl Pts',(0.504224943466218,-0.426168182146832,
-0.473780175232521));
#39672=CARTESIAN_POINT('Ctrl Pts',(0.567534747422353,-0.337292786105845,
-0.470321684482282));
#39673=CARTESIAN_POINT('Ctrl Pts',(0.606333445736285,-0.238765273900591,
-0.466863193732042));
#39674=CARTESIAN_POINT('Ctrl Pts',(0.645132144050218,-0.140237761695336,
-0.463404702981803));
#39675=CARTESIAN_POINT('Ctrl Pts',(0.659419736721948,-0.0320581333258157,
-0.459946212231564));
#39676=CARTESIAN_POINT('Ctrl Pts',(0.647530814933311,0.0731638377210296,
-0.456487721481324));
#39677=CARTESIAN_POINT('Ctrl Pts',(0.635641893144675,0.178385808767874,
-0.453029230731085));
#39678=CARTESIAN_POINT('Ctrl Pts',(0.597576456895672,0.280650122492043,
-0.449570739980845));
#39679=CARTESIAN_POINT('Ctrl Pts',(0.537771538702094,0.368036513950164,
-0.446112249230605));
#39680=CARTESIAN_POINT('Ctrl Pts',(0.477966620508516,0.455422905408286,
-0.442653758480366));
#39681=CARTESIAN_POINT('Ctrl Pts',(0.396422220370362,0.527931374600361,
-0.439195267730127));
#39682=CARTESIAN_POINT('Ctrl Pts',(0.302643421918522,0.57711009574258,-0.435736776979887));
#39683=CARTESIAN_POINT('Ctrl Pts',(0.208864623466684,0.626288816884798,
-0.432278286229648));
#39684=CARTESIAN_POINT('Ctrl Pts',(0.102851426701161,0.652137789977161,
-0.428819795479408));
#39685=CARTESIAN_POINT('Ctrl Pts',(-0.00303892128990968,0.651643973651179,
-0.425361304729169));
#39686=CARTESIAN_POINT('Ctrl Pts',(-0.108929269280981,0.651150157325197,
-0.421902813978929));
#39687=CARTESIAN_POINT('Ctrl Pts',(-0.2146967684976,0.624313551580869,-0.41844432322869));
#39688=CARTESIAN_POINT('Ctrl Pts',(-0.308012811166104,0.574262319498799,
-0.414985832478451));
#39689=CARTESIAN_POINT('Ctrl Pts',(-0.401328853834608,0.524211087416729,
-0.411527341728211));
#39690=CARTESIAN_POINT('Ctrl Pts',(-0.482193439954999,0.450945228996916,
-0.408068850977972));
#39691=CARTESIAN_POINT('Ctrl Pts',(-0.541180727256026,0.363004853803835,
-0.404610360227732));
#39692=CARTESIAN_POINT('Ctrl Pts',(-0.600168014557053,0.275064478610752,
-0.401151869477493));
#39693=CARTESIAN_POINT('Ctrl Pts',(-0.637278003038717,0.1724495866444,-0.397693378727254));
#39694=CARTESIAN_POINT('Ctrl Pts',(-0.648185030320193,0.0671213074021386,
-0.394234887977014));
#39695=CARTESIAN_POINT('Ctrl Pts',(-0.659092057601669,-0.0382069718401229,
-0.390776397226775));
#39696=CARTESIAN_POINT('Ctrl Pts',(-0.643796123682957,-0.146248638358292,
-0.387317906476535));
#39697=CARTESIAN_POINT('Ctrl Pts',(-0.604080172958263,-0.244409999953607,
-0.383859415726295));
#39698=CARTESIAN_POINT('Ctrl Pts',(-0.564364222233568,-0.342571361548922,
-0.380400924976056));
#39699=CARTESIAN_POINT('Ctrl Pts',(-0.50022825470289,-0.430852418221385,
-0.376942434225817));
#39700=CARTESIAN_POINT('Ctrl Pts',(-0.419148169803331,-0.498962839486855,
-0.373483943475577));
#39701=CARTESIAN_POINT('Ctrl Pts',(-0.338068084903774,-0.567073260752324,
-0.370025452725338));
#39702=CARTESIAN_POINT('Ctrl Pts',(-0.240043882635337,-0.615013046610803,
-0.366566961975098));
#39703=CARTESIAN_POINT('Ctrl Pts',(-0.13650158659733,-0.637194177857639,
-0.363108471224859));
#39704=CARTESIAN_POINT('Ctrl Pts',(-0.0329592905593207,-0.659375309104476,
-0.359649980474619));
#39705=CARTESIAN_POINT('Ctrl Pts',(0.0761010992482581,-0.65579778573967,
-0.35619148972438));
#39706=CARTESIAN_POINT('Ctrl Pts',(0.17796714488833,-0.626878615664482,
-0.352732998974141));
#39707=CARTESIAN_POINT('Ctrl Pts',(0.279833190528402,-0.597959445589294,
-0.349274508223901));
#39708=CARTESIAN_POINT('Ctrl Pts',(0.374504892000968,-0.543698628803726,
-0.345816017473662));
#39709=CARTESIAN_POINT('Ctrl Pts',(0.450947004231846,-0.470420984666961,
-0.342357526723422));
#39710=CARTESIAN_POINT('Ctrl Pts',(0.527389116462723,-0.397143340530196,
-0.338899035973183));
#39711=CARTESIAN_POINT('Ctrl Pts',(0.585601639451913,-0.304848869042235,
-0.335440545222943));
#39712=CARTESIAN_POINT('Ctrl Pts',(0.618799129951752,-0.204295717545714,
-0.331982054472704));
#39713=CARTESIAN_POINT('Ctrl Pts',(0.651996620451591,-0.103742566049191,
-0.328523563722465));
#39714=CARTESIAN_POINT('Ctrl Pts',(0.660179078462078,0.00506926545589149,
-0.325065072972225));
#39715=CARTESIAN_POINT('Ctrl Pts',(0.642392729749155,0.109456311843489,
-0.321606582221986));
#39716=CARTESIAN_POINT('Ctrl Pts',(0.624606381036232,0.213843358231086,
-0.318148091471746));
#39717=CARTESIAN_POINT('Ctrl Pts',(0.580851225599901,0.313805619501198,
-0.314689600721507));
#39718=CARTESIAN_POINT('Ctrl Pts',(0.516227508351651,0.397691165445017,
-0.311231109971267));
#39719=CARTESIAN_POINT('Ctrl Pts',(0.451603791103401,0.481576711388838,
-0.307772619221028));
#39720=CARTESIAN_POINT('Ctrl Pts',(0.366111512043233,0.549385542006366,
-0.304314128470789));
#39721=CARTESIAN_POINT('Ctrl Pts',(0.269715932556123,0.593213637000255,
-0.300855637720549));
#39722=CARTESIAN_POINT('Ctrl Pts',(0.173320353069013,0.637041731994143,
-0.29739714697031));
#39723=CARTESIAN_POINT('Ctrl Pts',(0.0660214731549615,0.656889091364393,
-0.29393865622007));
#39724=CARTESIAN_POINT('Ctrl Pts',(-0.0396735966300387,0.65044224129389,
-0.290480165469831));
#39725=CARTESIAN_POINT('Ctrl Pts',(-0.145368666415039,0.643995391223387,
-0.287021674719591));
#39726=CARTESIAN_POINT('Ctrl Pts',(-0.249459926070987,0.611254331712133,
-0.283563183969352));
#39727=CARTESIAN_POINT('Ctrl Pts',(-0.339814155841332,0.556035468987531,
-0.280104693219112));
#39728=CARTESIAN_POINT('Ctrl Pts',(-0.430168385611676,0.500816606262931,
-0.276646202468873));
#39729=CARTESIAN_POINT('Ctrl Pts',(-0.506785585496417,0.423119940324984,
-0.273187711718634));
#39730=CARTESIAN_POINT('Ctrl Pts',(-0.560735002506506,0.332002049080791,
-0.269729220968394));
#39731=CARTESIAN_POINT('Ctrl Pts',(-0.614684419516595,0.240884157836599,
-0.266270730218155));
#39732=CARTESIAN_POINT('Ctrl Pts',(-0.645966053652034,0.136345041286161,
-0.262812239467915));
#39733=CARTESIAN_POINT('Ctrl Pts',(-0.650933614764165,0.0305701251879336,
-0.259353748717676));
#39734=CARTESIAN_POINT('Ctrl Pts',(-0.655901175876297,-0.075204790910295,
-0.255895257967436));
#39735=CARTESIAN_POINT('Ctrl Pts',(-0.634554663965122,-0.182215506556313,
-0.252436767217197));
#39736=CARTESIAN_POINT('Ctrl Pts',(-0.589382298569403,-0.27798850517175,
-0.248978276466957));
#39737=CARTESIAN_POINT('Ctrl Pts',(-0.544209933173686,-0.373761503787186,
-0.245519785716718));
#39738=CARTESIAN_POINT('Ctrl Pts',(-0.475211714293426,-0.458296785372042,
-0.242061294966479));
#39739=CARTESIAN_POINT('Ctrl Pts',(-0.390430301657806,-0.521740630181612,
-0.238602804216239));
#39740=CARTESIAN_POINT('Ctrl Pts',(-0.305648889022187,-0.585184474991182,
-0.235144313466));
#39741=CARTESIAN_POINT('Ctrl Pts',(-0.205084282631209,-0.627536883025467,
-0.23168582271576));
#39742=CARTESIAN_POINT('Ctrl Pts',(-0.100458623404491,-0.643861136377049,
-0.228227331965521));
#39743=CARTESIAN_POINT('Ctrl Pts',(0.00416703582222801,-0.660185389728631,
-0.224768841215281));
#39744=CARTESIAN_POINT('Ctrl Pts',(0.112853747884687,-0.650481488397511,
-0.221310350465042));
#39745=CARTESIAN_POINT('Ctrl Pts',(0.212932630871593,-0.615880514983204,
-0.217851859714803));
#39746=CARTESIAN_POINT('Ctrl Pts',(0.3130115138585,-0.581279541568896,-0.214393368964563));
#39747=CARTESIAN_POINT('Ctrl Pts',(0.404482567769854,-0.521781496071402,
-0.210934878214324));
#39748=CARTESIAN_POINT('Ctrl Pts',(0.47668362769456,-0.444321738176853,
-0.207476387464084));
#39749=CARTESIAN_POINT('Ctrl Pts',(0.548884687619267,-0.366861980282302,
-0.204017896713845));
#39750=CARTESIAN_POINT('Ctrl Pts',(0.601815753557325,-0.271440509990697,
-0.200559405963605));
#39751=CARTESIAN_POINT('Ctrl Pts',(0.629307002000867,-0.169179825370744,
-0.197100915213366));
#39752=CARTESIAN_POINT('Ctrl Pts',(0.656798250444408,-0.0669191407507926,
-0.193642424463126));
#39753=CARTESIAN_POINT('Ctrl Pts',(0.658849681393434,0.0421807581975068,
-0.190183933712887));
#39754=CARTESIAN_POINT('Ctrl Pts',(0.635222181800982,0.145402544921586,
-0.186725442962648));
#39755=CARTESIAN_POINT('Ctrl Pts',(0.61159468220853,0.248624331645664,-0.183266952212408));
#39756=CARTESIAN_POINT('Ctrl Pts',(0.5622882520746,0.345968006145523,-0.179808461462169));
#39757=CARTESIAN_POINT('Ctrl Pts',(0.493050194269639,0.426087432496028,
-0.176349970711929));
#39758=CARTESIAN_POINT('Ctrl Pts',(0.423812136464678,0.506206858846533,
-0.17289147996169));
#39759=CARTESIAN_POINT('Ctrl Pts',(0.334642450988686,0.569102037047685,
-0.16943298921145));
#39760=CARTESIAN_POINT('Ctrl Pts',(0.235935083384207,0.607440578819556,
-0.165974498461211));
#39761=CARTESIAN_POINT('Ctrl Pts',(0.137227715779728,0.645779120591427,
-0.162516007710972));
#39762=CARTESIAN_POINT('Ctrl Pts',(0.0289826660467615,0.659561025934017,
-0.159057516960732));
#39763=CARTESIAN_POINT('Ctrl Pts',(-0.0761827332461323,0.64718205573429,
-0.155599026210493));
#39764=CARTESIAN_POINT('Ctrl Pts',(-0.181348132539026,0.634803085534563,
-0.152140535460253));
#39765=CARTESIAN_POINT('Ctrl Pts',(-0.283433881391847,0.59626323979252,
-0.148682044710014));
#39766=CARTESIAN_POINT('Ctrl Pts',(-0.370540397243242,0.536050423989017,
-0.145223553959774));
#39767=CARTESIAN_POINT('Ctrl Pts',(-0.457646913094635,0.475837608185515,
-0.141765063209535));
#39768=CARTESIAN_POINT('Ctrl Pts',(-0.529774195944603,0.393951822320553,
-0.138306572459295));
#39769=CARTESIAN_POINT('Ctrl Pts',(-0.578515104713621,0.299946776280357,
-0.134848081709056));
#39770=CARTESIAN_POINT('Ctrl Pts',(-0.627256013482641,0.205941730240159,
-0.131389590958817));
#39771=CARTESIAN_POINT('Ctrl Pts',(-0.652610548170711,0.0998174240247245,
-0.127931100208577));
#39772=CARTESIAN_POINT('Ctrl Pts',(-0.651622907941676,-0.00607393589154021,
-0.124472609458338));
#39773=CARTESIAN_POINT('Ctrl Pts',(-0.651197160667425,-0.0517210820139664,
-0.122981739638892));
#39774=CARTESIAN_POINT('Ctrl Pts',(-0.645876355431924,-0.097324940684241,
-0.121490869819446));
#39775=CARTESIAN_POINT('Ctrl Pts',(-0.635915580576687,-0.141895556916034,
-0.12));
#39776=CARTESIAN_POINT('',(0.462889160393651,0.44445565849575,-0.72625));
#39777=CARTESIAN_POINT('Ctrl Pts',(0.46288916039365,0.444455658495751,-0.72625));
#39778=CARTESIAN_POINT('Ctrl Pts',(0.484632932366815,0.424517500232759,
-0.72625));
#39779=CARTESIAN_POINT('Ctrl Pts',(0.509898268129295,0.397586621949268,
-0.72625));
#39780=CARTESIAN_POINT('Ctrl Pts',(0.564515398139937,0.322282107413605,
-0.72625));
#39781=CARTESIAN_POINT('Ctrl Pts',(0.588817231863487,0.277831998563094,
-0.72625));
#39782=CARTESIAN_POINT('Ctrl Pts',(0.636649969955028,0.157623573436602,
-0.72625));
#39783=CARTESIAN_POINT('Ctrl Pts',(0.6516,0.079103795955392,-0.72625));
#39784=CARTESIAN_POINT('Ctrl Pts',(0.6516,2.83106871279415E-15,-0.72625));
#39785=CARTESIAN_POINT('Ctrl Pts',(0.462856220566271,0.444424947352554,
-0.72625));
#39786=CARTESIAN_POINT('Ctrl Pts',(0.431715399494611,0.476878719990873,
-0.724759130180555));
#39787=CARTESIAN_POINT('Ctrl Pts',(0.317128739570665,0.573849087968775,
-0.71980976961087));
#39788=CARTESIAN_POINT('Ctrl Pts',(0.0718792070526885,0.663831949137389,
-0.711401918290943));
#39789=CARTESIAN_POINT('Ctrl Pts',(-0.247549473477458,0.62013595091581,
-0.701026446040226));
#39790=CARTESIAN_POINT('Ctrl Pts',(-0.509253578428028,0.431859720500806,
-0.690650973789508));
#39791=CARTESIAN_POINT('Ctrl Pts',(-0.652244280175453,0.142910567006098,
-0.680275501538789));
#39792=CARTESIAN_POINT('Ctrl Pts',(-0.643175909604444,-0.179357382558957,
-0.669900029288072));
#39793=CARTESIAN_POINT('Ctrl Pts',(-0.484167945284686,-0.459811078726279,
-0.659524557037352));
#39794=CARTESIAN_POINT('Ctrl Pts',(-0.212286653582936,-0.633071233790531,
-0.649149084786634));
#39795=CARTESIAN_POINT('Ctrl Pts',(0.109083842531312,-0.658745332205166,
-0.638773612535916));
#39796=CARTESIAN_POINT('Ctrl Pts',(0.405024225471376,-0.530848546088013,
-0.628398140285198));
#39797=CARTESIAN_POINT('Ctrl Pts',(0.606542579433963,-0.279196771030968,
-0.618022668034478));
#39798=CARTESIAN_POINT('Ctrl Pts',(0.66665979345154,0.0375431516282889,
-0.607647195783762));
#39799=CARTESIAN_POINT('Ctrl Pts',(0.571360859360168,0.345530788434487,
-0.597271723533042));
#39800=CARTESIAN_POINT('Ctrl Pts',(0.342862535954226,0.572966003221409,
-0.586896251282324));
#39801=CARTESIAN_POINT('Ctrl Pts',(0.0344338341315972,0.666827617500848,
-0.576520779031606));
#39802=CARTESIAN_POINT('Ctrl Pts',(-0.282022306005166,0.60523398608833,
-0.566145306780888));
#39803=CARTESIAN_POINT('Ctrl Pts',(-0.532731551857879,0.40254422570126,
-0.555769834530169));
#39804=CARTESIAN_POINT('Ctrl Pts',(-0.659246911119028,0.106010705325554,
-0.545394362279451));
#39805=CARTESIAN_POINT('Ctrl Pts',(-0.632074291971503,-0.21523672806957,
-0.535018890028733));
#39806=CARTESIAN_POINT('Ctrl Pts',(-0.457548353518703,-0.486306758963348,
-0.524643417778014));
#39807=CARTESIAN_POINT('Ctrl Pts',(-0.176355731569013,-0.644005757398423,
-0.514267945527297));
#39808=CARTESIAN_POINT('Ctrl Pts',(0.145950099304638,-0.651569895060505,
-0.503892473276577));
#39809=CARTESIAN_POINT('Ctrl Pts',(0.43423108239854,-0.507235770328543,
-0.493517001025861));
#39810=CARTESIAN_POINT('Ctrl Pts',(0.621281257601356,-0.244651504356012,
-0.48314152877514));
#39811=CARTESIAN_POINT('Ctrl Pts',(0.663494256939109,0.0749675305396655,
-0.472766056524424));
#39812=CARTESIAN_POINT('Ctrl Pts',(0.551029108184565,0.377109641299561,
-0.462390584273704));
#39813=CARTESIAN_POINT('Ctrl Pts',(0.310104427021151,0.591337470459519,
-0.452015112022986));
#39814=CARTESIAN_POINT('Ctrl Pts',(-0.00311383918199809,0.667708816500798,
-0.441639639772268));
#39815=CARTESIAN_POINT('Ctrl Pts',(-0.31560618670119,0.588419488582432,
-0.431264167521549));
#39816=CARTESIAN_POINT('Ctrl Pts',(-0.554522342751875,0.371953936686142,
-0.420888695270832));
#39817=CARTESIAN_POINT('Ctrl Pts',(-0.664164600562044,0.0687760349819571,
-0.410513223020113));
#39818=CARTESIAN_POINT('Ctrl Pts',(-0.61897243535856,-0.25043538866153,
-0.400137750769395));
#39819=CARTESIAN_POINT('Ctrl Pts',(-0.429481342135034,-0.511263666207844,
-0.389762278518676));
#39820=CARTESIAN_POINT('Ctrl Pts',(-0.139866731716529,-0.652902792909725,
-0.379386806267958));
#39821=CARTESIAN_POINT('Ctrl Pts',(0.182354531759966,-0.642332923310336,
-0.369011334017239));
#39822=CARTESIAN_POINT('Ctrl Pts',(0.462064106590771,-0.48201817500657,
-0.358635861766521));
#39823=CARTESIAN_POINT('Ctrl Pts',(0.634054255725814,-0.209332177210148,
-0.348260389515803));
#39824=CARTESIAN_POINT('Ctrl Pts',(0.658229503614937,0.112154715424475,
-0.337884917265084));
#39825=CARTESIAN_POINT('Ctrl Pts',(0.528953957349416,0.407495362778231,
-0.327509445014367));
#39826=CARTESIAN_POINT('Ctrl Pts',(0.276365183140412,0.607838008857103,
-0.317133972763648));
#39827=CARTESIAN_POINT('Ctrl Pts',(-0.040651661531787,0.666477458287253,
-0.30675850051293));
#39828=CARTESIAN_POINT('Ctrl Pts',(-0.348191523276064,0.569743294931616,
-0.296383028262211));
#39829=CARTESIAN_POINT('Ctrl Pts',(-0.574558685491881,0.340186827082857,
-0.286007556011493));
#39830=CARTESIAN_POINT('Ctrl Pts',(-0.666980945237279,0.0313237625272405,
-0.275632083760775));
#39831=CARTESIAN_POINT('Ctrl Pts',(-0.60391221743454,-0.284841694627466,
-0.265256611510056));
#39832=CARTESIAN_POINT('Ctrl Pts',(-0.400055498194385,-0.534602999246615,
-0.254881139259338));
#39833=CARTESIAN_POINT('Ctrl Pts',(-0.102935209247226,-0.659734098192411,
-0.24450566700862));
#39834=CARTESIAN_POINT('Ctrl Pts',(0.218182015307551,-0.631063713343416,
-0.234130194757901));
#39835=CARTESIAN_POINT('Ctrl Pts',(0.488435208193123,-0.455275460354312,
-0.223754722507183));
#39836=CARTESIAN_POINT('Ctrl Pts',(0.644821179064956,-0.173350677448309,
-0.213379250256465));
#39837=CARTESIAN_POINT('Ctrl Pts',(0.65088217585303,0.148987316632804,-0.203003778005747));
#39838=CARTESIAN_POINT('Ctrl Pts',(0.505205269294179,0.436591293146462,
-0.192628305755028));
#39839=CARTESIAN_POINT('Ctrl Pts',(0.241751518866823,0.622416447653164,
-0.18225283350431));
#39840=CARTESIAN_POINT('Ctrl Pts',(-0.0780608048519096,0.663135382918645,
-0.171877361253591));
#39841=CARTESIAN_POINT('Ctrl Pts',(-0.379675341865185,0.549268581130195,
-0.161501889002874));
#39842=CARTESIAN_POINT('Ctrl Pts',(-0.592776947792401,0.307335268506549,
-0.151126416752155));
#39843=CARTESIAN_POINT('Ctrl Pts',(-0.667687464951409,-0.00621127295214926,
-0.140750944501437));
#39844=CARTESIAN_POINT('Ctrl Pts',(-0.586940939264991,-0.318381324725216,
-0.130375472250718));
#39845=CARTESIAN_POINT('Ctrl Pts',(-0.441883170803417,-0.476893507297812,
-0.12345849075024));
#39846=CARTESIAN_POINT('Ctrl Pts',(-0.354984681166936,-0.5345961871503,
-0.12));
#39847=CARTESIAN_POINT('Ctrl Pts',(0.419902519832407,0.403180862557734,
-0.75727273924394));
#39848=CARTESIAN_POINT('Ctrl Pts',(0.352813337597515,0.473052523864309,
-0.753732335137029));
#39849=CARTESIAN_POINT('Ctrl Pts',(0.183146826434185,0.578585044749363,
-0.746651526923207));
#39850=CARTESIAN_POINT('Ctrl Pts',(-0.116229043222437,0.595630586916603,
-0.736030314602476));
#39851=CARTESIAN_POINT('Ctrl Pts',(-0.38716554463002,0.467313281319197,
-0.725409102281742));
#39852=CARTESIAN_POINT('Ctrl Pts',(-0.5636424333859,0.224934817531868,-0.714787889961011));
#39853=CARTESIAN_POINT('Ctrl Pts',(-0.602534986633661,-0.0723403849529277,
-0.704166677640278));
#39854=CARTESIAN_POINT('Ctrl Pts',(-0.494377117526733,-0.351960929022743,
-0.693545465319546));
#39855=CARTESIAN_POINT('Ctrl Pts',(-0.265553394359715,-0.545678585605523,
-0.682924252998813));
#39856=CARTESIAN_POINT('Ctrl Pts',(0.0280810564139534,-0.606214132210099,
-0.672303040678082));
#39857=CARTESIAN_POINT('Ctrl Pts',(0.314862960821169,-0.518792316784799,
-0.661681828357348));
#39858=CARTESIAN_POINT('Ctrl Pts',(0.524796465182481,-0.30475021433233,
-0.651060616036617));
#39859=CARTESIAN_POINT('Ctrl Pts',(0.60664446863493,-0.0163284320554081,
-0.640439403715884));
#39860=CARTESIAN_POINT('Ctrl Pts',(0.540430098503603,0.27607856963071,-0.629818191395151));
#39861=CARTESIAN_POINT('Ctrl Pts',(0.342314351095128,0.501103761813076,
-0.619196979074419));
#39862=CARTESIAN_POINT('Ctrl Pts',(0.0606507420151454,0.603825781241362,
-0.608575766753688));
#39863=CARTESIAN_POINT('Ctrl Pts',(-0.235815726583716,0.55917352432788,
-0.597954554432955));
#39864=CARTESIAN_POINT('Ctrl Pts',(-0.474727237871055,0.378045153975223,
-0.587333342112222));
#39865=CARTESIAN_POINT('Ctrl Pts',(-0.597773230616621,0.104648229800698,
-0.576712129791491));
#39866=CARTESIAN_POINT('Ctrl Pts',(-0.574922177901191,-0.194289931772878,
-0.566090917470757));
#39867=CARTESIAN_POINT('Ctrl Pts',(-0.41175127661568,-0.445808225543571,
-0.555469705150026));
#39868=CARTESIAN_POINT('Ctrl Pts',(-0.148085250655247,-0.588519198041721,
-0.544848492829293));
#39869=CARTESIAN_POINT('Ctrl Pts',(0.151723579920602,-0.587591731726026,
-0.53422728050856));
#39870=CARTESIAN_POINT('Ctrl Pts',(0.414501607921562,-0.443252191094065,
-0.523606068187829));
#39871=CARTESIAN_POINT('Ctrl Pts',(0.576113244100042,-0.190729174156685,
-0.512984855867096));
#39872=CARTESIAN_POINT('Ctrl Pts',(0.597114332253383,0.108344645017158,
-0.502363643546364));
#39873=CARTESIAN_POINT('Ctrl Pts',(0.472379188307862,0.38097505213334,-0.491742431225632));
#39874=CARTESIAN_POINT('Ctrl Pts',(0.232351613210618,0.560621811678453,
-0.481121218904899));
#39875=CARTESIAN_POINT('Ctrl Pts',(-0.0643854508469475,0.603438979194421,
-0.470500006584167));
#39876=CARTESIAN_POINT('Ctrl Pts',(-0.345408115665845,0.498976273508361,
-0.459878794263435));
#39877=CARTESIAN_POINT('Ctrl Pts',(-0.542127867956924,0.272729651259685,
-0.449257581942702));
#39878=CARTESIAN_POINT('Ctrl Pts',(-0.606531799752129,-0.0200814287731599,
-0.43863636962197));
#39879=CARTESIAN_POINT('Ctrl Pts',(-0.522901001209041,-0.307991283685645,
-0.428015157301237));
#39880=CARTESIAN_POINT('Ctrl Pts',(-0.311647036430625,-0.52073046058026,
-0.417393944980506));
#39881=CARTESIAN_POINT('Ctrl Pts',(-0.0243301430172896,-0.606376229772182,
-0.406772732659772));
#39882=CARTESIAN_POINT('Ctrl Pts',(0.268924948789863,-0.54402523821012,
-0.396151520339041));
#39883=CARTESIAN_POINT('Ctrl Pts',(0.49654418722808,-0.348895339642708,
-0.385530308018308));
#39884=CARTESIAN_POINT('Ctrl Pts',(0.602973102433286,-0.0686114103358565,
-0.374909095697576));
#39885=CARTESIAN_POINT('Ctrl Pts',(0.562235849856194,0.22841833778935,-0.364287883376844));
#39886=CARTESIAN_POINT('Ctrl Pts',(0.384275070866584,0.469698581847689,
-0.353666671056111));
#39887=CARTESIAN_POINT('Ctrl Pts',(0.112525216897816,0.596340643809236,
-0.343045458735379));
#39888=CARTESIAN_POINT('Ctrl Pts',(-0.186688391221607,0.577435305907412,
-0.332424246414646));
#39889=CARTESIAN_POINT('Ctrl Pts',(-0.440337420784613,0.417596747609107,
-0.321803034093914));
#39890=CARTESIAN_POINT('Ctrl Pts',(-0.58651437550708,0.155836374298491,
-0.311181821773182));
#39891=CARTESIAN_POINT('Ctrl Pts',(-0.589542202382296,-0.14395860117576,
-0.30056060945245));
#39892=CARTESIAN_POINT('Ctrl Pts',(-0.44868191070889,-0.408617953378765,
-0.289939397131717));
#39893=CARTESIAN_POINT('Ctrl Pts',(-0.198312919647183,-0.573546923201999,
-0.279318184810985));
#39894=CARTESIAN_POINT('Ctrl Pts',(0.100457810451271,-0.598491699957539,
-0.268696972490252));
#39895=CARTESIAN_POINT('Ctrl Pts',(0.374710067503894,-0.477364075292773,
-0.25807576016952));
#39896=CARTESIAN_POINT('Ctrl Pts',(0.557507719479534,-0.239727367437853,
-0.247454547848788));
#39897=CARTESIAN_POINT('Ctrl Pts',(0.604235901607852,0.0564190059013063,
-0.236833335528056));
#39898=CARTESIAN_POINT('Ctrl Pts',(0.503489562133039,0.338795342097125,
-0.226212123207323));
#39899=CARTESIAN_POINT('Ctrl Pts',(0.279858047502047,0.538482706593586,
-0.215590910886591));
#39900=CARTESIAN_POINT('Ctrl Pts',(-0.0120783079673112,0.606743961071895,
-0.204969698565858));
#39901=CARTESIAN_POINT('Ctrl Pts',(-0.301065603751776,0.526918614476648,
-0.194348486245126));
#39902=CARTESIAN_POINT('Ctrl Pts',(-0.516574810615386,0.318489709300428,
-0.183727273924394));
#39903=CARTESIAN_POINT('Ctrl Pts',(-0.606000393860149,0.0323274504734039,
-0.173106061603662));
#39904=CARTESIAN_POINT('Ctrl Pts',(-0.54752982679742,-0.261724193796561,
-0.162484849282929));
#39905=CARTESIAN_POINT('Ctrl Pts',(-0.355407358238332,-0.491898842808179,
-0.151863636962197));
#39906=CARTESIAN_POINT('Ctrl Pts',(-0.076576683950909,-0.602014117802982,
-0.141242424641464));
#39907=CARTESIAN_POINT('Ctrl Pts',(0.221016091685922,-0.565203769676402,
-0.130621212320732));
#39908=CARTESIAN_POINT('Ctrl Pts',(0.383330620179427,-0.448679815853072,
-0.123540404106911));
#39909=CARTESIAN_POINT('Ctrl Pts',(0.44565123783516,-0.374523575106285,
-0.12));
#39910=CARTESIAN_POINT('Ctrl Pts',(0.434231400019489,0.416939127870406,
-0.746931826162627));
#39911=CARTESIAN_POINT('Ctrl Pts',(0.36485284630267,0.489195110813665,-0.743391422055716));
#39912=CARTESIAN_POINT('Ctrl Pts',(0.189396583958067,0.598328855259381,
-0.736310613841894));
#39913=CARTESIAN_POINT('Ctrl Pts',(-0.120195278136336,0.615956064646757,
-0.725689401521163));
#39914=CARTESIAN_POINT('Ctrl Pts',(-0.40037729840512,0.483260020625564,
-0.715068189200429));
#39915=CARTESIAN_POINT('Ctrl Pts',(-0.582876337720566,0.232610561063019,
-0.704446976879698));
#39916=CARTESIAN_POINT('Ctrl Pts',(-0.623096072181431,-0.0748089500596382,
-0.693825764558965));
#39917=CARTESIAN_POINT('Ctrl Pts',(-0.511247391339576,-0.363971349880692,
-0.683204552238233));
#39918=CARTESIAN_POINT('Ctrl Pts',(-0.274615218453011,-0.564299486182443,
-0.6725833399175));
#39919=CARTESIAN_POINT('Ctrl Pts',(0.0290393028494424,-0.62690076603078,
-0.661962127596768));
#39920=CARTESIAN_POINT('Ctrl Pts',(0.325607439427196,-0.536495742218289,
-0.651340915276035));
#39921=CARTESIAN_POINT('Ctrl Pts',(0.54270477798614,-0.315149602528186,
-0.640719702955303));
#39922=CARTESIAN_POINT('Ctrl Pts',(0.627345787385518,-0.0168856283938771,
-0.630098490634571));
#39923=CARTESIAN_POINT('Ctrl Pts',(0.558871898124242,0.285499557978287,
-0.619477278313838));
#39924=CARTESIAN_POINT('Ctrl Pts',(0.353995589219439,0.518203577663625,
-0.608856065993106));
#39925=CARTESIAN_POINT('Ctrl Pts',(0.0627204062218264,0.624430914253499,
-0.598234853672375));
#39926=CARTESIAN_POINT('Ctrl Pts',(-0.243862773535938,0.578254930262477,
-0.587613641351641));
#39927=CARTESIAN_POINT('Ctrl Pts',(-0.490926973266102,0.390945680789826,
-0.576992429030909));
#39928=CARTESIAN_POINT('Ctrl Pts',(-0.618171824566399,0.108219277545785,
-0.566371216710177));
#39929=CARTESIAN_POINT('Ctrl Pts',(-0.594540995638531,-0.200919939982977,
-0.555750004389445));
#39930=CARTESIAN_POINT('Ctrl Pts',(-0.425802001321639,-0.461021119842892,
-0.545128792068712));
#39931=CARTESIAN_POINT('Ctrl Pts',(-0.153138556396207,-0.60860200459383,
-0.53450757974798));
#39932=CARTESIAN_POINT('Ctrl Pts',(0.156901041106368,-0.607642889137947,
-0.523886367427247));
#39933=CARTESIAN_POINT('Ctrl Pts',(0.428646185762228,-0.458377862503188,
-0.513265155106516));
#39934=CARTESIAN_POINT('Ctrl Pts',(0.595772706139457,-0.197237674000322,
-0.502643942785783));
#39935=CARTESIAN_POINT('Ctrl Pts',(0.617490441756758,0.112041830349559,
-0.492022730465051));
#39936=CARTESIAN_POINT('Ctrl Pts',(0.488498798151678,0.393975559676054,
-0.481401518144319));
#39937=CARTESIAN_POINT('Ctrl Pts',(0.240280449713669,0.579752639407259,
-0.470780305823586));
#39938=CARTESIAN_POINT('Ctrl Pts',(-0.0665825593838184,0.624030912856886,
-0.460159093502854));
#39939=CARTESIAN_POINT('Ctrl Pts',(-0.357194926345134,0.516003490306564,
-0.449537881182121));
#39940=CARTESIAN_POINT('Ctrl Pts',(-0.560627602774265,0.282036360107072,
-0.438916668861389));
#39941=CARTESIAN_POINT('Ctrl Pts',(-0.627229273755788,-0.0207666935031524,
-0.428295456540656));
#39942=CARTESIAN_POINT('Ctrl Pts',(-0.540744632628591,-0.318501271109293,
-0.417674244219924));
#39943=CARTESIAN_POINT('Ctrl Pts',(-0.322281773863149,-0.538500023816976,
-0.407053031899192));
#39944=CARTESIAN_POINT('Ctrl Pts',(-0.0251603921531334,-0.627068395058943,
-0.39643181957846));
#39945=CARTESIAN_POINT('Ctrl Pts',(0.278101824823055,-0.562589719462036,
-0.385810607257727));
#39946=CARTESIAN_POINT('Ctrl Pts',(0.513488410780781,-0.36080114940438,
-0.375189394936995));
#39947=CARTESIAN_POINT('Ctrl Pts',(0.623549138376695,-0.0709527267884497,
-0.364568182616262));
#39948=CARTESIAN_POINT('Ctrl Pts',(0.581421755510406,0.236212954016045,
-0.35394697029553));
#39949=CARTESIAN_POINT('Ctrl Pts',(0.397388189243505,0.485726717868459,
-0.343325757974798));
#39950=CARTESIAN_POINT('Ctrl Pts',(0.116365061325512,0.616690351734874,
-0.332704545654065));
#39951=CARTESIAN_POINT('Ctrl Pts',(-0.193059002170075,0.597139882382544,
-0.322083333333333));
#39952=CARTESIAN_POINT('Ctrl Pts',(-0.455363627692896,0.431846944929651,
-0.311462121012601));
#39953=CARTESIAN_POINT('Ctrl Pts',(-0.606528768890564,0.161154181719611,
-0.300840908691869));
#39954=CARTESIAN_POINT('Ctrl Pts',(-0.609659918242957,-0.148871087885701,
-0.290219696371136));
#39955=CARTESIAN_POINT('Ctrl Pts',(-0.463992867507207,-0.422561755617893,
-0.279598484050404));
#39956=CARTESIAN_POINT('Ctrl Pts',(-0.205080209508431,-0.593118811333345,
-0.268977271729672));
#39957=CARTESIAN_POINT('Ctrl Pts',(0.10388586306307,-0.618914811171724,
-0.258356059408939));
#39958=CARTESIAN_POINT('Ctrl Pts',(0.387496786822224,-0.493653790923003,
-0.247734847088207));
#39959=CARTESIAN_POINT('Ctrl Pts',(0.576532280987245,-0.247907896401938,
-0.237113634767475));
#39960=CARTESIAN_POINT('Ctrl Pts',(0.624855029691027,0.058344265068974,
-0.226492422446742));
#39961=CARTESIAN_POINT('Ctrl Pts',(0.520670791753022,0.35035649649741,-0.21587121012601));
#39962=CARTESIAN_POINT('Ctrl Pts',(0.289408007892015,0.55685805282555,-0.205249997805277));
#39963=CARTESIAN_POINT('Ctrl Pts',(-0.0124904717899899,0.627448674932399,
-0.194628785484545));
#39964=CARTESIAN_POINT('Ctrl Pts',(-0.311339257185273,0.544899344142648,
-0.184007573163813));
#39965=CARTESIAN_POINT('Ctrl Pts',(-0.534202565199775,0.329357948165023,
-0.17338636084308));
#39966=CARTESIAN_POINT('Ctrl Pts',(-0.626679734008933,0.0334306021400623,
-0.162765148522348));
#39967=CARTESIAN_POINT('Ctrl Pts',(-0.566213899686921,-0.270655349095339,
-0.152143936201616));
#39968=CARTESIAN_POINT('Ctrl Pts',(-0.36753538608593,-0.508684547227327,
-0.141522723880884));
#39969=CARTESIAN_POINT('Ctrl Pts',(-0.0791898098018671,-0.622557429065733,
-0.130901511560151));
#39970=CARTESIAN_POINT('Ctrl Pts',(0.228558111434812,-0.584490953521386,
-0.120280299239419));
#39971=CARTESIAN_POINT('Ctrl Pts',(0.396411509836348,-0.463990701165897,
-0.113199491025597));
#39972=CARTESIAN_POINT('Ctrl Pts',(0.460858775038588,-0.387303930501811,
-0.109659086918687));
#39973=CARTESIAN_POINT('Ctrl Pts',(0.44856028020657,0.430697393183078,-0.736590913081313));
#39974=CARTESIAN_POINT('Ctrl Pts',(0.376892355007826,0.505337697763021,
-0.733050508974403));
#39975=CARTESIAN_POINT('Ctrl Pts',(0.195646341481949,0.618072665769401,
-0.725969700760581));
#39976=CARTESIAN_POINT('Ctrl Pts',(-0.124161513050235,0.63628154237691,
-0.715348488439849));
#39977=CARTESIAN_POINT('Ctrl Pts',(-0.41358905218022,0.499206759931933,
-0.704727276119116));
#39978=CARTESIAN_POINT('Ctrl Pts',(-0.60211024205523,0.240286304594168,
-0.694106063798384));
#39979=CARTESIAN_POINT('Ctrl Pts',(-0.643657157729202,-0.0772775151663482,
-0.683484851477652));
#39980=CARTESIAN_POINT('Ctrl Pts',(-0.528117665152417,-0.375981770738642,
-0.672863639156919));
#39981=CARTESIAN_POINT('Ctrl Pts',(-0.283677042546308,-0.582920386759363,
-0.662242426836187));
#39982=CARTESIAN_POINT('Ctrl Pts',(0.0299975492849321,-0.647587399851459,
-0.651621214515455));
#39983=CARTESIAN_POINT('Ctrl Pts',(0.336351918033223,-0.55419916765178,
-0.641000002194723));
#39984=CARTESIAN_POINT('Ctrl Pts',(0.5606130907898,-0.325548990724041,-0.63037878987399));
#39985=CARTESIAN_POINT('Ctrl Pts',(0.648047106136105,-0.0174428247323467,
-0.619757577553258));
#39986=CARTESIAN_POINT('Ctrl Pts',(0.577313697744881,0.294920546325864,
-0.609136365232525));
#39987=CARTESIAN_POINT('Ctrl Pts',(0.36567682734375,0.535303393514173,-0.598515152911793));
#39988=CARTESIAN_POINT('Ctrl Pts',(0.0647900704285079,0.645036047265636,
-0.587893940591061));
#39989=CARTESIAN_POINT('Ctrl Pts',(-0.25190982048816,0.597336336197074,
-0.577272728270329));
#39990=CARTESIAN_POINT('Ctrl Pts',(-0.507126708661149,0.40384620760443,
-0.566651515949596));
#39991=CARTESIAN_POINT('Ctrl Pts',(-0.638570418516177,0.111790325290873,
-0.556030303628864));
#39992=CARTESIAN_POINT('Ctrl Pts',(-0.614159813375872,-0.207549948193075,
-0.545409091308131));
#39993=CARTESIAN_POINT('Ctrl Pts',(-0.439852726027598,-0.476234014142214,
-0.534787878987399));
#39994=CARTESIAN_POINT('Ctrl Pts',(-0.158191862137167,-0.628684811145938,
-0.524166666666666));
#39995=CARTESIAN_POINT('Ctrl Pts',(0.162078502292133,-0.627694046549866,
-0.513545454345935));
#39996=CARTESIAN_POINT('Ctrl Pts',(0.442790763602892,-0.473503533912313,
-0.502924242025202));
#39997=CARTESIAN_POINT('Ctrl Pts',(0.615432168178873,-0.203746173843959,
-0.49230302970447));
#39998=CARTESIAN_POINT('Ctrl Pts',(0.637866551260131,0.11573901568196,-0.481681817383737));
#39999=CARTESIAN_POINT('Ctrl Pts',(0.504618407995495,0.406976067218768,
-0.471060605063006));
#40000=CARTESIAN_POINT('Ctrl Pts',(0.248209286216719,0.598883467136063,
-0.460439392742272));
#40001=CARTESIAN_POINT('Ctrl Pts',(-0.0687796679206887,0.644622846519354,
-0.449818180421541));
#40002=CARTESIAN_POINT('Ctrl Pts',(-0.368981737024425,0.533030707104764,
-0.439196968100808));
#40003=CARTESIAN_POINT('Ctrl Pts',(-0.579127337591605,0.291343068954459,
-0.428575755780076));
#40004=CARTESIAN_POINT('Ctrl Pts',(-0.64792674775945,-0.021451958233145,
-0.417954543459343));
#40005=CARTESIAN_POINT('Ctrl Pts',(-0.558588264048139,-0.329011258532942,
-0.407333331138611));
#40006=CARTESIAN_POINT('Ctrl Pts',(-0.332916511295674,-0.556269587053691,
-0.396712118817879));
#40007=CARTESIAN_POINT('Ctrl Pts',(-0.0259906412889762,-0.647760560345705,
-0.386090906497146));
#40008=CARTESIAN_POINT('Ctrl Pts',(0.287278700856247,-0.581154200713952,
-0.375469694176414));
#40009=CARTESIAN_POINT('Ctrl Pts',(0.530432634333482,-0.372706959166052,
-0.364848481855682));
#40010=CARTESIAN_POINT('Ctrl Pts',(0.644125174320103,-0.0732940432410428,
-0.354227269534949));
#40011=CARTESIAN_POINT('Ctrl Pts',(0.600607661164621,0.24400757024274,-0.343606057214217));
#40012=CARTESIAN_POINT('Ctrl Pts',(0.410501307620425,0.501754853889229,
-0.332984844893485));
#40013=CARTESIAN_POINT('Ctrl Pts',(0.120204905753208,0.637040059660513,
-0.322363632572752));
#40014=CARTESIAN_POINT('Ctrl Pts',(-0.199429613118542,0.616844458857675,
-0.31174242025202));
#40015=CARTESIAN_POINT('Ctrl Pts',(-0.470389834601179,0.446097142250195,
-0.301121207931288));
#40016=CARTESIAN_POINT('Ctrl Pts',(-0.626543162274047,0.166471989140732,
-0.290499995610555));
#40017=CARTESIAN_POINT('Ctrl Pts',(-0.629777634103618,-0.153783574595641,
-0.279878783289823));
#40018=CARTESIAN_POINT('Ctrl Pts',(-0.479303824305524,-0.436505557857022,
-0.269257570969091));
#40019=CARTESIAN_POINT('Ctrl Pts',(-0.211847499369681,-0.612690699464692,
-0.258636358648358));
#40020=CARTESIAN_POINT('Ctrl Pts',(0.107313915674871,-0.639337922385911,
-0.248015146327626));
#40021=CARTESIAN_POINT('Ctrl Pts',(0.400283506140554,-0.509943506553232,
-0.237393934006894));
#40022=CARTESIAN_POINT('Ctrl Pts',(0.595556842494959,-0.256088425366023,
-0.226772721686161));
#40023=CARTESIAN_POINT('Ctrl Pts',(0.6454741577742,0.0602695242366418,-0.216151509365429));
#40024=CARTESIAN_POINT('Ctrl Pts',(0.537852021373006,0.361917650897694,
-0.205530297044696));
#40025=CARTESIAN_POINT('Ctrl Pts',(0.298957968281983,0.575233399057514,
-0.194909084723964));
#40026=CARTESIAN_POINT('Ctrl Pts',(-0.0129026356126682,0.648153388792901,
-0.184287872403232));
#40027=CARTESIAN_POINT('Ctrl Pts',(-0.321612910618771,0.562880073808648,
-0.1736666600825));
#40028=CARTESIAN_POINT('Ctrl Pts',(-0.551830319784164,0.340226187029618,
-0.163045447761767));
#40029=CARTESIAN_POINT('Ctrl Pts',(-0.647359074157716,0.0345337538067202,
-0.152424235441035));
#40030=CARTESIAN_POINT('Ctrl Pts',(-0.584897972576422,-0.279586504394117,
-0.141803023120302));
#40031=CARTESIAN_POINT('Ctrl Pts',(-0.379663413933528,-0.525470251646476,
-0.131181810799571));
#40032=CARTESIAN_POINT('Ctrl Pts',(-0.0818029356528252,-0.643100740328482,
-0.120560598478838));
#40033=CARTESIAN_POINT('Ctrl Pts',(0.236100131183702,-0.603778137366371,
-0.109939386158106));
#40034=CARTESIAN_POINT('Ctrl Pts',(0.409492399493268,-0.479301586478722,
-0.102858577944284));
#40035=CARTESIAN_POINT('Ctrl Pts',(0.476066312242016,-0.400084285897338,
-0.0993181738373734));
#40036=CARTESIAN_POINT('Ctrl Pts',(0.462889160393651,0.44445565849575,-0.72625));
#40037=CARTESIAN_POINT('Ctrl Pts',(0.388931863712981,0.521480284712376,
-0.722709595893089));
#40038=CARTESIAN_POINT('Ctrl Pts',(0.20189609900583,0.63781647627942,-0.715628787679269));
#40039=CARTESIAN_POINT('Ctrl Pts',(-0.128127747964134,0.656607020107064,
-0.705007575358535));
#40040=CARTESIAN_POINT('Ctrl Pts',(-0.42680080595532,0.515153499238301,
-0.694386363037804));
#40041=CARTESIAN_POINT('Ctrl Pts',(-0.621344146389896,0.247962048125318,
-0.68376515071707));
#40042=CARTESIAN_POINT('Ctrl Pts',(-0.664218243276972,-0.0797460802730583,
-0.673143938396339));
#40043=CARTESIAN_POINT('Ctrl Pts',(-0.544987938965259,-0.387992191596592,
-0.662522726075605));
#40044=CARTESIAN_POINT('Ctrl Pts',(-0.292738866639604,-0.601541287336283,
-0.651901513754874));
#40045=CARTESIAN_POINT('Ctrl Pts',(0.0309557957204211,-0.66827403367214,
-0.641280301434142));
#40046=CARTESIAN_POINT('Ctrl Pts',(0.34709639663925,-0.571902593085269,
-0.630659089113409));
#40047=CARTESIAN_POINT('Ctrl Pts',(0.578521403593459,-0.335948378919897,
-0.620037876792677));
#40048=CARTESIAN_POINT('Ctrl Pts',(0.668748424886692,-0.018000021070816,
-0.609416664471945));
#40049=CARTESIAN_POINT('Ctrl Pts',(0.59575549736552,0.30434153467344,-0.598795452151212));
#40050=CARTESIAN_POINT('Ctrl Pts',(0.377358065468061,0.552403209364722,
-0.58817423983048));
#40051=CARTESIAN_POINT('Ctrl Pts',(0.0668597346351892,0.665641180277773,
-0.577553027509748));
#40052=CARTESIAN_POINT('Ctrl Pts',(-0.259956867440381,0.61641774213167,
-0.566931815189015));
#40053=CARTESIAN_POINT('Ctrl Pts',(-0.523326444056197,0.416746734419033,
-0.556310602868283));
#40054=CARTESIAN_POINT('Ctrl Pts',(-0.658969012465955,0.115361373035961,
-0.54568939054755));
#40055=CARTESIAN_POINT('Ctrl Pts',(-0.633778631113213,-0.214179956403173,
-0.535068178226818));
#40056=CARTESIAN_POINT('Ctrl Pts',(-0.453903450733557,-0.491446908441536,
-0.524446965906085));
#40057=CARTESIAN_POINT('Ctrl Pts',(-0.163245167878128,-0.648767617698046,
-0.513825753585354));
#40058=CARTESIAN_POINT('Ctrl Pts',(0.167255963477899,-0.647745203961788,
-0.50320454126462));
#40059=CARTESIAN_POINT('Ctrl Pts',(0.456935341443556,-0.488629205321436,
-0.492583328943889));
#40060=CARTESIAN_POINT('Ctrl Pts',(0.635091630218289,-0.210254673687596,
-0.481962116623156));
#40061=CARTESIAN_POINT('Ctrl Pts',(0.658242660763504,0.119436201014362,
-0.471340904302425));
#40062=CARTESIAN_POINT('Ctrl Pts',(0.520738017839312,0.419976574761482,
-0.460719691981691));
#40063=CARTESIAN_POINT('Ctrl Pts',(0.256138122719768,0.618014294864869,
-0.45009847966096));
#40064=CARTESIAN_POINT('Ctrl Pts',(-0.0709767764575589,0.66521478018182,
-0.439477267340227));
#40065=CARTESIAN_POINT('Ctrl Pts',(-0.380768547703715,0.550057923902966,
-0.428856055019495));
#40066=CARTESIAN_POINT('Ctrl Pts',(-0.597627072408945,0.300649777801846,
-0.418234842698762));
#40067=CARTESIAN_POINT('Ctrl Pts',(-0.668624221763112,-0.0221372229631371,
-0.40761363037803));
#40068=CARTESIAN_POINT('Ctrl Pts',(-0.576431895467687,-0.339521245956591,
-0.396992418057298));
#40069=CARTESIAN_POINT('Ctrl Pts',(-0.343551248728199,-0.574039150290406,
-0.386371205736565));
#40070=CARTESIAN_POINT('Ctrl Pts',(-0.0268208904248193,-0.668452725632466,
-0.375749993415833));
#40071=CARTESIAN_POINT('Ctrl Pts',(0.296455576889439,-0.599718681965868,
-0.365128781095101));
#40072=CARTESIAN_POINT('Ctrl Pts',(0.547376857886183,-0.384612768927724,
-0.354507568774369));
#40073=CARTESIAN_POINT('Ctrl Pts',(0.664701210263511,-0.0756353596936366,
-0.343886356453636));
#40074=CARTESIAN_POINT('Ctrl Pts',(0.619793566818835,0.251802186469436,
-0.333265144132904));
#40075=CARTESIAN_POINT('Ctrl Pts',(0.423614425997345,0.517782989909997,
-0.322643931812171));
#40076=CARTESIAN_POINT('Ctrl Pts',(0.124044750180905,0.657389767586153,
-0.312022719491439));
#40077=CARTESIAN_POINT('Ctrl Pts',(-0.20580022406701,0.636549035332806,
-0.301401507170707));
#40078=CARTESIAN_POINT('Ctrl Pts',(-0.485416041509462,0.46034733957074,
-0.290780294849974));
#40079=CARTESIAN_POINT('Ctrl Pts',(-0.64655755565753,0.171789796561853,
-0.280159082529243));
#40080=CARTESIAN_POINT('Ctrl Pts',(-0.649895349964279,-0.158696061305582,
-0.26953787020851));
#40081=CARTESIAN_POINT('Ctrl Pts',(-0.49461478110384,-0.45044936009615,
-0.258916657887777));
#40082=CARTESIAN_POINT('Ctrl Pts',(-0.218614789230929,-0.632262587596038,
-0.248295445567045));
#40083=CARTESIAN_POINT('Ctrl Pts',(0.11074196828667,-0.659761033600097,
-0.237674233246313));
#40084=CARTESIAN_POINT('Ctrl Pts',(0.413070225458884,-0.526233222183462,
-0.22705302092558));
#40085=CARTESIAN_POINT('Ctrl Pts',(0.614581404002671,-0.264268954330109,
-0.216431808604848));
#40086=CARTESIAN_POINT('Ctrl Pts',(0.666093285857374,0.0621947834043098,
-0.205810596284116));
#40087=CARTESIAN_POINT('Ctrl Pts',(0.555033250992989,0.373478805297979,
-0.195189383963383));
#40088=CARTESIAN_POINT('Ctrl Pts',(0.308507928671951,0.593608745289479,
-0.184568171642651));
#40089=CARTESIAN_POINT('Ctrl Pts',(-0.0133147994353463,0.668858102653405,
-0.173946959321918));
#40090=CARTESIAN_POINT('Ctrl Pts',(-0.331886564052269,0.580860803474647,
-0.163325747001187));
#40091=CARTESIAN_POINT('Ctrl Pts',(-0.569458074368552,0.351094425894214,
-0.152704534680454));
#40092=CARTESIAN_POINT('Ctrl Pts',(-0.668038414306502,0.0356369054733784,
-0.142083322359722));
#40093=CARTESIAN_POINT('Ctrl Pts',(-0.603582045465921,-0.288517659692895,
-0.131462110038989));
#40094=CARTESIAN_POINT('Ctrl Pts',(-0.391791441781126,-0.542255956065624,
-0.120840897718257));
#40095=CARTESIAN_POINT('Ctrl Pts',(-0.084416061503783,-0.663644051591233,
-0.110219685397525));
#40096=CARTESIAN_POINT('Ctrl Pts',(0.243642150932592,-0.623065321211354,
-0.0995984730767924));
#40097=CARTESIAN_POINT('Ctrl Pts',(0.422573289150189,-0.494612471791547,
-0.0925176648629709));
#40098=CARTESIAN_POINT('Ctrl Pts',(0.491273849445444,-0.412864641292864,
-0.0889772607560602));
#40099=CARTESIAN_POINT('',(0.445651237835157,-0.374523575106288,-0.12));
#40100=CARTESIAN_POINT('Ctrl Pts',(-0.355015686975108,-0.534630012137314,
-0.12));
#40101=CARTESIAN_POINT('Ctrl Pts',(-0.327773074693179,-0.55029714351302,
-0.12));
#40102=CARTESIAN_POINT('Ctrl Pts',(-0.299464346019529,-0.563882057522015,
-0.12));
#40103=CARTESIAN_POINT('Ctrl Pts',(-0.270342974496624,-0.575326154153575,
-0.12));
#40104=CARTESIAN_POINT('Ctrl Pts',(-0.239781266261733,-0.587336273319513,
-0.12));
#40105=CARTESIAN_POINT('Ctrl Pts',(-0.208323126958149,-0.596989401715483,
-0.12));
#40106=CARTESIAN_POINT('Ctrl Pts',(-0.176246299508229,-0.604158357140015,
-0.12));
#40107=CARTESIAN_POINT('Ctrl Pts',(-0.161891963957468,-0.607366454694951,
-0.12));
#40108=CARTESIAN_POINT('Ctrl Pts',(-0.147413669750131,-0.610076237005704,
-0.12));
#40109=CARTESIAN_POINT('Ctrl Pts',(-0.132836594213696,-0.612272034267081,
-0.12));
#40110=CARTESIAN_POINT('Ctrl Pts',(-0.124920402928789,-0.613464478602056,
-0.12));
#40111=CARTESIAN_POINT('Ctrl Pts',(-0.116973279753054,-0.61450528464571,
-0.12));
#40112=CARTESIAN_POINT('Ctrl Pts',(-0.10902091463483,-0.615389836202277,
-0.12));
#40113=CARTESIAN_POINT('Ctrl Pts',(-0.0988935419311309,-0.616516316583374,
-0.12));
#40114=CARTESIAN_POINT('Ctrl Pts',(-0.0887499005304207,-0.617390725698137,
-0.12));
#40115=CARTESIAN_POINT('Ctrl Pts',(-0.0785983814394652,-0.61801027904089,
-0.12));
#40116=CARTESIAN_POINT('Ctrl Pts',(-0.0478707602737524,-0.61988560432349,
-0.12));
#40117=CARTESIAN_POINT('Ctrl Pts',(-0.0170704984466291,-0.619429816208118,
-0.12));
#40118=CARTESIAN_POINT('Ctrl Pts',(0.0135460552793042,-0.616696753535392,
-0.12));
#40119=CARTESIAN_POINT('Ctrl Pts',(0.0363940854309653,-0.614657167404575,
-0.12));
#40120=CARTESIAN_POINT('Ctrl Pts',(0.0591399790301594,-0.611348192348154,
-0.12));
#40121=CARTESIAN_POINT('Ctrl Pts',(0.0816716129165091,-0.606774115783264,
-0.12));
#40122=CARTESIAN_POINT('Ctrl Pts',(0.0917546790591232,-0.604727184043747,
-0.12));
#40123=CARTESIAN_POINT('Ctrl Pts',(0.101794739333339,-0.602426702231052,
-0.12));
#40124=CARTESIAN_POINT('Ctrl Pts',(0.111781158534424,-0.599872121726624,
-0.12));
#40125=CARTESIAN_POINT('Ctrl Pts',(0.118182233540509,-0.598234691824207,
-0.12));
#40126=CARTESIAN_POINT('Ctrl Pts',(0.124557115310639,-0.59649382554347,
-0.12));
#40127=CARTESIAN_POINT('Ctrl Pts',(0.130895502574684,-0.594652107438951,
-0.12));
#40128=CARTESIAN_POINT('Ctrl Pts',(0.16128528154991,-0.585821879212206,
-0.12));
#40129=CARTESIAN_POINT('Ctrl Pts',(0.190892183977264,-0.574664264569325,
-0.12));
#40130=CARTESIAN_POINT('Ctrl Pts',(0.21942623032083,-0.561211828032157,
-0.12));
#40131=CARTESIAN_POINT('Ctrl Pts',(0.241737226557842,-0.550693261637977,
-0.12));
#40132=CARTESIAN_POINT('Ctrl Pts',(0.263392112795318,-0.53877018802294,
-0.12));
#40133=CARTESIAN_POINT('Ctrl Pts',(0.284272054715151,-0.525522446725764,
-0.12));
#40134=CARTESIAN_POINT('Ctrl Pts',(0.29057737878399,-0.521521894311416,
-0.12));
#40135=CARTESIAN_POINT('Ctrl Pts',(0.296813196360162,-0.517399549803865,
-0.12));
#40136=CARTESIAN_POINT('Ctrl Pts',(0.302971897916213,-0.513160117534818,
-0.12));
#40137=CARTESIAN_POINT('Ctrl Pts',(0.327487947260565,-0.496284136493344,
-0.12));
#40138=CARTESIAN_POINT('Ctrl Pts',(0.350669698473764,-0.477636222421621,
-0.12));
#40139=CARTESIAN_POINT('Ctrl Pts',(0.372326859018955,-0.457378924688331,
-0.12));
#40140=CARTESIAN_POINT('Ctrl Pts',(0.393597599384017,-0.43748306993473,
-0.12));
#40141=CARTESIAN_POINT('Ctrl Pts',(0.413398440600423,-0.416033780451133,
-0.12));
#40142=CARTESIAN_POINT('Ctrl Pts',(0.431509449154427,-0.393155467378397,
-0.12));
#40143=CARTESIAN_POINT('Ctrl Pts',(0.43634572983353,-0.387046147560331,
-0.12));
#40144=CARTESIAN_POINT('Ctrl Pts',(0.441061254550602,-0.380834805043548,
-0.12));
#40145=CARTESIAN_POINT('Ctrl Pts',(0.44565123783516,-0.374523575106285,
-0.12));
#40146=CARTESIAN_POINT('',(-0.353390396098499,0.46258854508056,-0.72625));
#40147=CARTESIAN_POINT('Ctrl Pts',(-0.353420490498553,0.462617301267147,
-0.72625));
#40148=CARTESIAN_POINT('Ctrl Pts',(-0.331343914475331,0.482052117168188,
-0.72625));
#40149=CARTESIAN_POINT('Ctrl Pts',(-0.307843201132015,0.499732456588995,
-0.72625));
#40150=CARTESIAN_POINT('Ctrl Pts',(-0.283172855491956,0.515579930268511,
-0.72625));
#40151=CARTESIAN_POINT('Ctrl Pts',(-0.257338168972133,0.53217534083206,
-0.72625));
#40152=CARTESIAN_POINT('Ctrl Pts',(-0.230219925034403,0.546761932985982,
-0.72625));
#40153=CARTESIAN_POINT('Ctrl Pts',(-0.202067218313667,0.559208190060778,
-0.72625));
#40154=CARTESIAN_POINT('Ctrl Pts',(-0.195896923741982,0.561936065331465,
-0.72625));
#40155=CARTESIAN_POINT('Ctrl Pts',(-0.189676811570407,0.564560935846749,
-0.72625));
#40156=CARTESIAN_POINT('Ctrl Pts',(-0.183409317371435,0.567081079046547,
-0.72625));
#40157=CARTESIAN_POINT('Ctrl Pts',(-0.176798752551787,0.569739170055198,
-0.72625));
#40158=CARTESIAN_POINT('Ctrl Pts',(-0.17014384257185,0.572277351670826,
-0.72625));
#40159=CARTESIAN_POINT('Ctrl Pts',(-0.163450714977005,0.574693394083012,
-0.72625));
#40160=CARTESIAN_POINT('Ctrl Pts',(-0.147536270437225,0.580438088537081,
-0.72625));
#40161=CARTESIAN_POINT('Ctrl Pts',(-0.131400896704278,0.585494582417171,
-0.72625));
#40162=CARTESIAN_POINT('Ctrl Pts',(-0.115087389998091,0.589845129045876,
-0.72625));
#40163=CARTESIAN_POINT('Ctrl Pts',(-0.0904845801913842,0.59640629784845,
-0.72625));
#40164=CARTESIAN_POINT('Ctrl Pts',(-0.065476953188039,0.601363175763682,
-0.72625));
#40165=CARTESIAN_POINT('Ctrl Pts',(-0.040220969016932,0.604734997002558,
-0.72625));
#40166=CARTESIAN_POINT('Ctrl Pts',(-0.0232728051723021,0.60699767575719,
-0.72625));
#40167=CARTESIAN_POINT('Ctrl Pts',(-0.00621251576441358,0.608546060010427,
-0.72625));
#40168=CARTESIAN_POINT('Ctrl Pts',(0.0109143171267901,0.609379421018909,
-0.72625));
#40169=CARTESIAN_POINT('Ctrl Pts',(0.0179713338528023,0.60972280281127,
-0.72625));
#40170=CARTESIAN_POINT('Ctrl Pts',(0.0250400715171394,0.609944566997145,
-0.72625));
#40171=CARTESIAN_POINT('Ctrl Pts',(0.0321018300265921,0.610044668541972,
-0.72625));
#40172=CARTESIAN_POINT('Ctrl Pts',(0.0629203426176338,0.610481525836862,
-0.72625));
#40173=CARTESIAN_POINT('Ctrl Pts',(0.0936755695308824,0.608609614963221,
-0.72625));
#40174=CARTESIAN_POINT('Ctrl Pts',(0.124099989476803,0.60446798569458,-0.72625));
#40175=CARTESIAN_POINT('Ctrl Pts',(0.14542332482861,0.601565273006711,-0.72625));
#40176=CARTESIAN_POINT('Ctrl Pts',(0.166584716115012,0.597546610890188,
-0.72625));
#40177=CARTESIAN_POINT('Ctrl Pts',(0.187494048945749,0.592410339560903,
-0.72625));
#40178=CARTESIAN_POINT('Ctrl Pts',(0.202188505813513,0.588800720922169,
-0.72625));
#40179=CARTESIAN_POINT('Ctrl Pts',(0.216758501690732,0.584638862439533,
-0.72625));
#40180=CARTESIAN_POINT('Ctrl Pts',(0.231178697027477,0.579939611265494,
-0.72625));
#40181=CARTESIAN_POINT('Ctrl Pts',(0.238102595557612,0.577683252212315,
-0.72625));
#40182=CARTESIAN_POINT('Ctrl Pts',(0.244991946660547,0.575302954377583,
-0.72625));
#40183=CARTESIAN_POINT('Ctrl Pts',(0.251843864110581,0.572800121359829,
-0.72625));
#40184=CARTESIAN_POINT('Ctrl Pts',(0.258582145288071,0.570338796812808,
-0.72625));
#40185=CARTESIAN_POINT('Ctrl Pts',(0.265277205063595,0.567761447216236,
-0.72625));
#40186=CARTESIAN_POINT('Ctrl Pts',(0.271920132877671,0.565072819537037,
-0.72625));
#40187=CARTESIAN_POINT('Ctrl Pts',(0.30080227087538,0.553383197456466,-0.72625));
#40188=CARTESIAN_POINT('Ctrl Pts',(0.328737399818583,0.539580421272658,
-0.72625));
#40189=CARTESIAN_POINT('Ctrl Pts',(0.355518167806567,0.523830055574735,
-0.72625));
#40190=CARTESIAN_POINT('Ctrl Pts',(0.382426618369393,0.508004596912789,
-0.72625));
#40191=CARTESIAN_POINT('Ctrl Pts',(0.408170864031784,0.490212434749928,
-0.72625));
#40192=CARTESIAN_POINT('Ctrl Pts',(0.432524619771516,0.470572470283676,
-0.72625));
#40193=CARTESIAN_POINT('Ctrl Pts',(0.442905486761684,0.462200872038434,
-0.72625));
#40194=CARTESIAN_POINT('Ctrl Pts',(0.45303341106848,0.453492981462904,-0.72625));
#40195=CARTESIAN_POINT('Ctrl Pts',(0.46288916039365,0.444455658495751,-0.72625));
#40196=CARTESIAN_POINT('Ctrl Pts',(-0.353420490498551,0.462617301267149,
-0.72625));
#40197=CARTESIAN_POINT('Ctrl Pts',(-0.359516126172293,0.457966781316138,
-0.725969700760581));
#40198=CARTESIAN_POINT('Ctrl Pts',(-0.441333858628395,0.392916952001327,
-0.722148997414251));
#40199=CARTESIAN_POINT('Ctrl Pts',(-0.5636424333859,0.224934817531868,-0.714787889961011));
#40200=CARTESIAN_POINT('Ctrl Pts',(-0.602534986633661,-0.0723403849529277,
-0.704166677640278));
#40201=CARTESIAN_POINT('Ctrl Pts',(-0.494377117526733,-0.351960929022743,
-0.693545465319546));
#40202=CARTESIAN_POINT('Ctrl Pts',(-0.265553394359715,-0.545678585605523,
-0.682924252998813));
#40203=CARTESIAN_POINT('Ctrl Pts',(0.0280810564139534,-0.606214132210099,
-0.672303040678082));
#40204=CARTESIAN_POINT('Ctrl Pts',(0.314862960821169,-0.518792316784799,
-0.661681828357348));
#40205=CARTESIAN_POINT('Ctrl Pts',(0.524796465182481,-0.30475021433233,
-0.651060616036617));
#40206=CARTESIAN_POINT('Ctrl Pts',(0.60664446863493,-0.0163284320554081,
-0.640439403715884));
#40207=CARTESIAN_POINT('Ctrl Pts',(0.540430098503603,0.27607856963071,-0.629818191395151));
#40208=CARTESIAN_POINT('Ctrl Pts',(0.342314351095128,0.501103761813076,
-0.619196979074419));
#40209=CARTESIAN_POINT('Ctrl Pts',(0.0606507420151454,0.603825781241362,
-0.608575766753688));
#40210=CARTESIAN_POINT('Ctrl Pts',(-0.235815726583716,0.55917352432788,
-0.597954554432955));
#40211=CARTESIAN_POINT('Ctrl Pts',(-0.474727237871055,0.378045153975223,
-0.587333342112222));
#40212=CARTESIAN_POINT('Ctrl Pts',(-0.597773230616621,0.104648229800698,
-0.576712129791491));
#40213=CARTESIAN_POINT('Ctrl Pts',(-0.574922177901191,-0.194289931772878,
-0.566090917470757));
#40214=CARTESIAN_POINT('Ctrl Pts',(-0.41175127661568,-0.445808225543571,
-0.555469705150026));
#40215=CARTESIAN_POINT('Ctrl Pts',(-0.148085250655247,-0.588519198041721,
-0.544848492829293));
#40216=CARTESIAN_POINT('Ctrl Pts',(0.151723579920602,-0.587591731726026,
-0.53422728050856));
#40217=CARTESIAN_POINT('Ctrl Pts',(0.414501607921562,-0.443252191094065,
-0.523606068187829));
#40218=CARTESIAN_POINT('Ctrl Pts',(0.576113244100042,-0.190729174156685,
-0.512984855867096));
#40219=CARTESIAN_POINT('Ctrl Pts',(0.597114332253383,0.108344645017158,
-0.502363643546364));
#40220=CARTESIAN_POINT('Ctrl Pts',(0.472379188307862,0.38097505213334,-0.491742431225632));
#40221=CARTESIAN_POINT('Ctrl Pts',(0.232351613210618,0.560621811678453,
-0.481121218904899));
#40222=CARTESIAN_POINT('Ctrl Pts',(-0.0643854508469475,0.603438979194421,
-0.470500006584167));
#40223=CARTESIAN_POINT('Ctrl Pts',(-0.345408115665845,0.498976273508361,
-0.459878794263435));
#40224=CARTESIAN_POINT('Ctrl Pts',(-0.542127867956924,0.272729651259685,
-0.449257581942702));
#40225=CARTESIAN_POINT('Ctrl Pts',(-0.606531799752129,-0.0200814287731599,
-0.43863636962197));
#40226=CARTESIAN_POINT('Ctrl Pts',(-0.522901001209041,-0.307991283685645,
-0.428015157301237));
#40227=CARTESIAN_POINT('Ctrl Pts',(-0.311647036430625,-0.52073046058026,
-0.417393944980506));
#40228=CARTESIAN_POINT('Ctrl Pts',(-0.0243301430172896,-0.606376229772182,
-0.406772732659772));
#40229=CARTESIAN_POINT('Ctrl Pts',(0.268924948789863,-0.54402523821012,
-0.396151520339041));
#40230=CARTESIAN_POINT('Ctrl Pts',(0.49654418722808,-0.348895339642708,
-0.385530308018308));
#40231=CARTESIAN_POINT('Ctrl Pts',(0.602973102433286,-0.0686114103358565,
-0.374909095697576));
#40232=CARTESIAN_POINT('Ctrl Pts',(0.562235849856194,0.22841833778935,-0.364287883376844));
#40233=CARTESIAN_POINT('Ctrl Pts',(0.384275070866584,0.469698581847689,
-0.353666671056111));
#40234=CARTESIAN_POINT('Ctrl Pts',(0.112525216897816,0.596340643809236,
-0.343045458735379));
#40235=CARTESIAN_POINT('Ctrl Pts',(-0.186688391221607,0.577435305907412,
-0.332424246414646));
#40236=CARTESIAN_POINT('Ctrl Pts',(-0.440337420784613,0.417596747609107,
-0.321803034093914));
#40237=CARTESIAN_POINT('Ctrl Pts',(-0.58651437550708,0.155836374298491,
-0.311181821773182));
#40238=CARTESIAN_POINT('Ctrl Pts',(-0.589542202382296,-0.14395860117576,
-0.30056060945245));
#40239=CARTESIAN_POINT('Ctrl Pts',(-0.44868191070889,-0.408617953378765,
-0.289939397131717));
#40240=CARTESIAN_POINT('Ctrl Pts',(-0.198312919647183,-0.573546923201999,
-0.279318184810985));
#40241=CARTESIAN_POINT('Ctrl Pts',(0.100457810451271,-0.598491699957539,
-0.268696972490252));
#40242=CARTESIAN_POINT('Ctrl Pts',(0.374710067503894,-0.477364075292773,
-0.25807576016952));
#40243=CARTESIAN_POINT('Ctrl Pts',(0.557507719479534,-0.239727367437853,
-0.247454547848788));
#40244=CARTESIAN_POINT('Ctrl Pts',(0.604235901607852,0.0564190059013063,
-0.236833335528056));
#40245=CARTESIAN_POINT('Ctrl Pts',(0.503489562133039,0.338795342097125,
-0.226212123207323));
#40246=CARTESIAN_POINT('Ctrl Pts',(0.279858047502047,0.538482706593586,
-0.215590910886591));
#40247=CARTESIAN_POINT('Ctrl Pts',(-0.0120783079673112,0.606743961071895,
-0.204969698565858));
#40248=CARTESIAN_POINT('Ctrl Pts',(-0.301065603751776,0.526918614476648,
-0.194348486245126));
#40249=CARTESIAN_POINT('Ctrl Pts',(-0.516574810615386,0.318489709300428,
-0.183727273924394));
#40250=CARTESIAN_POINT('Ctrl Pts',(-0.606000393860149,0.0323274504734039,
-0.173106061603662));
#40251=CARTESIAN_POINT('Ctrl Pts',(-0.54752982679742,-0.261724193796561,
-0.162484849282929));
#40252=CARTESIAN_POINT('Ctrl Pts',(-0.355407358238332,-0.491898842808179,
-0.151863636962197));
#40253=CARTESIAN_POINT('Ctrl Pts',(-0.076576683950909,-0.602014117802982,
-0.141242424641464));
#40254=CARTESIAN_POINT('Ctrl Pts',(0.221016091685922,-0.565203769676402,
-0.130621212320732));
#40255=CARTESIAN_POINT('Ctrl Pts',(0.383330620179427,-0.448679815853072,
-0.123540404106911));
#40256=CARTESIAN_POINT('Ctrl Pts',(0.44565123783516,-0.374523575106285,
-0.12));
#40257=CARTESIAN_POINT('Ctrl Pts',(-0.347393831483963,0.454739033234329,
-0.742528335043099));
#40258=CARTESIAN_POINT('Ctrl Pts',(-0.421311558764174,0.398270244285598,
-0.73906984429286));
#40259=CARTESIAN_POINT('Ctrl Pts',(-0.541032820871556,0.248672210016143,
-0.732152862792381));
#40260=CARTESIAN_POINT('Ctrl Pts',(-0.594466754531496,-0.0338563072418703,
-0.721777390541663));
#40261=CARTESIAN_POINT('Ctrl Pts',(-0.509318192700196,-0.308427575223672,
-0.711401918290944));
#40262=CARTESIAN_POINT('Ctrl Pts',(-0.305432606070274,-0.511127575150115,
-0.701026446040226));
#40263=CARTESIAN_POINT('Ctrl Pts',(-0.0303432431553614,-0.594654413195259,
-0.690650973789507));
#40264=CARTESIAN_POINT('Ctrl Pts',(0.251820278225985,-0.539559427088026,
-0.680275501538789));
#40265=CARTESIAN_POINT('Ctrl Pts',(0.47527762677182,-0.358674800641695,
-0.669900029288071));
#40266=CARTESIAN_POINT('Ctrl Pts',(0.587935213613219,-0.0941755582271385,
-0.659524557037353));
#40267=CARTESIAN_POINT('Ctrl Pts',(0.563529430095987,0.192279525622204,
-0.649149084786634));
#40268=CARTESIAN_POINT('Ctrl Pts',(0.407749978910367,0.433908628992312,
-0.638773612535916));
#40269=CARTESIAN_POINT('Ctrl Pts',(0.156913157834808,0.574382355007991,
-0.628398140285198));
#40270=CARTESIAN_POINT('Ctrl Pts',(-0.130504285744414,0.580952155897969,
-0.618022668034479));
#40271=CARTESIAN_POINT('Ctrl Pts',(-0.387497714117257,0.452086632150457,
-0.607647195783761));
#40272=CARTESIAN_POINT('Ctrl Pts',(-0.554155123557569,0.217827664148314,
-0.597271723533043));
#40273=CARTESIAN_POINT('Ctrl Pts',(-0.591624244031004,-0.0672127059237326,
-0.586896251282324));
#40274=CARTESIAN_POINT('Ctrl Pts',(-0.491170026481974,-0.336584016022301,
-0.576520779031606));
#40275=CARTESIAN_POINT('Ctrl Pts',(-0.276211019809465,-0.527488640774144,
-0.566145306780888));
#40276=CARTESIAN_POINT('Ctrl Pts',(0.0031401178304551,-0.595421643954287,
-0.555769834530169));
#40277=CARTESIAN_POINT('Ctrl Pts',(0.281759210488034,-0.524546033533648,
-0.545394362279452));
#40278=CARTESIAN_POINT('Ctrl Pts',(0.494692741566129,-0.331384799915253,
-0.535018890028733));
#40279=CARTESIAN_POINT('Ctrl Pts',(0.59230024480053,-0.0609689603923613,
-0.524643417778015));
#40280=CARTESIAN_POINT('Ctrl Pts',(0.551826816631903,0.223660364318458,
-0.514267945527296));
#40281=CARTESIAN_POINT('Ctrl Pts',(0.382707889009843,0.456148512904055,
-0.503892473276577));
#40282=CARTESIAN_POINT('Ctrl Pts',(0.124369579435742,0.582296317894835,
-0.49351700102586));
#40283=CARTESIAN_POINT('Ctrl Pts',(-0.162962585060135,0.572695372777406,
-0.483141528775141));
#40284=CARTESIAN_POINT('Ctrl Pts',(-0.412303839155969,0.429583913041453,
-0.472766056524423));
#40285=CARTESIAN_POINT('Ctrl Pts',(-0.565526108608774,0.186325024110395,
-0.462390584273704));
#40286=CARTESIAN_POINT('Ctrl Pts',(-0.586909209500827,-0.100371180778523,
-0.452015112022986));
#40287=CARTESIAN_POINT('Ctrl Pts',(-0.471468172615134,-0.363668195390408,
-0.441639639772268));
#40288=CARTESIAN_POINT('Ctrl Pts',(-0.24611537226857,-0.542184486739477,
-0.431264167521549));
#40289=CARTESIAN_POINT('Ctrl Pts',(0.0366134635183988,-0.594303162045059,
-0.420888695270832));
#40290=CARTESIAN_POINT('Ctrl Pts',(0.310806727710773,-0.507873972691536,
-0.410513223020113));
#40291=CARTESIAN_POINT('Ctrl Pts',(0.51254268190422,-0.30304586015049,-0.400137750769395));
#40292=CARTESIAN_POINT('Ctrl Pts',(0.594791312689474,-0.0275697021364228,
-0.389762278518676));
#40293=CARTESIAN_POINT('Ctrl Pts',(0.53837827792754,0.254333686297961,-0.379386806267958));
#40294=CARTESIAN_POINT('Ctrl Pts',(0.356454955565181,0.476945131829576,
-0.36901133401724));
#40295=CARTESIAN_POINT('Ctrl Pts',(0.0914325078965691,0.588367989131544,
-0.358635861766521));
#40296=CARTESIAN_POINT('Ctrl Pts',(-0.1949052878214,0.562626628325057,-0.348260389515803));
#40297=CARTESIAN_POINT('Ctrl Pts',(-0.435805479980445,0.405722044928676,
-0.337884917265085));
#40298=CARTESIAN_POINT('Ctrl Pts',(-0.575107830414381,0.154232867992362,
-0.327509445014366));
#40299=CARTESIAN_POINT('Ctrl Pts',(-0.580337258022503,-0.133212090073103,
-0.317133972763648));
#40300=CARTESIAN_POINT('Ctrl Pts',(-0.450274644860222,-0.389601769278859,
-0.30675850051293));
#40301=CARTESIAN_POINT('Ctrl Pts',(-0.215241042075345,-0.555164919115264,
-0.296383028262211));
#40302=CARTESIAN_POINT('Ctrl Pts',(0.0699709674208999,-0.591304370416951,
-0.286007556011493));
#40303=CARTESIAN_POINT('Ctrl Pts',(0.338870887774159,-0.489595052448449,
-0.275632083760774));
#40304=CARTESIAN_POINT('Ctrl Pts',(0.528770989858389,-0.273748118747132,
-0.265256611510057));
#40305=CARTESIAN_POINT('Ctrl Pts',(0.595400531599021,0.00591678855841044,
-0.254881139259338));
#40306=CARTESIAN_POINT('Ctrl Pts',(0.523226356835316,0.284202314475096,
-0.24450566700862));
#40307=CARTESIAN_POINT('Ctrl Pts',(0.329074261287382,0.496232767362635,
-0.234130194757902));
#40308=CARTESIAN_POINT('Ctrl Pts',(0.0582061064454895,0.592578090033583,
-0.223754722507183));
#40309=CARTESIAN_POINT('Ctrl Pts',(-0.226231237425986,0.550777869717469,
-0.213379250256465));
#40310=CARTESIAN_POINT('Ctrl Pts',(-0.457928466129024,0.380576366952199,
-0.203003778005746));
#40311=CARTESIAN_POINT('Ctrl Pts',(-0.582869603662733,0.121653032232085,
-0.192628305755028));
#40312=CARTESIAN_POINT('Ctrl Pts',(-0.57192991628486,-0.165632118696112,
-0.18225283350431));
#40313=CARTESIAN_POINT('Ctrl Pts',(-0.427655041590171,-0.414301519355521,
-0.171877361253592));
#40314=CARTESIAN_POINT('Ctrl Pts',(-0.183688600698895,-0.566391183638125,
-0.161501889002873));
#40315=CARTESIAN_POINT('Ctrl Pts',(0.103112831945545,-0.586430161623632,
-0.151126416752155));
#40316=CARTESIAN_POINT('Ctrl Pts',(0.365851355459577,-0.469776284513869,
-0.140750944501437));
#40317=CARTESIAN_POINT('Ctrl Pts',(0.543351022386391,-0.243565284402786,
-0.130375472250718));
#40318=CARTESIAN_POINT('Ctrl Pts',(0.577149518655877,-0.0549640805153465,
-0.123458490750239));
#40319=CARTESIAN_POINT('Ctrl Pts',(0.570996795169322,0.0378513197440182,
-0.12));
#40320=CARTESIAN_POINT('Ctrl Pts',(-0.347393831483963,0.454739033234329,
-0.739668503816594));
#40321=CARTESIAN_POINT('Ctrl Pts',(-0.421311232212742,0.398270493751654,
-0.736210013066354));
#40322=CARTESIAN_POINT('Ctrl Pts',(-0.541032978501356,0.24867202957397,
-0.729293031565875));
#40323=CARTESIAN_POINT('Ctrl Pts',(-0.594466633440188,-0.0338562272977153,
-0.718917559315157));
#40324=CARTESIAN_POINT('Ctrl Pts',(-0.509318208145951,-0.30842759690902,
-0.708542087064439));
#40325=CARTESIAN_POINT('Ctrl Pts',(-0.305432567022533,-0.511127527137462,
-0.698166614813721));
#40326=CARTESIAN_POINT('Ctrl Pts',(-0.0303432525733253,-0.594654389935448,
-0.687791142563002));
#40327=CARTESIAN_POINT('Ctrl Pts',(0.251820269803062,-0.53955939207586,
-0.677415670312284));
#40328=CARTESIAN_POINT('Ctrl Pts',(0.475277597483338,-0.358674783173242,
-0.667040198061565));
#40329=CARTESIAN_POINT('Ctrl Pts',(0.587935182297583,-0.0941755517205918,
-0.656664725810847));
#40330=CARTESIAN_POINT('Ctrl Pts',(0.563529397998721,0.192279514278788,
-0.64628925356013));
#40331=CARTESIAN_POINT('Ctrl Pts',(0.407749956566778,0.433908605151244,
-0.635913781309409));
#40332=CARTESIAN_POINT('Ctrl Pts',(0.156913148914841,0.574382322862107,
-0.625538309058693));
#40333=CARTESIAN_POINT('Ctrl Pts',(-0.130504278385431,0.580952123629563,
-0.615162836807973));
#40334=CARTESIAN_POINT('Ctrl Pts',(-0.387497692586036,0.452086606935182,
-0.604787364557256));
#40335=CARTESIAN_POINT('Ctrl Pts',(-0.554155092676422,0.217827652039444,
-0.594411892306537));
#40336=CARTESIAN_POINT('Ctrl Pts',(-0.591624211098557,-0.0672127021914847,
-0.584036420055819));
#40337=CARTESIAN_POINT('Ctrl Pts',(-0.491169999125539,-0.336583997274562,
-0.5736609478051));
#40338=CARTESIAN_POINT('Ctrl Pts',(-0.276211004431821,-0.527488611403925,
-0.563285475554383));
#40339=CARTESIAN_POINT('Ctrl Pts',(0.00314011765710889,-0.595421610797266,
-0.552910003303663));
#40340=CARTESIAN_POINT('Ctrl Pts',(0.281759194797687,-0.524546004325305,
-0.542534531052945));
#40341=CARTESIAN_POINT('Ctrl Pts',(0.494692714019857,-0.331384781461957,
-0.532159058802227));
#40342=CARTESIAN_POINT('Ctrl Pts',(0.592300211818467,-0.060968956997514,
-0.521783586551509));
#40343=CARTESIAN_POINT('Ctrl Pts',(0.551826785903869,0.223660351864156,
-0.51140811430079));
#40344=CARTESIAN_POINT('Ctrl Pts',(0.382707867698945,0.456148487503667,
-0.501032642050072));
#40345=CARTESIAN_POINT('Ctrl Pts',(0.124369572510325,0.58229628547005,-0.490657169799354));
#40346=CARTESIAN_POINT('Ctrl Pts',(-0.162962575985677,0.572695340887211,
-0.480281697548635));
#40347=CARTESIAN_POINT('Ctrl Pts',(-0.412303816197081,0.429583889120347,
-0.469906225297917));
#40348=CARTESIAN_POINT('Ctrl Pts',(-0.565526077117809,0.186325013734999,
-0.459530753047199));
#40349=CARTESIAN_POINT('Ctrl Pts',(-0.586909176819153,-0.100371175189415,
-0.44915528079648));
#40350=CARTESIAN_POINT('Ctrl Pts',(-0.471468146361724,-0.363668175139773,
-0.438779808545763));
#40351=CARTESIAN_POINT('Ctrl Pts',(-0.246115358563789,-0.542184456548272,
-0.428404336295043));
#40352=CARTESIAN_POINT('Ctrl Pts',(0.0366134614796009,-0.59430312895166,
-0.418028864044326));
#40353=CARTESIAN_POINT('Ctrl Pts',(0.310806710403695,-0.507873944410889,
-0.407653391793607));
#40354=CARTESIAN_POINT('Ctrl Pts',(0.5125426533636,-0.303045843275575,-0.397277919542889));
#40355=CARTESIAN_POINT('Ctrl Pts',(0.594791279568892,-0.0275697006012128,
-0.386902447292171));
#40356=CARTESIAN_POINT('Ctrl Pts',(0.538378247948281,0.254333672135533,
-0.376526975041452));
#40357=CARTESIAN_POINT('Ctrl Pts',(0.356454935716209,0.476945105271217,
-0.366151502790734));
#40358=CARTESIAN_POINT('Ctrl Pts',(0.0914325028052065,0.588367956368575,
-0.355776030540016));
#40359=CARTESIAN_POINT('Ctrl Pts',(-0.19490527696822,0.562626596995675,
-0.345400558289297));
#40360=CARTESIAN_POINT('Ctrl Pts',(-0.435805455712891,0.405722022336039,
-0.335025086038579));
#40361=CARTESIAN_POINT('Ctrl Pts',(-0.575107798389857,0.154232859404514,
-0.324649613787861));
#40362=CARTESIAN_POINT('Ctrl Pts',(-0.580337225706793,-0.133212082656289,
-0.314274141537142));
#40363=CARTESIAN_POINT('Ctrl Pts',(-0.450274619786945,-0.389601747582111,
-0.303898669286424));
#40364=CARTESIAN_POINT('Ctrl Pts',(-0.215241030089811,-0.555164888205254,
-0.293523197035706));
#40365=CARTESIAN_POINT('Ctrl Pts',(0.069970963524667,-0.591304337482598,
-0.283147724784988));
#40366=CARTESIAN_POINT('Ctrl Pts',(0.338870868904234,-0.489595025201401,
-0.272772252534269));
#40367=CARTESIAN_POINT('Ctrl Pts',(0.528770960414329,-0.273748103472406,
-0.262396780283551));
#40368=CARTESIAN_POINT('Ctrl Pts',(0.595400498444076,0.00591678816698449,
-0.252021308032832));
#40369=CARTESIAN_POINT('Ctrl Pts',(0.523226327700652,0.284202298772356,
-0.241645835782114));
#40370=CARTESIAN_POINT('Ctrl Pts',(0.329074242961365,0.496232739486468,
-0.231270363531395));
#40371=CARTESIAN_POINT('Ctrl Pts',(0.0582061032077348,0.592578057519749,
-0.220894891280678));
#40372=CARTESIAN_POINT('Ctrl Pts',(-0.226231224835217,0.550777838088684,
-0.210519419029959));
#40373=CARTESIAN_POINT('Ctrl Pts',(-0.457928440616124,0.380576347662404,
-0.200143946779241));
#40374=CARTESIAN_POINT('Ctrl Pts',(-0.582869571232661,0.121653021684456,
-0.189768474528522));
#40375=CARTESIAN_POINT('Ctrl Pts',(-0.571929884384423,-0.165632101988046,
-0.179393002277804));
#40376=CARTESIAN_POINT('Ctrl Pts',(-0.427655017881361,-0.414301511133043,
-0.169017530027086));
#40377=CARTESIAN_POINT('Ctrl Pts',(-0.18368859026215,-0.566391122638,-0.158642057776367));
#40378=CARTESIAN_POINT('Ctrl Pts',(0.103112825789684,-0.586430187525968,
-0.148266585525649));
#40379=CARTESIAN_POINT('Ctrl Pts',(0.365851335923764,-0.469776140734439,
-0.137891113274931));
#40380=CARTESIAN_POINT('Ctrl Pts',(0.543350990324924,-0.243565521844555,
-0.127515641024213));
#40381=CARTESIAN_POINT('Ctrl Pts',(0.577149491474567,-0.0549636704783635,
-0.120598659523734));
#40382=CARTESIAN_POINT('Ctrl Pts',(0.570996795169322,0.0378513197440182,
-0.117140168773494));
#40383=CARTESIAN_POINT('Ctrl Pts',(-0.348354931983335,0.455997115192948,
-0.732991220638421));
#40384=CARTESIAN_POINT('Ctrl Pts',(-0.422477789664249,0.399371618702867,
-0.729532729888182));
#40385=CARTESIAN_POINT('Ctrl Pts',(-0.542529339555234,0.249360534892675,
-0.722615748387703));
#40386=CARTESIAN_POINT('Ctrl Pts',(-0.596111640911723,-0.0339501282728968,
-0.712240276136984));
#40387=CARTESIAN_POINT('Ctrl Pts',(-0.510727243702018,-0.309280829796352,
-0.701864803886266));
#40388=CARTESIAN_POINT('Ctrl Pts',(-0.306277691824433,-0.512541754315929,
-0.691489331635547));
#40389=CARTESIAN_POINT('Ctrl Pts',(-0.0304271726811044,-0.596299630171875,
-0.68111385938483));
#40390=CARTESIAN_POINT('Ctrl Pts',(0.25251698096947,-0.541052240814961,
-0.67073838713411));
#40391=CARTESIAN_POINT('Ctrl Pts',(0.476592587302813,-0.359667144766162,
-0.660362914883394));
#40392=CARTESIAN_POINT('Ctrl Pts',(0.589561856766694,-0.0944361170651719,
-0.649987442632673));
#40393=CARTESIAN_POINT('Ctrl Pts',(0.565088553664507,0.192811508424799,
-0.639611970381957));
#40394=CARTESIAN_POINT('Ctrl Pts',(0.408878103922812,0.435109127467229,
-0.629236498131237));
#40395=CARTESIAN_POINT('Ctrl Pts',(0.157347291299003,0.575971504394943,
-0.61886102588052));
#40396=CARTESIAN_POINT('Ctrl Pts',(-0.130865353358995,0.582559481545958,
-0.608485553629801));
#40397=CARTESIAN_POINT('Ctrl Pts',(-0.388569807605722,0.453337424575784,
-0.598110081379083));
#40398=CARTESIAN_POINT('Ctrl Pts',(-0.555688309805857,0.218430329959781,
-0.587734609128365));
#40399=CARTESIAN_POINT('Ctrl Pts',(-0.593261096380303,-0.0673986639305479,
-0.577359136877646));
#40400=CARTESIAN_POINT('Ctrl Pts',(-0.492528951234956,-0.337515246201882,
-0.566983664626928));
#40401=CARTESIAN_POINT('Ctrl Pts',(-0.276975215435484,-0.528948048563023,
-0.55660819237621));
#40402=CARTESIAN_POINT('Ctrl Pts',(0.00314880562114232,-0.597069002631033,
-0.546232720125491));
#40403=CARTESIAN_POINT('Ctrl Pts',(0.282538756352733,-0.525997299987159,
-0.535857247874774));
#40404=CARTESIAN_POINT('Ctrl Pts',(0.496061412635949,-0.33230164536513,
-0.525481775624054));
#40405=CARTESIAN_POINT('Ctrl Pts',(0.59393896747061,-0.0611376437893791,
-0.515106303373337));
#40406=CARTESIAN_POINT('Ctrl Pts',(0.553353561086247,0.224279167556245,
-0.504730831122618));
#40407=CARTESIAN_POINT('Ctrl Pts',(0.383766730533475,0.457410543293981,
-0.4943553588719));
#40408=CARTESIAN_POINT('Ctrl Pts',(0.1247136739233,0.583907362605643,-0.483979886621181));
#40409=CARTESIAN_POINT('Ctrl Pts',(-0.163413455180115,0.574279854462932,
-0.473604414370463));
#40410=CARTESIAN_POINT('Ctrl Pts',(-0.413444564073729,0.430772446902474,
-0.463228942119745));
#40411=CARTESIAN_POINT('Ctrl Pts',(-0.567090755023527,0.186840531310716,
-0.452853469869027));
#40412=CARTESIAN_POINT('Ctrl Pts',(-0.588533016742363,-0.100648878670382,
-0.442477997618308));
#40413=CARTESIAN_POINT('Ctrl Pts',(-0.472772588051884,-0.364674359614158,
-0.43210252536759));
#40414=CARTESIAN_POINT('Ctrl Pts',(-0.246796301988659,-0.543684553669019,
-0.421727053116871));
#40415=CARTESIAN_POINT('Ctrl Pts',(0.0367147623329972,-0.595947426204782,
-0.411351580866153));
#40416=CARTESIAN_POINT('Ctrl Pts',(0.311666639613677,-0.509279112398487,
-0.400976108615435));
#40417=CARTESIAN_POINT('Ctrl Pts',(0.513960738572949,-0.303884299987962,
-0.390600636364716));
#40418=CARTESIAN_POINT('Ctrl Pts',(0.596436927420187,-0.0276459794911836,
-0.380225164113998));
#40419=CARTESIAN_POINT('Ctrl Pts',(0.539867814183286,0.255037353704964,
-0.36984969186328));
#40420=CARTESIAN_POINT('Ctrl Pts',(0.357441162850323,0.478264700420943,
-0.359474219612561));
#40421=CARTESIAN_POINT('Ctrl Pts',(0.0916854750779169,0.589995832392556,
-0.349098747361843));
#40422=CARTESIAN_POINT('Ctrl Pts',(-0.195444534118195,0.564183252720138,
-0.338723275111125));
#40423=CARTESIAN_POINT('Ctrl Pts',(-0.437011227109361,0.4068445599348,-0.328347802860406));
#40424=CARTESIAN_POINT('Ctrl Pts',(-0.576698986669175,0.15465958552089,
-0.317972330609689));
#40425=CARTESIAN_POINT('Ctrl Pts',(-0.581942882583927,-0.13358064921627,
-0.30759685835897));
#40426=CARTESIAN_POINT('Ctrl Pts',(-0.451520423964013,-0.3906796841698,
-0.297221386108251));
#40427=CARTESIAN_POINT('Ctrl Pts',(-0.215836551495043,-0.556700899121684,
-0.286845913857534));
#40428=CARTESIAN_POINT('Ctrl Pts',(0.0701645567558304,-0.592940337806916,
-0.276470441606815));
#40429=CARTESIAN_POINT('Ctrl Pts',(0.339808445053429,-0.49094961966413,
-0.266094969356097));
#40430=CARTESIAN_POINT('Ctrl Pts',(0.530233945539261,-0.274505500307545,
-0.255719497105378));
#40431=CARTESIAN_POINT('Ctrl Pts',(0.597047831862276,0.00593315871250194,
-0.24534402485466));
#40432=CARTESIAN_POINT('Ctrl Pts',(0.524673972126497,0.284988619460275,
-0.234968552603942));
#40433=CARTESIAN_POINT('Ctrl Pts',(0.329984714150923,0.497605699706947,
-0.224593080353223));
#40434=CARTESIAN_POINT('Ctrl Pts',(0.0583671458221994,0.594217580488307,
-0.214217608102505));
#40435=CARTESIAN_POINT('Ctrl Pts',(-0.226857153509737,0.552301713889382,
-0.203842135851787));
#40436=CARTESIAN_POINT('Ctrl Pts',(-0.459195421158135,0.381629307506569,
-0.193466663601068));
#40437=CARTESIAN_POINT('Ctrl Pts',(-0.584482234437336,0.12198961809667,
-0.18309119135035));
#40438=CARTESIAN_POINT('Ctrl Pts',(-0.5735122802766,-0.166090389068003,
-0.172715719099632));
#40439=CARTESIAN_POINT('Ctrl Pts',(-0.428838238622185,-0.415447742653517,
-0.162340246848914));
#40440=CARTESIAN_POINT('Ctrl Pts',(-0.184196814082961,-0.567958280253259,
-0.151964774598195));
#40441=CARTESIAN_POINT('Ctrl Pts',(0.103398115987721,-0.588052530603492,
-0.141589302347477));
#40442=CARTESIAN_POINT('Ctrl Pts',(0.366863558240637,-0.471076245713187,
-0.131213830096758));
#40443=CARTESIAN_POINT('Ctrl Pts',(0.544854320261013,-0.244238674933168,
-0.12083835784604));
#40444=CARTESIAN_POINT('Ctrl Pts',(0.57874631411382,-0.0551169346444906,
-0.113921376345561));
#40445=CARTESIAN_POINT('Ctrl Pts',(0.572576516094799,0.037956039284237,
-0.110462885595322));
#40446=CARTESIAN_POINT('Ctrl Pts',(-0.351337134117122,0.45990082214547,
-0.728010697470567));
#40447=CARTESIAN_POINT('Ctrl Pts',(-0.426092626832245,0.402792029759496,
-0.724552206720328));
#40448=CARTESIAN_POINT('Ctrl Pts',(-0.547174758248607,0.251494205008789,
-0.717635225219848));
#40449=CARTESIAN_POINT('Ctrl Pts',(-0.601214131526913,-0.0342402997241306,
-0.707259752969131));
#40450=CARTESIAN_POINT('Ctrl Pts',(-0.515099575835888,-0.31192865307436,
-0.696884280718412));
#40451=CARTESIAN_POINT('Ctrl Pts',(-0.308899449256672,-0.516929247603259,
-0.686508808467694));
#40452=CARTESIAN_POINT('Ctrl Pts',(-0.0306877093666915,-0.601404304453816,
-0.676133336216976));
#40453=CARTESIAN_POINT('Ctrl Pts',(0.254678682685534,-0.545683883423435,
-0.665757863966257));
#40454=CARTESIAN_POINT('Ctrl Pts',(0.480672436342572,-0.362746086111476,
-0.655382391715539));
#40455=CARTESIAN_POINT('Ctrl Pts',(0.594608802924677,-0.0952445289974541,
-0.64500691946482));
#40456=CARTESIAN_POINT('Ctrl Pts',(0.569925983813122,0.194462065489843,
-0.634631447214103));
#40457=CARTESIAN_POINT('Ctrl Pts',(0.412378302566623,0.438833876260333,
-0.624255974963383));
#40458=CARTESIAN_POINT('Ctrl Pts',(0.158694259988426,0.580902101186212,
-0.613880502712666));
#40459=CARTESIAN_POINT('Ctrl Pts',(-0.131985624240206,0.587546476071686,
-0.603505030461946));
#40460=CARTESIAN_POINT('Ctrl Pts',(-0.391896155450462,0.457218214381192,
-0.59312955821123));
#40461=CARTESIAN_POINT('Ctrl Pts',(-0.560445273344952,0.220300200523357,
-0.58275408596051));
#40462=CARTESIAN_POINT('Ctrl Pts',(-0.598339701552755,-0.0679756295146297,
-0.572378613709792));
#40463=CARTESIAN_POINT('Ctrl Pts',(-0.496745239880617,-0.340404541731139,
-0.562003141459074));
#40464=CARTESIAN_POINT('Ctrl Pts',(-0.279346258744421,-0.533476102542041,
-0.551627669208356));
#40465=CARTESIAN_POINT('Ctrl Pts',(0.00317576094595877,-0.60218020526613,
-0.541252196957638));
#40466=CARTESIAN_POINT('Ctrl Pts',(0.284957426270576,-0.530500094103756,
-0.530876724706919));
#40467=CARTESIAN_POINT('Ctrl Pts',(0.500307940915774,-0.335146309950583,
-0.520501252456201));
#40468=CARTESIAN_POINT('Ctrl Pts',(0.599023375480799,-0.0616610119189332,
-0.510125780205482));
#40469=CARTESIAN_POINT('Ctrl Pts',(0.5580905381723,0.226199106908691,-0.499750307954764));
#40470=CARTESIAN_POINT('Ctrl Pts',(0.387051961417286,0.461326201228568,
-0.489374835704046));
#40471=CARTESIAN_POINT('Ctrl Pts',(0.125781283960076,0.588905895173768,
-0.478999363453328));
#40472=CARTESIAN_POINT('Ctrl Pts',(-0.164812354269457,0.579195970853089,
-0.468623891202609));
#40473=CARTESIAN_POINT('Ctrl Pts',(-0.416983851726037,0.434460069705598,
-0.458248418951891));
#40474=CARTESIAN_POINT('Ctrl Pts',(-0.571945329206932,0.188439977628023,
-0.447872946701173));
#40475=CARTESIAN_POINT('Ctrl Pts',(-0.593571147171812,-0.101510482291401,
-0.437497474450454));
#40476=CARTESIAN_POINT('Ctrl Pts',(-0.476819752602251,-0.367796150466586,
-0.427122002199736));
#40477=CARTESIAN_POINT('Ctrl Pts',(-0.248908999022731,-0.548338759322636,
-0.416746529949018));
#40478=CARTESIAN_POINT('Ctrl Pts',(0.037029058652927,-0.601049027605061,
-0.406371057698299));
#40479=CARTESIAN_POINT('Ctrl Pts',(0.314334658460906,-0.513638790649771,
-0.395995585447581));
#40480=CARTESIAN_POINT('Ctrl Pts',(0.518360493833721,-0.306485698202276,
-0.385620113196863));
#40481=CARTESIAN_POINT('Ctrl Pts',(0.601542719190241,-0.0278826425950967,
-0.375244640946144));
#40482=CARTESIAN_POINT('Ctrl Pts',(0.544489346680437,0.257220598171695,
-0.364869168695426));
#40483=CARTESIAN_POINT('Ctrl Pts',(0.36050103400125,0.482358880139147,-0.354493696444707));
#40484=CARTESIAN_POINT('Ctrl Pts',(0.092470347580881,0.595046485238944,
-0.34411822419399));
#40485=CARTESIAN_POINT('Ctrl Pts',(-0.197117634907101,0.569012937262736,
-0.33374275194327));
#40486=CARTESIAN_POINT('Ctrl Pts',(-0.44075225692194,0.410327348322645,
-0.323367279692553));
#40487=CARTESIAN_POINT('Ctrl Pts',(-0.581635812014072,0.155983547208043,
-0.312991807441834));
#40488=CARTESIAN_POINT('Ctrl Pts',(-0.586924598242304,-0.134724164903533,
-0.302616335191116));
#40489=CARTESIAN_POINT('Ctrl Pts',(-0.455385659596904,-0.394024093305776,
-0.292240862940398));
#40490=CARTESIAN_POINT('Ctrl Pts',(-0.217684217925031,-0.561466531081166,
-0.281865390689679));
#40491=CARTESIAN_POINT('Ctrl Pts',(0.0707651996740672,-0.598016197013366,
-0.271489918438961));
#40492=CARTESIAN_POINT('Ctrl Pts',(0.342717371516556,-0.495152388586516,
-0.261114446188242));
#40493=CARTESIAN_POINT('Ctrl Pts',(0.534773007410933,-0.276855401446306,
-0.250738973937525));
#40494=CARTESIAN_POINT('Ctrl Pts',(0.602158853270531,0.00598394908883089,
-0.240363501686806));
#40495=CARTESIAN_POINT('Ctrl Pts',(0.529165437910601,0.287428262130249,
-0.229988029436088));
#40496=CARTESIAN_POINT('Ctrl Pts',(0.332809544664039,0.501865446406052,
-0.219612557185369));
#40497=CARTESIAN_POINT('Ctrl Pts',(0.0588667971533626,0.599304376401761,
-0.209237084934651));
#40498=CARTESIAN_POINT('Ctrl Pts',(-0.228799161721906,0.557029681018242,
-0.198861612683933));
#40499=CARTESIAN_POINT('Ctrl Pts',(-0.463126358441445,0.384896252172232,
-0.188486140433214));
#40500=CARTESIAN_POINT('Ctrl Pts',(-0.589485688345832,0.12303388673101,
-0.178110668182496));
#40501=CARTESIAN_POINT('Ctrl Pts',(-0.578421825546005,-0.167512160079637,
-0.167735195931778));
#40502=CARTESIAN_POINT('Ctrl Pts',(-0.432509304272308,-0.419004265658045,
-0.157359723681059));
#40503=CARTESIAN_POINT('Ctrl Pts',(-0.18577362766596,-0.572820107924446,
-0.146984251430341));
#40504=CARTESIAN_POINT('Ctrl Pts',(0.104283251993704,-0.593086891600813,
-0.136608779179623));
#40505=CARTESIAN_POINT('Ctrl Pts',(0.370004094613953,-0.47510819824727,
-0.126233306928905));
#40506=CARTESIAN_POINT('Ctrl Pts',(0.549518529090563,-0.246330950965504,
-0.115857834678186));
#40507=CARTESIAN_POINT('Ctrl Pts',(0.583700694682622,-0.0555863733805506,
-0.108940853177707));
#40508=CARTESIAN_POINT('Ctrl Pts',(0.577478237733509,0.0382809739154165,
-0.105482362427468));
#40509=CARTESIAN_POINT('Ctrl Pts',(-0.353390396098499,0.46258854508056,
-0.72625));
#40510=CARTESIAN_POINT('Ctrl Pts',(-0.42858405975876,0.405145015906336,
-0.722791509249761));
#40511=CARTESIAN_POINT('Ctrl Pts',(-0.55037189938968,0.252964683975255,
-0.715874527749282));
#40512=CARTESIAN_POINT('Ctrl Pts',(-0.604728186893475,-0.0344407204224906,
-0.705499055498564));
#40513=CARTESIAN_POINT('Ctrl Pts',(-0.518109826791218,-0.313751520890275,
-0.695123583247845));
#40514=CARTESIAN_POINT('Ctrl Pts',(-0.310704853852748,-0.519950442031676,
-0.684748110997127));
#40515=CARTESIAN_POINT('Ctrl Pts',(-0.0308670153174011,-0.604919084841303,
-0.674372638746408));
#40516=CARTESIAN_POINT('Ctrl Pts',(0.256167092800043,-0.548873072509114,
-0.663997166495691));
#40517=CARTESIAN_POINT('Ctrl Pts',(0.483481667087119,-0.364866092549401,
-0.653621694244972));
#40518=CARTESIAN_POINT('Ctrl Pts',(0.598083901292941,-0.0958011766717911,
-0.643246221994253));
#40519=CARTESIAN_POINT('Ctrl Pts',(0.573256835517459,0.19559857304029,-0.632870749743536));
#40520=CARTESIAN_POINT('Ctrl Pts',(0.414788385679614,0.441398575257167,
-0.622495277492817));
#40521=CARTESIAN_POINT('Ctrl Pts',(0.159621726049182,0.584297099004858,
-0.612119805242099));
#40522=CARTESIAN_POINT('Ctrl Pts',(-0.132756995237261,0.59098030500446,
-0.601744332991381));
#40523=CARTESIAN_POINT('Ctrl Pts',(-0.394186534902482,0.459890359376923,
-0.591368860740661));
#40524=CARTESIAN_POINT('Ctrl Pts',(-0.563720713685333,0.221587712671107,
-0.580993388489944));
#40525=CARTESIAN_POINT('Ctrl Pts',(-0.601836610185299,-0.068372903075961,
-0.570617916239225));
#40526=CARTESIAN_POINT('Ctrl Pts',(-0.499648394643955,-0.342393986198443,
-0.560242443988507));
#40527=CARTESIAN_POINT('Ctrl Pts',(-0.280978856994308,-0.536593925414127,
-0.549866971737789));
#40528=CARTESIAN_POINT('Ctrl Pts',(0.00319432120933226,-0.605699559211484,
-0.539491499487071));
#40529=CARTESIAN_POINT('Ctrl Pts',(0.286622818181397,-0.53360052413858,
-0.529116027236352));
#40530=CARTESIAN_POINT('Ctrl Pts',(0.503231917338109,-0.337105023433553,
-0.518740554985634));
#40531=CARTESIAN_POINT('Ctrl Pts',(0.602524279792687,-0.0620213806639361,
-0.508365082734915));
#40532=CARTESIAN_POINT('Ctrl Pts',(0.561352216515463,0.227521094431647,
-0.497989610484197));
#40533=CARTESIAN_POINT('Ctrl Pts',(0.389314029870597,0.464022354589065,
-0.487614138233479));
#40534=CARTESIAN_POINT('Ctrl Pts',(0.126516394236637,0.592347669354205,
-0.477238665982761));
#40535=CARTESIAN_POINT('Ctrl Pts',(-0.165775575915184,0.582580996804279,
-0.466863193732042));
#40536=CARTESIAN_POINT('Ctrl Pts',(-0.41942085272457,0.436999207898342,
-0.456487721481324));
#40537=CARTESIAN_POINT('Ctrl Pts',(-0.575287979845788,0.189541287455112,
-0.446112249230606));
#40538=CARTESIAN_POINT('Ctrl Pts',(-0.597040186733796,-0.10210374542541,
-0.435736776979887));
#40539=CARTESIAN_POINT('Ctrl Pts',(-0.479606455752478,-0.369945681155179,
-0.425361304729169));
#40540=CARTESIAN_POINT('Ctrl Pts',(-0.250363711181598,-0.55154344482415,
-0.41498583247845));
#40541=CARTESIAN_POINT('Ctrl Pts',(0.03724546955838,-0.604561770543093,
-0.404610360227732));
#40542=CARTESIAN_POINT('Ctrl Pts',(0.316171741296042,-0.51664067727082,
-0.394234887977014));
#40543=CARTESIAN_POINT('Ctrl Pts',(0.521389975756897,-0.308276908939691,
-0.383859415726296));
#40544=CARTESIAN_POINT('Ctrl Pts',(0.605058347436381,-0.0280455986126449,
-0.373483943475577));
#40545=CARTESIAN_POINT('Ctrl Pts',(0.54767153485402,0.25872388625351,-0.363108471224859));
#40546=CARTESIAN_POINT('Ctrl Pts',(0.362607929451007,0.485177955908193,
-0.35273299897414));
#40547=CARTESIAN_POINT('Ctrl Pts',(0.0930107769727027,0.598524147198255,
-0.342357526723423));
#40548=CARTESIAN_POINT('Ctrl Pts',(-0.198269660030149,0.572338449966212,
-0.331982054472703));
#40549=CARTESIAN_POINT('Ctrl Pts',(-0.443328168880556,0.412725446363766,
-0.321606582221986));
#40550=CARTESIAN_POINT('Ctrl Pts',(-0.585035097259257,0.156895170183079,
-0.311231109971267));
#40551=CARTESIAN_POINT('Ctrl Pts',(-0.59035479302331,-0.13551154053297,
-0.300855637720549));
#40552=CARTESIAN_POINT('Ctrl Pts',(-0.458047094332503,-0.396326909369684,
-0.29048016546983));
#40553=CARTESIAN_POINT('Ctrl Pts',(-0.218956441427693,-0.564747939904601,
-0.280104693219113));
#40554=CARTESIAN_POINT('Ctrl Pts',(0.0711787765103383,-0.601511215048924,
-0.269729220968394));
#40555=CARTESIAN_POINT('Ctrl Pts',(0.344720332958152,-0.49804623407831,
-0.259353748717676));
#40556=CARTESIAN_POINT('Ctrl Pts',(0.537898409863037,-0.27847344238101,
-0.248978276466957));
#40557=CARTESIAN_POINT('Ctrl Pts',(0.605678082423716,0.00601892164681181,
-0.238602804216239));
#40558=CARTESIAN_POINT('Ctrl Pts',(0.532258067742181,0.289108093990727,
-0.228227331965521));
#40559=CARTESIAN_POINT('Ctrl Pts',(0.334754601270279,0.504798526405128,
-0.217851859714803));
#40560=CARTESIAN_POINT('Ctrl Pts',(0.0592108355069413,0.602806921072019,
-0.207476387464084));
#40561=CARTESIAN_POINT('Ctrl Pts',(-0.230136344857676,0.560285163125383,
-0.197100915213366));
#40562=CARTESIAN_POINT('Ctrl Pts',(-0.465833032609804,0.387145714385472,
-0.186725442962647));
#40563=CARTESIAN_POINT('Ctrl Pts',(-0.592930850937281,0.123752955150168,
-0.176349970711929));
#40564=CARTESIAN_POINT('Ctrl Pts',(-0.581802327327214,-0.168491189905756,
-0.165974498461211));
#40565=CARTESIAN_POINT('Ctrl Pts',(-0.435037041088184,-0.421453016030356,
-0.155599026210493));
#40566=CARTESIAN_POINT('Ctrl Pts',(-0.186859355223635,-0.576167987432484,
-0.145223553959774));
#40567=CARTESIAN_POINT('Ctrl Pts',(0.104892721809184,-0.596552869735825,
-0.134848081709056));
#40568=CARTESIAN_POINT('Ctrl Pts',(0.372166526005229,-0.477885362998166,
-0.124472609458337));
#40569=CARTESIAN_POINT('Ctrl Pts',(0.552730116713414,-0.247769604783317,
-0.114097137207619));
#40570=CARTESIAN_POINT('Ctrl Pts',(0.587112028255095,-0.055912847103633,
-0.10718015570714));
#40571=CARTESIAN_POINT('Ctrl Pts',(0.580853099071723,0.0385046931318555,
-0.103721664956901));
#40572=CARTESIAN_POINT('Ctrl Pts',(0.445651237835157,-0.374523575106288,
-0.12));
#40573=CARTESIAN_POINT('Ctrl Pts',(0.471006333574204,-0.339660302329497,
-0.12));
#40574=CARTESIAN_POINT('Ctrl Pts',(0.506496757742905,-0.286240975539979,
-0.12));
#40575=CARTESIAN_POINT('Ctrl Pts',(0.548090602650708,-0.175383051808221,
-0.12));
#40576=CARTESIAN_POINT('Ctrl Pts',(0.558638194972283,-0.135500469697039,
-0.12));
#40577=CARTESIAN_POINT('Ctrl Pts',(0.571925545859982,-0.0509094028730825,
-0.12));
#40578=CARTESIAN_POINT('Ctrl Pts',(0.573933770267675,-0.00645369735957208,
-0.12));
#40579=CARTESIAN_POINT('Ctrl Pts',(0.570996795169322,0.0378513197440184,
-0.12));
#40580=CARTESIAN_POINT('',(-0.565495273463993,0.0874028629208282,-0.72625));
#40581=CARTESIAN_POINT('Ctrl Pts',(-0.565534825602702,0.0874095162469272,
-0.72625));
#40582=CARTESIAN_POINT('Ctrl Pts',(-0.558753848852679,0.131282067753869,
-0.72625));
#40583=CARTESIAN_POINT('Ctrl Pts',(-0.547115463002498,0.17422512350475,
-0.72625));
#40584=CARTESIAN_POINT('Ctrl Pts',(-0.515734564221166,0.253877204522193,
-0.72625));
#40585=CARTESIAN_POINT('Ctrl Pts',(-0.496760829533906,0.290498979877212,
-0.72625));
#40586=CARTESIAN_POINT('Ctrl Pts',(-0.432021967366878,0.389656916743186,
-0.72625));
#40587=CARTESIAN_POINT('Ctrl Pts',(-0.385735474250614,0.434078643348275,
-0.72625));
#40588=CARTESIAN_POINT('Ctrl Pts',(-0.353390396098499,0.46258854508056,
-0.72625));
#40589=CARTESIAN_POINT('Ctrl Pts',(-0.565495271712367,0.0874028626261757,
-0.726250000000001));
#40590=CARTESIAN_POINT('Ctrl Pts',(-0.56997393358064,0.05848913808605,-0.725162434688994));
#40591=CARTESIAN_POINT('Ctrl Pts',(-0.572256945759171,0.0292370242315025,
-0.724074869377987));
#40592=CARTESIAN_POINT('Ctrl Pts',(-0.57227986394681,-1.09618492728156E-5,
-0.722987304066981));
#40593=CARTESIAN_POINT('Origin',(-1.17892742873597E-16,0.,-0.72625));
#40594=CARTESIAN_POINT('',(-0.6516,-7.97979854324415E-17,-0.72625));
#40595=CARTESIAN_POINT('Origin',(0.,0.,-0.72625));
#40596=CARTESIAN_POINT('Origin',(0.,0.,-0.72625));
#40597=CARTESIAN_POINT('',(0.462889160393653,-0.444455658495748,-0.72625));
#40598=CARTESIAN_POINT('Ctrl Pts',(0.6516,-1.66533453693773E-16,-0.72625));
#40599=CARTESIAN_POINT('Ctrl Pts',(0.6516,-0.0505003751377495,-0.72625));
#40600=CARTESIAN_POINT('Ctrl Pts',(0.645506923582183,-0.100849053895293,
-0.72625));
#40601=CARTESIAN_POINT('Ctrl Pts',(0.622270462633308,-0.195195237486754,
-0.72625));
#40602=CARTESIAN_POINT('Ctrl Pts',(0.606052107869727,-0.239165633749014,
-0.72625));
#40603=CARTESIAN_POINT('Ctrl Pts',(0.546829171420724,-0.35650676310561,
-0.72625));
#40604=CARTESIAN_POINT('Ctrl Pts',(0.499772339104853,-0.410635277409444,
-0.72625));
#40605=CARTESIAN_POINT('Ctrl Pts',(0.462889160393654,-0.444455658495747,
-0.72625));
#40606=CARTESIAN_POINT('',(-0.353390396098496,-0.462588545080562,-0.72625));
#40607=CARTESIAN_POINT('Ctrl Pts',(0.462926795561194,-0.444481916564912,
-0.72625));
#40608=CARTESIAN_POINT('Ctrl Pts',(0.439708289239495,-0.465744192282609,
-0.72625));
#40609=CARTESIAN_POINT('Ctrl Pts',(0.414979050320746,-0.485210232281103,
-0.72625));
#40610=CARTESIAN_POINT('Ctrl Pts',(0.388971950023878,-0.502761089181296,
-0.72625));
#40611=CARTESIAN_POINT('Ctrl Pts',(0.361777826790807,-0.521113006924594,
-0.72625));
#40612=CARTESIAN_POINT('Ctrl Pts',(0.333185315488392,-0.537372018715419,
-0.72625));
#40613=CARTESIAN_POINT('Ctrl Pts',(0.303435179814313,-0.551346893096332,
-0.72625));
#40614=CARTESIAN_POINT('Ctrl Pts',(0.296196613580324,-0.554747148306128,
-0.72625));
#40615=CARTESIAN_POINT('Ctrl Pts',(0.288889451743085,-0.558011890011791,
-0.72625));
#40616=CARTESIAN_POINT('Ctrl Pts',(0.281517080262701,-0.56113778168721,
-0.72625));
#40617=CARTESIAN_POINT('Ctrl Pts',(0.274909983304274,-0.563939196325089,
-0.72625));
#40618=CARTESIAN_POINT('Ctrl Pts',(0.268259434616051,-0.566625287495204,
-0.72625));
#40619=CARTESIAN_POINT('Ctrl Pts',(0.261569430937461,-0.56919401133889,
-0.72625));
#40620=CARTESIAN_POINT('Ctrl Pts',(0.24504403797673,-0.575539175402156,
-0.72625));
#40621=CARTESIAN_POINT('Ctrl Pts',(0.22827539249502,-0.581169692531995,
-0.72625));
#40622=CARTESIAN_POINT('Ctrl Pts',(0.211302790467133,-0.586059341419264,
-0.72625));
#40623=CARTESIAN_POINT('Ctrl Pts',(0.186757466137251,-0.593130621214788,
-0.72625));
#40624=CARTESIAN_POINT('Ctrl Pts',(0.161785415196603,-0.59865351137275,
-0.72625));
#40625=CARTESIAN_POINT('Ctrl Pts',(0.136536085409988,-0.602617904235996,
-0.72625));
#40626=CARTESIAN_POINT('Ctrl Pts',(0.121331994017328,-0.605005095972118,
-0.72625));
#40627=CARTESIAN_POINT('Ctrl Pts',(0.106027319098842,-0.606826713214505,
-0.72625));
#40628=CARTESIAN_POINT('Ctrl Pts',(0.0906551911462363,-0.608076286524706,
-0.72625));
#40629=CARTESIAN_POINT('Ctrl Pts',(0.0807017050580736,-0.608885387944989,
-0.72625));
#40630=CARTESIAN_POINT('Ctrl Pts',(0.0707139335318761,-0.609454531657244,
-0.72625));
#40631=CARTESIAN_POINT('Ctrl Pts',(0.0607349132915466,-0.609780907620945,
-0.72625));
#40632=CARTESIAN_POINT('Ctrl Pts',(0.0304829114827247,-0.610770336042418,
-0.72625));
#40633=CARTESIAN_POINT('Ctrl Pts',(0.00026269855040462,-0.609539106859905,
-0.72625));
#40634=CARTESIAN_POINT('Ctrl Pts',(-0.0296765491183145,-0.606076614826858,
-0.72625));
#40635=CARTESIAN_POINT('Ctrl Pts',(-0.0505970509746303,-0.603657146181342,
-0.72625));
#40636=CARTESIAN_POINT('Ctrl Pts',(-0.0713804846129305,-0.600147135085872,
-0.72625));
#40637=CARTESIAN_POINT('Ctrl Pts',(-0.0919381111643192,-0.595528262125297,
-0.72625));
#40638=CARTESIAN_POINT('Ctrl Pts',(-0.106527466400008,-0.592250336133116,
-0.72625));
#40639=CARTESIAN_POINT('Ctrl Pts',(-0.121003020799398,-0.588413642459459,
-0.72625));
#40640=CARTESIAN_POINT('Ctrl Pts',(-0.135334733667594,-0.584028646208658,
-0.72625));
#40641=CARTESIAN_POINT('Ctrl Pts',(-0.142283241551999,-0.581902649037072,
-0.72625));
#40642=CARTESIAN_POINT('Ctrl Pts',(-0.149197909713515,-0.579647727780099,
-0.72625));
#40643=CARTESIAN_POINT('Ctrl Pts',(-0.156075139006189,-0.577264873365136,
-0.72625));
#40644=CARTESIAN_POINT('Ctrl Pts',(-0.162218696929079,-0.575136224821203,
-0.72625));
#40645=CARTESIAN_POINT('Ctrl Pts',(-0.168323407331897,-0.572908574802006,
-0.72625));
#40646=CARTESIAN_POINT('Ctrl Pts',(-0.174385772185665,-0.570583909329584,
-0.72625));
#40647=CARTESIAN_POINT('Ctrl Pts',(-0.202180396576834,-0.559925823714537,
-0.72625));
#40648=CARTESIAN_POINT('Ctrl Pts',(-0.229096085134795,-0.547228928394159,
-0.72625));
#40649=CARTESIAN_POINT('Ctrl Pts',(-0.254911830827949,-0.532610490159781,
-0.72625));
#40650=CARTESIAN_POINT('Ctrl Pts',(-0.280232930328858,-0.518272150547971,
-0.72625));
#40651=CARTESIAN_POINT('Ctrl Pts',(-0.304496791249199,-0.502084414991184,
-0.72625));
#40652=CARTESIAN_POINT('Ctrl Pts',(-0.327463169349827,-0.484120324940849,
-0.72625));
#40653=CARTESIAN_POINT('Ctrl Pts',(-0.336303377345208,-0.477205595426387,
-0.72625));
#40654=CARTESIAN_POINT('Ctrl Pts',(-0.344950933524855,-0.470027335227127,
-0.72625));
#40655=CARTESIAN_POINT('Ctrl Pts',(-0.353390396098497,-0.462588545080562,
-0.72625));
#40656=CARTESIAN_POINT('Ctrl Pts',(-0.353390396098497,-0.462588545080562,
-0.72625));
#40657=CARTESIAN_POINT('Ctrl Pts',(-0.390098616296541,-0.430232841820501,
-0.72625));
#40658=CARTESIAN_POINT('Ctrl Pts',(-0.444801171208843,-0.377290789425656,
-0.72625));
#40659=CARTESIAN_POINT('Ctrl Pts',(-0.528751914986461,-0.232845672680449,
-0.72625));
#40660=CARTESIAN_POINT('Ctrl Pts',(-0.554058019076711,-0.161663831518696,
-0.72625));
#40661=CARTESIAN_POINT('Ctrl Pts',(-0.565534825602701,-0.0874095162469292,
-0.72625));
#40662=CARTESIAN_POINT('Origin',(0.,0.,-0.72625));
#40663=CARTESIAN_POINT('Origin',(0.,0.,-0.930039011722494));
#40664=CARTESIAN_POINT('Ctrl Pts',(-0.575296847308758,-0.0889183421516984,
-0.742528335043099));
#40665=CARTESIAN_POINT('Ctrl Pts',(-0.560843190848635,-0.182432714916398,
-0.73906984429286));
#40666=CARTESIAN_POINT('Ctrl Pts',(-0.485503739143021,-0.362196725342242,
-0.732152862792381));
#40667=CARTESIAN_POINT('Ctrl Pts',(-0.259159251093108,-0.547465824506594,
-0.721777390541662));
#40668=CARTESIAN_POINT('Ctrl Pts',(0.0275428991067036,-0.605077845001504,
-0.711401918290945));
#40669=CARTESIAN_POINT('Ctrl Pts',(0.307852790782245,-0.521644157320061,
-0.701026446040225));
#40670=CARTESIAN_POINT('Ctrl Pts',(0.516379630382223,-0.316594299265632,
-0.690650973789508));
#40671=CARTESIAN_POINT('Ctrl Pts',(0.604531894922356,-0.037741447613471,
-0.680275501538789));
#40672=CARTESIAN_POINT('Ctrl Pts',(0.551748054568745,0.249911729814406,
-0.669900029288071));
#40673=CARTESIAN_POINT('Ctrl Pts',(0.370338916630071,0.479302937024635,
-0.659524557037353));
#40674=CARTESIAN_POINT('Ctrl Pts',(0.102593005245228,0.596956344106599,
-0.649149084786633));
#40675=CARTESIAN_POINT('Ctrl Pts',(-0.189069595066604,0.575443129800777,
-0.638773612535917));
#40676=CARTESIAN_POINT('Ctrl Pts',(-0.436655282749753,0.419778941359981,
-0.628398140285197));
#40677=CARTESIAN_POINT('Ctrl Pts',(-0.582444898128172,0.166253064936486,
-0.618022668034479));
#40678=CARTESIAN_POINT('Ctrl Pts',(-0.59245118529686,-0.126030790814807,
-0.607647195783762));
#40679=CARTESIAN_POINT('Ctrl Pts',(-0.464341322608817,-0.388933533934673,
-0.597271723533042));
#40680=CARTESIAN_POINT('Ctrl Pts',(-0.227981169867371,-0.561165524309829,
-0.586896251282325));
#40681=CARTESIAN_POINT('Ctrl Pts',(0.0615274613730338,-0.602574918002375,
-0.576520779031606));
#40682=CARTESIAN_POINT('Ctrl Pts',(0.336692401993215,-0.503508078945706,
-0.566145306780887));
#40683=CARTESIAN_POINT('Ctrl Pts',(0.533365395804019,-0.287060123544462,
-0.55576983453017));
#40684=CARTESIAN_POINT('Ctrl Pts',(0.605696737111815,-0.00369082231710978,
-0.545394362279451));
#40685=CARTESIAN_POINT('Ctrl Pts',(0.536824069047151,0.280538907457441,
-0.535018890028733));
#40686=CARTESIAN_POINT('Ctrl Pts',(0.342803440542624,0.499367560825895,
-0.524643417778015));
#40687=CARTESIAN_POINT('Ctrl Pts',(0.0688662178762295,0.601780361666548,
-0.514267945527296));
#40688=CARTESIAN_POINT('Ctrl Pts',(-0.221125550821607,0.563902163890325,
-0.503892473276578));
#40689=CARTESIAN_POINT('Ctrl Pts',(-0.459567075698392,0.394563382218786,
-0.493517001025859));
#40690=CARTESIAN_POINT('Ctrl Pts',(-0.590871299173015,0.133241387995481,
-0.483141528775141));
#40691=CARTESIAN_POINT('Ctrl Pts',(-0.584427716440101,-0.159142715555849,
-0.472766056524423));
#40692=CARTESIAN_POINT('Ctrl Pts',(-0.441738497928306,-0.414426421825547,
-0.462390584273705));
#40693=CARTESIAN_POINT('Ctrl Pts',(-0.196068293388198,-0.573096313010961,
-0.452015112022986));
#40694=CARTESIAN_POINT('Ctrl Pts',(0.0953106421677161,-0.598162219760071,
-0.441639639772268));
#40695=CARTESIAN_POINT('Ctrl Pts',(0.364470133516224,-0.483780612916302,
-0.43126416752155));
#40696=CARTESIAN_POINT('Ctrl Pts',(0.548661948506927,-0.256616885491388,
-0.420888695270832));
#40697=CARTESIAN_POINT('Ctrl Pts',(0.60494607893493,0.0303710592533639,
-0.410513223020113));
#40698=CARTESIAN_POINT('Ctrl Pts',(0.520201197869222,0.310278702773021,
-0.400137750769395));
#40699=CARTESIAN_POINT('Ctrl Pts',(0.314183589749731,0.517852132939369,
-0.389762278518676));
#40700=CARTESIAN_POINT('Ctrl Pts',(0.0349214353255983,0.604700465533282,
-0.379386806267958));
#40701=CARTESIAN_POINT('Ctrl Pts',(-0.252481833942362,0.550577045637576,
-0.36901133401724));
#40702=CARTESIAN_POINT('Ctrl Pts',(-0.481024876325774,0.368099481148946,
-0.358635861766521));
#40703=CARTESIAN_POINT('Ctrl Pts',(-0.597428233573601,0.0998081428603092,
-0.348260389515803));
#40704=CARTESIAN_POINT('Ctrl Pts',(-0.574555188931242,-0.191751126529284,
-0.337884917265085));
#40705=CARTESIAN_POINT('Ctrl Pts',(-0.417738057072088,-0.43860811139261,
-0.327509445014367));
#40706=CARTESIAN_POINT('Ctrl Pts',(-0.163535079971663,-0.583213886268098,
-0.317133972763648));
#40707=CARTESIAN_POINT('Ctrl Pts',(0.128792271407237,-0.591857001983,-0.30675850051293));
#40708=CARTESIAN_POINT('Ctrl Pts',(0.3910947206114,-0.462522516893444,-0.296383028262211));
#40709=CARTESIAN_POINT('Ctrl Pts',(0.562222594861329,-0.225361740621548,
-0.286007556011493));
#40710=CARTESIAN_POINT('Ctrl Pts',(0.602281436660628,0.0643368521302563,
-0.275632083760774));
#40711=CARTESIAN_POINT('Ctrl Pts',(0.501932467413927,0.339036806050298,
-0.265256611510057));
#40712=CARTESIAN_POINT('Ctrl Pts',(0.284569694815385,0.534698285003551,
-0.254881139259338));
#40713=CARTESIAN_POINT('Ctrl Pts',(0.00086616792234151,0.605707347412463,
-0.24450566700862));
#40714=CARTESIAN_POINT('Ctrl Pts',(-0.283039297466054,0.535509992112656,
-0.234130194757901));
#40715=CARTESIAN_POINT('Ctrl Pts',(-0.500960755684866,0.340470892555017,
-0.223754722507184));
#40716=CARTESIAN_POINT('Ctrl Pts',(-0.602094991516589,0.066059236182406,
-0.213379250256465));
#40717=CARTESIAN_POINT('Ctrl Pts',(-0.562864788572229,-0.223753096954469,
-0.203003778005747));
#40718=CARTESIAN_POINT('Ctrl Pts',(-0.392416023107415,-0.46140161814604,
-0.192628305755028));
#40719=CARTESIAN_POINT('Ctrl Pts',(-0.130484291345699,-0.591487175311845,
-0.18225283350431));
#40720=CARTESIAN_POINT('Ctrl Pts',(0.161866082666176,-0.583677346042729,
-0.171877361253592));
#40721=CARTESIAN_POINT('Ctrl Pts',(0.416482587440825,-0.439804754427654,
-0.161501889002873));
#40722=CARTESIAN_POINT('Ctrl Pts',(0.574003120398452,-0.193386213509922,
-0.151126416752155));
#40723=CARTESIAN_POINT('Ctrl Pts',(0.597713822063416,0.0980843175241036,
-0.140750944501437));
#40724=CARTESIAN_POINT('Ctrl Pts',(0.482070740684944,0.366753526971408,
-0.130375472250718));
#40725=CARTESIAN_POINT('Ctrl Pts',(0.33006409929725,0.48875809000787,-0.12345849075024));
#40726=CARTESIAN_POINT('Ctrl Pts',(0.244165145742818,0.528447079373888,
-0.12));
#40727=CARTESIAN_POINT('Ctrl Pts',(-0.572789913424251,-0.088530868439758,
-0.741207811940174));
#40728=CARTESIAN_POINT('Ctrl Pts',(-0.558399233618351,-0.181637785669948,
-0.737749321189935));
#40729=CARTESIAN_POINT('Ctrl Pts',(-0.483388100289454,-0.360618378632632,
-0.730832339689455));
#40730=CARTESIAN_POINT('Ctrl Pts',(-0.258029928191081,-0.545080184451301,
-0.720456867438737));
#40731=CARTESIAN_POINT('Ctrl Pts',(0.0274228758760488,-0.602441133683186,
-0.71008139518802));
#40732=CARTESIAN_POINT('Ctrl Pts',(0.306511283236796,-0.519371028784781,
-0.699705922937301));
#40733=CARTESIAN_POINT('Ctrl Pts',(0.514129439073967,-0.315214697079695,
-0.689330450686582));
#40734=CARTESIAN_POINT('Ctrl Pts',(0.601897569304816,-0.0375769852070561,
-0.678954978435864));
#40735=CARTESIAN_POINT('Ctrl Pts',(0.549343741066101,0.248822707591735,
-0.668579506185146));
#40736=CARTESIAN_POINT('Ctrl Pts',(0.368725117019615,0.477214312364194,
-0.658204033934427));
#40737=CARTESIAN_POINT('Ctrl Pts',(0.102145942950475,0.594355029845439,
-0.64782856168371));
#40738=CARTESIAN_POINT('Ctrl Pts',(-0.188245699875266,0.572935561990258,
-0.63745308943299));
#40739=CARTESIAN_POINT('Ctrl Pts',(-0.434752500966896,0.417949700435014,
-0.627077617182273));
#40740=CARTESIAN_POINT('Ctrl Pts',(-0.579906819258096,0.165528595720715,
-0.616702144931554));
#40741=CARTESIAN_POINT('Ctrl Pts',(-0.589869502742826,-0.125481595359992,
-0.606326672680836));
#40742=CARTESIAN_POINT('Ctrl Pts',(-0.462317895324597,-0.387238705832832,
-0.595951200430118));
#40743=CARTESIAN_POINT('Ctrl Pts',(-0.226987712476072,-0.558720173060809,
-0.585575728179399));
#40744=CARTESIAN_POINT('Ctrl Pts',(0.061259347513968,-0.599949119974886,
-0.575200255928681));
#40745=CARTESIAN_POINT('Ctrl Pts',(0.335225221367258,-0.501313977462673,
-0.564824783677962));
#40746=CARTESIAN_POINT('Ctrl Pts',(0.531041187207166,-0.285809221982231,
-0.554449311427245));
#40747=CARTESIAN_POINT('Ctrl Pts',(0.603057335353469,-0.00367473908207673,
-0.544073839176526));
#40748=CARTESIAN_POINT('Ctrl Pts',(0.534484788834912,0.27931642293625,-0.533698366925808));
#40749=CARTESIAN_POINT('Ctrl Pts',(0.341309630277037,0.497191502185792,
-0.523322894675089));
#40750=CARTESIAN_POINT('Ctrl Pts',(0.0685661244376943,0.599158026020019,
-0.512947422424371));
#40751=CARTESIAN_POINT('Ctrl Pts',(-0.220161967675312,0.561444887382637,
-0.502571950173652));
#40752=CARTESIAN_POINT('Ctrl Pts',(-0.457564452812476,0.392844021322498,
-0.492196477922934));
#40753=CARTESIAN_POINT('Ctrl Pts',(-0.588296501175234,0.132660771439031,
-0.481821005672216));
#40754=CARTESIAN_POINT('Ctrl Pts',(-0.581880997186273,-0.15844923061937,
-0.471445533421498));
#40755=CARTESIAN_POINT('Ctrl Pts',(-0.439813565372604,-0.412620505168844,
-0.461070061170779));
#40756=CARTESIAN_POINT('Ctrl Pts',(-0.195213900477338,-0.570598971811038,
-0.450694588920061));
#40757=CARTESIAN_POINT('Ctrl Pts',(0.0948953137350028,-0.595555650634202,
-0.440319116669343));
#40758=CARTESIAN_POINT('Ctrl Pts',(0.362881907837736,-0.481672476414757,
-0.429943644418624));
#40759=CARTESIAN_POINT('Ctrl Pts',(0.546271083206054,-0.255498644270525,
-0.419568172167906));
#40760=CARTESIAN_POINT('Ctrl Pts',(0.602309948266564,0.0302387134402138,
-0.409192699917188));
#40761=CARTESIAN_POINT('Ctrl Pts',(0.517934353964987,0.308926623252875,
-0.398817227666469));
#40762=CARTESIAN_POINT('Ctrl Pts',(0.312814494180264,0.51559552538895,-0.388441755415751));
#40763=CARTESIAN_POINT('Ctrl Pts',(0.0347692606610258,0.602065405157036,
-0.378066283165032));
#40764=CARTESIAN_POINT('Ctrl Pts',(-0.251381611742667,0.548177835053618,
-0.367690810914315));
#40765=CARTESIAN_POINT('Ctrl Pts',(-0.478928748302335,0.366495440119418,
-0.357315338663596));
#40766=CARTESIAN_POINT('Ctrl Pts',(-0.594824862887321,0.0993732159874641,
-0.346939866412878));
#40767=CARTESIAN_POINT('Ctrl Pts',(-0.572051490491107,-0.190915546230564,
-0.336564394162159));
#40768=CARTESIAN_POINT('Ctrl Pts',(-0.415917709537047,-0.436696819900557,
-0.326188921911441));
#40769=CARTESIAN_POINT('Ctrl Pts',(-0.162822454740063,-0.580672456435957,
-0.315813449660722));
#40770=CARTESIAN_POINT('Ctrl Pts',(0.128231042451125,-0.589277908658029,
-0.305437977410005));
#40771=CARTESIAN_POINT('Ctrl Pts',(0.389390474855656,-0.460507015290604,
-0.295062505159286));
#40772=CARTESIAN_POINT('Ctrl Pts',(0.55977263729338,-0.224379697731525,
-0.284687032908568));
#40773=CARTESIAN_POINT('Ctrl Pts',(0.599656917513555,0.0640564959887923,
-0.274311560657849));
#40774=CARTESIAN_POINT('Ctrl Pts',(0.499745231865169,0.337559409379268,
-0.263936088407131));
#40775=CARTESIAN_POINT('Ctrl Pts',(0.283329645611625,0.532368268173216,
-0.253560616156412));
#40776=CARTESIAN_POINT('Ctrl Pts',(0.000862393495920531,0.603067899411643,
-0.243185143905695));
#40777=CARTESIAN_POINT('Ctrl Pts',(-0.281805917196665,0.533176438173738,
-0.232809671654976));
#40778=CARTESIAN_POINT('Ctrl Pts',(-0.498777754444496,0.338987246642003,
-0.222434199404258));
#40779=CARTESIAN_POINT('Ctrl Pts',(-0.59947128492484,0.0657713745817691,
-0.21205872715354));
#40780=CARTESIAN_POINT('Ctrl Pts',(-0.560412032373069,-0.22277806404098,
-0.201683254902822));
#40781=CARTESIAN_POINT('Ctrl Pts',(-0.390706019979498,-0.459391000797317,
-0.191307782652103));
#40782=CARTESIAN_POINT('Ctrl Pts',(-0.129915688452667,-0.588909693965184,
-0.180932310401385));
#40783=CARTESIAN_POINT('Ctrl Pts',(0.161160728835196,-0.581133895809618,
-0.170556838150666));
#40784=CARTESIAN_POINT('Ctrl Pts',(0.414667713695017,-0.437888250026621,
-0.160181365899948));
#40785=CARTESIAN_POINT('Ctrl Pts',(0.571501821867847,-0.192543504893118,
-0.14980589364923));
#40786=CARTESIAN_POINT('Ctrl Pts',(0.59510921853944,0.0976568959835189,
-0.139430421398511));
#40787=CARTESIAN_POINT('Ctrl Pts',(0.479970030309954,0.365155364897378,
-0.129054949147793));
#40788=CARTESIAN_POINT('Ctrl Pts',(0.328625842563643,0.48662824094783,-0.122137967647314));
#40789=CARTESIAN_POINT('Ctrl Pts',(0.243101163069974,0.526144299694755,
-0.118679476897075));
#40790=CARTESIAN_POINT('Ctrl Pts',(-0.567659051683199,-0.0877378383337212,
-0.736720279419894));
#40791=CARTESIAN_POINT('Ctrl Pts',(-0.553397145962568,-0.180011594221972,
-0.733261788669655));
#40792=CARTESIAN_POINT('Ctrl Pts',(-0.479058246054666,-0.357387603482484,
-0.726344807169176));
#40793=CARTESIAN_POINT('Ctrl Pts',(-0.255718555936061,-0.540197843291853,
-0.715969334918457));
#40794=CARTESIAN_POINT('Ctrl Pts',(0.0271772062107107,-0.597044615620193,
-0.70559386266774));
#40795=CARTESIAN_POINT('Ctrl Pts',(0.303765706721173,-0.514718796922303,
-0.695218390417021));
#40796=CARTESIAN_POINT('Ctrl Pts',(0.509524091217568,-0.31239111466724,
-0.684842918166304));
#40797=CARTESIAN_POINT('Ctrl Pts',(0.596506044544102,-0.0372404028672287,
-0.674467445915583));
#40798=CARTESIAN_POINT('Ctrl Pts',(0.544422964561454,0.246593873216988,
-0.664091973664867));
#40799=CARTESIAN_POINT('Ctrl Pts',(0.365422243793962,0.472939636786017,
-0.653716501414147));
#40800=CARTESIAN_POINT('Ctrl Pts',(0.101230964976293,0.589031066186152,
-0.643341029163429));
#40801=CARTESIAN_POINT('Ctrl Pts',(-0.186559479142561,0.567803461338418,
-0.632965556912711));
#40802=CARTESIAN_POINT('Ctrl Pts',(-0.430858183277496,0.414205895078914,
-0.622590084661993));
#40803=CARTESIAN_POINT('Ctrl Pts',(-0.574712274150216,0.164045864589158,
-0.612214612411273));
#40804=CARTESIAN_POINT('Ctrl Pts',(-0.584585716474985,-0.12435758741187,
-0.601839140160557));
#40805=CARTESIAN_POINT('Ctrl Pts',(-0.458176659071989,-0.383769995346564,
-0.591463667909837));
#40806=CARTESIAN_POINT('Ctrl Pts',(-0.224954458417602,-0.553715408447872,
-0.58108819565912));
#40807=CARTESIAN_POINT('Ctrl Pts',(0.0607106137732936,-0.594575045006088,
-0.570712723408401));
#40808=CARTESIAN_POINT('Ctrl Pts',(0.332222424267133,-0.496823431812653,
-0.560337251157683));
#40809=CARTESIAN_POINT('Ctrl Pts',(0.526284358561762,-0.283249071234861,
-0.549961778906964));
#40810=CARTESIAN_POINT('Ctrl Pts',(0.597655418369305,-0.00364182241635053,
-0.539586306656246));
#40811=CARTESIAN_POINT('Ctrl Pts',(0.529697113950753,0.276814431763831,
-0.529210834405528));
#40812=CARTESIAN_POINT('Ctrl Pts',(0.3382523317741,0.492737883828088,-0.51883536215481));
#40813=CARTESIAN_POINT('Ctrl Pts',(0.0679519398645962,0.593791037299236,
-0.508459889904091));
#40814=CARTESIAN_POINT('Ctrl Pts',(-0.21818985556821,0.556415716034123,
-0.498084417653373));
#40815=CARTESIAN_POINT('Ctrl Pts',(-0.453465795779581,0.389325100871067,
-0.487708945402654));
#40816=CARTESIAN_POINT('Ctrl Pts',(-0.583026805120096,0.131472455781011,
-0.477333473151936));
#40817=CARTESIAN_POINT('Ctrl Pts',(-0.576668768336853,-0.157029913516757,
-0.466958000901218));
#40818=CARTESIAN_POINT('Ctrl Pts',(-0.43587391282357,-0.40892443585002,
-0.4565825286505));
#40819=CARTESIAN_POINT('Ctrl Pts',(-0.193465261960535,-0.565487802282046,
-0.446207056399781));
#40820=CARTESIAN_POINT('Ctrl Pts',(0.0940452840995342,-0.590220930375798,
-0.435831584149063));
#40821=CARTESIAN_POINT('Ctrl Pts',(0.359631374553251,-0.477357870525102,
-0.425456111898345));
#40822=CARTESIAN_POINT('Ctrl Pts',(0.54137783198586,-0.253210002072044,
-0.415080639647626));
#40823=CARTESIAN_POINT('Ctrl Pts',(0.596914726041016,0.0299678486150587,
-0.404705167396908));
#40824=CARTESIAN_POINT('Ctrl Pts',(0.513294930449014,0.306159397194876,
-0.394329695146189));
#40825=CARTESIAN_POINT('Ctrl Pts',(0.310012442319218,0.510977052049793,
-0.383954222895472));
#40826=CARTESIAN_POINT('Ctrl Pts',(0.0344578132269551,0.596672373438936,
-0.373578750644753));
#40827=CARTESIAN_POINT('Ctrl Pts',(-0.249129848073962,0.54326750400601,
-0.363203278394035));
#40828=CARTESIAN_POINT('Ctrl Pts',(-0.474638719497963,0.36321253843442,
-0.352827806143316));
#40829=CARTESIAN_POINT('Ctrl Pts',(-0.589496688697369,0.0984830753129765,
-0.342452333892598));
#40830=CARTESIAN_POINT('Ctrl Pts',(-0.566927309952081,-0.189205410441921,
-0.33207686164188));
#40831=CARTESIAN_POINT('Ctrl Pts',(-0.412192105340198,-0.432785085759324,
-0.321701389391161));
#40832=CARTESIAN_POINT('Ctrl Pts',(-0.161363964260157,-0.575471053151198,
-0.311325917140443));
#40833=CARTESIAN_POINT('Ctrl Pts',(0.127082406321203,-0.583999421597136,
-0.300950444889725));
#40834=CARTESIAN_POINT('Ctrl Pts',(0.385902489716337,-0.456382000099439,
-0.290574972639006));
#40835=CARTESIAN_POINT('Ctrl Pts',(0.554758445225278,-0.222369805099424,
-0.280199500388288));
#40836=CARTESIAN_POINT('Ctrl Pts',(0.594285459917798,0.0634827066596925,
-0.26982402813757));
#40837=CARTESIAN_POINT('Ctrl Pts',(0.495268738400242,0.334535703640292,
-0.259448555886852));
#40838=CARTESIAN_POINT('Ctrl Pts',(0.2807917056779,0.527599552194623,-0.249073083636133));
#40839=CARTESIAN_POINT('Ctrl Pts',(0.000854668789314793,0.597665887673856,
-0.238697611385415));
#40840=CARTESIAN_POINT('Ctrl Pts',(-0.279281626703832,0.528400483157397,
-0.228322139134696));
#40841=CARTESIAN_POINT('Ctrl Pts',(-0.494309926255865,0.33595075051375,
-0.217946666883978));
#40842=CARTESIAN_POINT('Ctrl Pts',(-0.594101491946025,0.0651822251072623,
-0.20757119463326));
#40843=CARTESIAN_POINT('Ctrl Pts',(-0.555392109356301,-0.220782520067741,
-0.197195722382542));
#40844=CARTESIAN_POINT('Ctrl Pts',(-0.387206257766804,-0.455275978496852,
-0.186820250131823));
#40845=CARTESIAN_POINT('Ctrl Pts',(-0.12875194816593,-0.583634512881856,
-0.176444777881105));
#40846=CARTESIAN_POINT('Ctrl Pts',(0.159717095872789,-0.575928343928385,
-0.166069305630386));
#40847=CARTESIAN_POINT('Ctrl Pts',(0.410953360921151,-0.433965873811025,
-0.155693833379668));
#40848=CARTESIAN_POINT('Ctrl Pts',(0.56638245664278,-0.19081872650705,-0.14531836112895));
#40849=CARTESIAN_POINT('Ctrl Pts',(0.589778714899386,0.0967820086525517,
-0.134942888878231));
#40850=CARTESIAN_POINT('Ctrl Pts',(0.475670209653462,0.361884724579745,
-0.124567416627513));
#40851=CARTESIAN_POINT('Ctrl Pts',(0.325682910944071,0.482268822061771,
-0.117650435127034));
#40852=CARTESIAN_POINT('Ctrl Pts',(0.240923543618988,0.52143127386398,-0.114191944376795));
#40853=CARTESIAN_POINT('Ctrl Pts',(-0.565534825602701,-0.0874095162469292,
-0.730063108302008));
#40854=CARTESIAN_POINT('Ctrl Pts',(-0.551326779224584,-0.179334805112556,
-0.726604617551768));
#40855=CARTESIAN_POINT('Ctrl Pts',(-0.477264922845315,-0.356051984665031,
-0.719687636051289));
#40856=CARTESIAN_POINT('Ctrl Pts',(-0.254761731927526,-0.53817525012622,
-0.70931216380057));
#40857=CARTESIAN_POINT('Ctrl Pts',(0.0270755978711435,-0.594810612863019,
-0.698936691549854));
#40858=CARTESIAN_POINT('Ctrl Pts',(0.302628807416583,-0.512792230164359,
-0.688561219299133));
#40859=CARTESIAN_POINT('Ctrl Pts',(0.50761721588506,-0.311222099281607,
-0.678185747048417));
#40860=CARTESIAN_POINT('Ctrl Pts',(0.594273598793385,-0.0371009731803471,
-0.667810274797697));
#40861=CARTESIAN_POINT('Ctrl Pts',(0.542385460253111,0.245670963329659,
-0.65743480254698));
#40862=CARTESIAN_POINT('Ctrl Pts',(0.364054642350776,0.471169667728722,
-0.647059330296261));
#40863=CARTESIAN_POINT('Ctrl Pts',(0.100852108287779,0.586826601489527,
-0.636683858045543));
#40864=CARTESIAN_POINT('Ctrl Pts',(-0.18586127840427,0.565678452235062,
-0.626308385794825));
#40865=CARTESIAN_POINT('Ctrl Pts',(-0.429245689780927,0.412655721589033,
-0.615932913544106));
#40866=CARTESIAN_POINT('Ctrl Pts',(-0.57256140525216,0.163431921469813,
-0.605557441293388));
#40867=CARTESIAN_POINT('Ctrl Pts',(-0.582397895750055,-0.123892177788475,
-0.59518196904267));
#40868=CARTESIAN_POINT('Ctrl Pts',(-0.456461926261484,-0.382333730273898,
-0.58480649679195));
#40869=CARTESIAN_POINT('Ctrl Pts',(-0.224112563030628,-0.551643120531786,
-0.574431024541234));
#40870=CARTESIAN_POINT('Ctrl Pts',(0.0604834033970661,-0.592349839120952,
-0.564055552290514));
#40871=CARTESIAN_POINT('Ctrl Pts',(0.330979076979619,-0.494964062864097,
-0.553680080039796));
#40872=CARTESIAN_POINT('Ctrl Pts',(0.524314731628871,-0.282189007416862,
-0.543304607789078));
#40873=CARTESIAN_POINT('Ctrl Pts',(0.59541868420382,-0.00362819285028554,
-0.53292913553836));
#40874=CARTESIAN_POINT('Ctrl Pts',(0.527714714733413,0.275778449697644,
-0.522553663287641));
#40875=CARTESIAN_POINT('Ctrl Pts',(0.336986417462755,0.490893805070386,
-0.512178191036923));
#40876=CARTESIAN_POINT('Ctrl Pts',(0.0676976287329768,0.591568765635781,
-0.501802718786204));
#40877=CARTESIAN_POINT('Ctrl Pts',(-0.217373276834094,0.554333322057082,
-0.491427246535487));
#40878=CARTESIAN_POINT('Ctrl Pts',(-0.45176869338931,0.387868045972245,
-0.481051774284768));
#40879=CARTESIAN_POINT('Ctrl Pts',(-0.580844818752399,0.130980418187211,
-0.47067630203405));
#40880=CARTESIAN_POINT('Ctrl Pts',(-0.574510577015094,-0.15644222676267,
-0.460300829783332));
#40881=CARTESIAN_POINT('Ctrl Pts',(-0.434242648313164,-0.407394030152414,
-0.449925357532613));
#40882=CARTESIAN_POINT('Ctrl Pts',(-0.192741215380677,-0.563371455889674,
-0.439549885281895));
#40883=CARTESIAN_POINT('Ctrl Pts',(0.0936933182447148,-0.588012019888873,
-0.429174413031176));
#40884=CARTESIAN_POINT('Ctrl Pts',(0.358285448860346,-0.475571351694678,
-0.418798940780458));
#40885=CARTESIAN_POINT('Ctrl Pts',(0.539351717510894,-0.252262359926223,
-0.40842346852974));
#40886=CARTESIAN_POINT('Ctrl Pts',(0.594680763925633,0.0298556935021776,
-0.398047996279021));
#40887=CARTESIAN_POINT('Ctrl Pts',(0.511373916644878,0.305013591161334,
-0.387672524028303));
#40888=CARTESIAN_POINT('Ctrl Pts',(0.308852216207758,0.509064712939559,
-0.377297051777585));
#40889=CARTESIAN_POINT('Ctrl Pts',(0.0343288543557777,0.594439318331672,
-0.366921579526867));
#40890=CARTESIAN_POINT('Ctrl Pts',(-0.24819747596453,0.541234317405916,
-0.356546107276148));
#40891=CARTESIAN_POINT('Ctrl Pts',(-0.47286237712969,0.361853210182931,
-0.34617063502543));
#40892=CARTESIAN_POINT('Ctrl Pts',(-0.587290488696427,0.0981145009599544,
-0.335795162774712));
#40893=CARTESIAN_POINT('Ctrl Pts',(-0.564805576179397,-0.188497306419811,
-0.325419690523993));
#40894=CARTESIAN_POINT('Ctrl Pts',(-0.410649470345074,-0.431165381227568,
-0.315044218273275));
#40895=CARTESIAN_POINT('Ctrl Pts',(-0.160760057250731,-0.573317344299916,
-0.304668746022556));
#40896=CARTESIAN_POINT('Ctrl Pts',(0.126606798538242,-0.581813795190408,
-0.294293273771839));
#40897=CARTESIAN_POINT('Ctrl Pts',(0.384458244017007,-0.454673983786817,
-0.28391780152112));
#40898=CARTESIAN_POINT('Ctrl Pts',(0.552682253554872,-0.22153758281298,
-0.273542329270402));
#40899=CARTESIAN_POINT('Ctrl Pts',(0.592061337976905,0.0632451216395426,
-0.263166857019683));
#40900=CARTESIAN_POINT('Ctrl Pts',(0.493415187671003,0.333283698981943,
-0.252791384768965));
#40901=CARTESIAN_POINT('Ctrl Pts',(0.279740839024693,0.525625002899427,
-0.242415912518246));
#40902=CARTESIAN_POINT('Ctrl Pts',(0.000851469340100179,0.595429114790003,
-0.232040440267529));
#40903=CARTESIAN_POINT('Ctrl Pts',(-0.278236409456736,0.526422935678427,
-0.22166496801681));
#40904=CARTESIAN_POINT('Ctrl Pts',(-0.492459967408646,0.334693451733073,
-0.211289495766092));
#40905=CARTESIAN_POINT('Ctrl Pts',(-0.591878051853725,0.064938276044851,
-0.200914023515373));
#40906=CARTESIAN_POINT('Ctrl Pts',(-0.553313559229366,-0.219956231049899,
-0.190538551264655));
#40907=CARTESIAN_POINT('Ctrl Pts',(-0.385757106908071,-0.453572115751417,
-0.180163079013937));
#40908=CARTESIAN_POINT('Ctrl Pts',(-0.128270143213515,-0.581450223831547,
-0.169787606763218));
#40909=CARTESIAN_POINT('Ctrl Pts',(0.159119453673079,-0.573772979850855,
-0.1594121345125));
#40910=CARTESIAN_POINT('Ctrl Pts',(0.409415160784161,-0.432341638655589,
-0.149036662261782));
#40911=CARTESIAN_POINT('Ctrl Pts',(0.564263161836264,-0.190104806275652,
-0.138661190011064));
#40912=CARTESIAN_POINT('Ctrl Pts',(0.587570656259513,0.0964202458298895,
-0.128285717760345));
#40913=CARTESIAN_POINT('Ctrl Pts',(0.473891720790759,0.360529415344193,
-0.117910245509627));
#40914=CARTESIAN_POINT('Ctrl Pts',(0.324461266232845,0.480465479019555,
-0.110993264009148));
#40915=CARTESIAN_POINT('Ctrl Pts',(0.240021988234213,0.519480035866726,
-0.107534773258909));
#40916=CARTESIAN_POINT('Ctrl Pts',(-0.565534825602701,-0.0874095162469292,
-0.72625));
#40917=CARTESIAN_POINT('Ctrl Pts',(-0.551326428453064,-0.179337074585254,
-0.722791509249761));
#40918=CARTESIAN_POINT('Ctrl Pts',(-0.477265386956567,-0.356050729042777,
-0.715874527749281));
#40919=CARTESIAN_POINT('Ctrl Pts',(-0.254761663575757,-0.538176058210883,
-0.705499055498564));
#40920=CARTESIAN_POINT('Ctrl Pts',(0.0270755327719408,-0.594810479406871,
-0.695123583247846));
#40921=CARTESIAN_POINT('Ctrl Pts',(0.302628938713621,-0.512792550344605,
-0.684748110997126));
#40922=CARTESIAN_POINT('Ctrl Pts',(0.507617355421152,-0.311222115434097,
-0.674372638746409));
#40923=CARTESIAN_POINT('Ctrl Pts',(0.594273793373837,-0.0371010254861046,
-0.66399716649569));
#40924=CARTESIAN_POINT('Ctrl Pts',(0.542385624529068,0.245671060423536,
-0.653621694244972));
#40925=CARTESIAN_POINT('Ctrl Pts',(0.364054758182736,0.471169804196079,
-0.643246221994254));
#40926=CARTESIAN_POINT('Ctrl Pts',(0.100852138510465,0.586826789571409,
-0.632870749743535));
#40927=CARTESIAN_POINT('Ctrl Pts',(-0.185861335713837,0.565678625875551,
-0.622495277492817));
#40928=CARTESIAN_POINT('Ctrl Pts',(-0.429245823844828,0.412655851503898,
-0.612119805242099));
#40929=CARTESIAN_POINT('Ctrl Pts',(-0.572561583514668,0.163431971728343,
-0.601744332991379));
#40930=CARTESIAN_POINT('Ctrl Pts',(-0.582398077309737,-0.123892216057582,
-0.591368860740663));
#40931=CARTESIAN_POINT('Ctrl Pts',(-0.4564620684611,-0.382333849583464,
-0.580993388489942));
#40932=CARTESIAN_POINT('Ctrl Pts',(-0.224112632886457,-0.551643292344488,
-0.570617916239226));
#40933=CARTESIAN_POINT('Ctrl Pts',(0.0604834222543564,-0.592350023747205,
-0.560242443988507));
#40934=CARTESIAN_POINT('Ctrl Pts',(0.330979180111506,-0.494964217078851,
-0.549866971737789));
#40935=CARTESIAN_POINT('Ctrl Pts',(0.524314895013938,-0.282189095361197,
-0.539491499487071));
#40936=CARTESIAN_POINT('Ctrl Pts',(0.595418869741894,-0.00362819397533901,
-0.529116027236352));
#40937=CARTESIAN_POINT('Ctrl Pts',(0.527714879176066,0.27577853563061,-0.518740554985634));
#40938=CARTESIAN_POINT('Ctrl Pts',(0.336986522471297,0.490893958039981,
-0.508365082734915));
#40939=CARTESIAN_POINT('Ctrl Pts',(0.0676976498285046,0.591568949974742,
-0.497989610484197));
#40940=CARTESIAN_POINT('Ctrl Pts',(-0.217373344570204,0.554333494794116,
-0.487614138233479));
#40941=CARTESIAN_POINT('Ctrl Pts',(-0.451768834165619,0.387868166836234,
-0.47723866598276));
#40942=CARTESIAN_POINT('Ctrl Pts',(-0.580844999750384,0.130980459002316,
-0.466863193732042));
#40943=CARTESIAN_POINT('Ctrl Pts',(-0.574510756039226,-0.156442275511923,
-0.456487721481324));
#40944=CARTESIAN_POINT('Ctrl Pts',(-0.434242783628202,-0.407394157101084,
-0.446112249230605));
#40945=CARTESIAN_POINT('Ctrl Pts',(-0.192741275441066,-0.563371631442748,
-0.435736776979888));
#40946=CARTESIAN_POINT('Ctrl Pts',(0.0936933474406337,-0.588012203120214,
-0.425361304729168));
#40947=CARTESIAN_POINT('Ctrl Pts',(0.35828556050624,-0.475571499888217,
-0.414985832478451));
#40948=CARTESIAN_POINT('Ctrl Pts',(0.539351885579122,-0.252262438534088,
-0.404610360227732));
#40949=CARTESIAN_POINT('Ctrl Pts',(0.594680949235049,0.0298557028055502,
-0.394234887977014));
#40950=CARTESIAN_POINT('Ctrl Pts',(0.511374075994885,0.30501368620711,-0.383859415726295));
#40951=CARTESIAN_POINT('Ctrl Pts',(0.308852312449722,0.509064871569989,
-0.373483943475578));
#40952=CARTESIAN_POINT('Ctrl Pts',(0.0343288650529642,0.594439503565886,
-0.363108471224859));
#40953=CARTESIAN_POINT('Ctrl Pts',(-0.248197553305573,0.5412344860607,-0.352732998974141));
#40954=CARTESIAN_POINT('Ctrl Pts',(-0.472862524479398,0.361853322940755,
-0.342357526723422));
#40955=CARTESIAN_POINT('Ctrl Pts',(-0.5872906717023,0.0981145315332149,
-0.331982054472704));
#40956=CARTESIAN_POINT('Ctrl Pts',(-0.564805752180611,-0.188497365157053,
-0.321606582221986));
#40957=CARTESIAN_POINT('Ctrl Pts',(-0.410649598305695,-0.431165515585077,
-0.311231109971268));
#40958=CARTESIAN_POINT('Ctrl Pts',(-0.160760107350392,-0.57331752294948,
-0.300855637720549));
#40959=CARTESIAN_POINT('Ctrl Pts',(0.126606838000238,-0.581813976495778,
-0.290480165469831));
#40960=CARTESIAN_POINT('Ctrl Pts',(0.3844583637991,-0.454674125457656,-0.280104693219112));
#40961=CARTESIAN_POINT('Ctrl Pts',(0.552682425815823,-0.221537651868143,
-0.269729220968394));
#40962=CARTESIAN_POINT('Ctrl Pts',(0.592061522393167,0.0632451413900827,
-0.259353748717676));
#40963=CARTESIAN_POINT('Ctrl Pts',(0.493415341577429,0.333283802752439,
-0.248978276466957));
#40964=CARTESIAN_POINT('Ctrl Pts',(0.279740925892577,0.525625166857998,
-0.238602804216239));
#40965=CARTESIAN_POINT('Ctrl Pts',(0.000851470205678055,0.595429299999864,
-0.228227331965521));
#40966=CARTESIAN_POINT('Ctrl Pts',(-0.278236497349112,0.526423100377946,
-0.217851859714802));
#40967=CARTESIAN_POINT('Ctrl Pts',(-0.492460118502939,0.334693554718123,
-0.207476387464084));
#40968=CARTESIAN_POINT('Ctrl Pts',(-0.591878240975039,0.0649382988775781,
-0.197100915213366));
#40969=CARTESIAN_POINT('Ctrl Pts',(-0.553313722354291,-0.219956304742787,
-0.186725442962648));
#40970=CARTESIAN_POINT('Ctrl Pts',(-0.385757245550577,-0.453572246869937,
-0.176349970711929));
#40971=CARTESIAN_POINT('Ctrl Pts',(-0.128270146612636,-0.581450425290948,
-0.165974498461211));
#40972=CARTESIAN_POINT('Ctrl Pts',(0.159119430707533,-0.573773118428659,
-0.155599026210492));
#40973=CARTESIAN_POINT('Ctrl Pts',(0.409415432322886,-0.432341853180699,
-0.145223553959774));
#40974=CARTESIAN_POINT('Ctrl Pts',(0.56426305151595,-0.190104706888137,
-0.134848081709056));
#40975=CARTESIAN_POINT('Ctrl Pts',(0.587571414135597,0.0964199572183358,
-0.124472609458338));
#40976=CARTESIAN_POINT('Ctrl Pts',(0.47389064191257,0.360530207813974,-0.114097137207619));
#40977=CARTESIAN_POINT('Ctrl Pts',(0.324463350889184,0.480464515819192,
-0.10718015570714));
#40978=CARTESIAN_POINT('Ctrl Pts',(0.240021988234213,0.519480035866726,
-0.103721664956901));
#40979=CARTESIAN_POINT('',(0.244165145742818,0.528447079373888,-0.12));
#40980=CARTESIAN_POINT('Ctrl Pts',(0.532924512516476,0.208474282488455,
-0.12));
#40981=CARTESIAN_POINT('Ctrl Pts',(0.505551419169843,0.278448344774197,
-0.12));
#40982=CARTESIAN_POINT('Ctrl Pts',(0.465349567486002,0.342411647567949,
-0.12));
#40983=CARTESIAN_POINT('Ctrl Pts',(0.351955928646152,0.46510551701231,-0.12));
#40984=CARTESIAN_POINT('Ctrl Pts',(0.287038107347888,0.504862695897963,
-0.12));
#40985=CARTESIAN_POINT('Ctrl Pts',(0.244165145742818,0.528447079373888,
-0.12));
#40986=CARTESIAN_POINT('Ctrl Pts',(-0.353365195478197,-0.462556454142148,
-0.72625));
#40987=CARTESIAN_POINT('Ctrl Pts',(-0.320950876724053,-0.487335965390693,
-0.724759130180554));
#40988=CARTESIAN_POINT('Ctrl Pts',(-0.204788602894649,-0.558391458988749,
-0.719809769610869));
#40989=CARTESIAN_POINT('Ctrl Pts',(0.0275428991067036,-0.605077845001504,
-0.711401918290945));
#40990=CARTESIAN_POINT('Ctrl Pts',(0.307852790782245,-0.521644157320061,
-0.701026446040225));
#40991=CARTESIAN_POINT('Ctrl Pts',(0.516379630382223,-0.316594299265632,
-0.690650973789508));
#40992=CARTESIAN_POINT('Ctrl Pts',(0.604531894922356,-0.037741447613471,
-0.680275501538789));
#40993=CARTESIAN_POINT('Ctrl Pts',(0.551748054568745,0.249911729814406,
-0.669900029288071));
#40994=CARTESIAN_POINT('Ctrl Pts',(0.370338916630071,0.479302937024635,
-0.659524557037353));
#40995=CARTESIAN_POINT('Ctrl Pts',(0.102593005245228,0.596956344106599,
-0.649149084786633));
#40996=CARTESIAN_POINT('Ctrl Pts',(-0.189069595066604,0.575443129800777,
-0.638773612535917));
#40997=CARTESIAN_POINT('Ctrl Pts',(-0.436655282749753,0.419778941359981,
-0.628398140285197));
#40998=CARTESIAN_POINT('Ctrl Pts',(-0.582444898128172,0.166253064936486,
-0.618022668034479));
#40999=CARTESIAN_POINT('Ctrl Pts',(-0.59245118529686,-0.126030790814807,
-0.607647195783762));
#41000=CARTESIAN_POINT('Ctrl Pts',(-0.464341322608817,-0.388933533934673,
-0.597271723533042));
#41001=CARTESIAN_POINT('Ctrl Pts',(-0.227981169867371,-0.561165524309829,
-0.586896251282325));
#41002=CARTESIAN_POINT('Ctrl Pts',(0.0615274613730338,-0.602574918002375,
-0.576520779031606));
#41003=CARTESIAN_POINT('Ctrl Pts',(0.336692401993215,-0.503508078945706,
-0.566145306780887));
#41004=CARTESIAN_POINT('Ctrl Pts',(0.533365395804019,-0.287060123544462,
-0.55576983453017));
#41005=CARTESIAN_POINT('Ctrl Pts',(0.605696737111815,-0.00369082231710978,
-0.545394362279451));
#41006=CARTESIAN_POINT('Ctrl Pts',(0.536824069047151,0.280538907457441,
-0.535018890028733));
#41007=CARTESIAN_POINT('Ctrl Pts',(0.342803440542624,0.499367560825895,
-0.524643417778015));
#41008=CARTESIAN_POINT('Ctrl Pts',(0.0688662178762295,0.601780361666548,
-0.514267945527296));
#41009=CARTESIAN_POINT('Ctrl Pts',(-0.221125550821607,0.563902163890325,
-0.503892473276578));
#41010=CARTESIAN_POINT('Ctrl Pts',(-0.459567075698392,0.394563382218786,
-0.493517001025859));
#41011=CARTESIAN_POINT('Ctrl Pts',(-0.590871299173015,0.133241387995481,
-0.483141528775141));
#41012=CARTESIAN_POINT('Ctrl Pts',(-0.584427716440101,-0.159142715555849,
-0.472766056524423));
#41013=CARTESIAN_POINT('Ctrl Pts',(-0.441738497928306,-0.414426421825547,
-0.462390584273705));
#41014=CARTESIAN_POINT('Ctrl Pts',(-0.196068293388198,-0.573096313010961,
-0.452015112022986));
#41015=CARTESIAN_POINT('Ctrl Pts',(0.0953106421677161,-0.598162219760071,
-0.441639639772268));
#41016=CARTESIAN_POINT('Ctrl Pts',(0.364470133516224,-0.483780612916302,
-0.43126416752155));
#41017=CARTESIAN_POINT('Ctrl Pts',(0.548661948506927,-0.256616885491388,
-0.420888695270832));
#41018=CARTESIAN_POINT('Ctrl Pts',(0.60494607893493,0.0303710592533639,
-0.410513223020113));
#41019=CARTESIAN_POINT('Ctrl Pts',(0.520201197869222,0.310278702773021,
-0.400137750769395));
#41020=CARTESIAN_POINT('Ctrl Pts',(0.314183589749731,0.517852132939369,
-0.389762278518676));
#41021=CARTESIAN_POINT('Ctrl Pts',(0.0349214353255983,0.604700465533282,
-0.379386806267958));
#41022=CARTESIAN_POINT('Ctrl Pts',(-0.252481833942362,0.550577045637576,
-0.36901133401724));
#41023=CARTESIAN_POINT('Ctrl Pts',(-0.481024876325774,0.368099481148946,
-0.358635861766521));
#41024=CARTESIAN_POINT('Ctrl Pts',(-0.597428233573601,0.0998081428603092,
-0.348260389515803));
#41025=CARTESIAN_POINT('Ctrl Pts',(-0.574555188931242,-0.191751126529284,
-0.337884917265085));
#41026=CARTESIAN_POINT('Ctrl Pts',(-0.417738057072088,-0.43860811139261,
-0.327509445014367));
#41027=CARTESIAN_POINT('Ctrl Pts',(-0.163535079971663,-0.583213886268098,
-0.317133972763648));
#41028=CARTESIAN_POINT('Ctrl Pts',(0.128792271407237,-0.591857001983,-0.30675850051293));
#41029=CARTESIAN_POINT('Ctrl Pts',(0.3910947206114,-0.462522516893444,-0.296383028262211));
#41030=CARTESIAN_POINT('Ctrl Pts',(0.562222594861329,-0.225361740621548,
-0.286007556011493));
#41031=CARTESIAN_POINT('Ctrl Pts',(0.602281436660628,0.0643368521302563,
-0.275632083760774));
#41032=CARTESIAN_POINT('Ctrl Pts',(0.501932467413927,0.339036806050298,
-0.265256611510057));
#41033=CARTESIAN_POINT('Ctrl Pts',(0.284569694815385,0.534698285003551,
-0.254881139259338));
#41034=CARTESIAN_POINT('Ctrl Pts',(0.00086616792234151,0.605707347412463,
-0.24450566700862));
#41035=CARTESIAN_POINT('Ctrl Pts',(-0.283039297466054,0.535509992112656,
-0.234130194757901));
#41036=CARTESIAN_POINT('Ctrl Pts',(-0.500960755684866,0.340470892555017,
-0.223754722507184));
#41037=CARTESIAN_POINT('Ctrl Pts',(-0.602094991516589,0.066059236182406,
-0.213379250256465));
#41038=CARTESIAN_POINT('Ctrl Pts',(-0.562864788572229,-0.223753096954469,
-0.203003778005747));
#41039=CARTESIAN_POINT('Ctrl Pts',(-0.392416023107415,-0.46140161814604,
-0.192628305755028));
#41040=CARTESIAN_POINT('Ctrl Pts',(-0.130484291345699,-0.591487175311845,
-0.18225283350431));
#41041=CARTESIAN_POINT('Ctrl Pts',(0.161866082666176,-0.583677346042729,
-0.171877361253592));
#41042=CARTESIAN_POINT('Ctrl Pts',(0.416482587440825,-0.439804754427654,
-0.161501889002873));
#41043=CARTESIAN_POINT('Ctrl Pts',(0.574003120398452,-0.193386213509922,
-0.151126416752155));
#41044=CARTESIAN_POINT('Ctrl Pts',(0.597713822063416,0.0980843175241036,
-0.140750944501437));
#41045=CARTESIAN_POINT('Ctrl Pts',(0.482070740684944,0.366753526971408,
-0.130375472250718));
#41046=CARTESIAN_POINT('Ctrl Pts',(0.33006409929725,0.48875809000787,-0.12345849075024));
#41047=CARTESIAN_POINT('Ctrl Pts',(0.244165145742818,0.528447079373888,
-0.12));
#41048=CARTESIAN_POINT('Ctrl Pts',(-0.389567997368774,-0.509945078027931,
-0.75727273924394));
#41049=CARTESIAN_POINT('Ctrl Pts',(-0.304713279680621,-0.574769083320626,
-0.753732335137029));
#41050=CARTESIAN_POINT('Ctrl Pts',(-0.102102228503407,-0.661170845788992,
-0.746651526923207));
#41051=CARTESIAN_POINT('Ctrl Pts',(0.226918975852293,-0.629330849807756,
-0.736030314602476));
#41052=CARTESIAN_POINT('Ctrl Pts',(0.500480649699589,-0.443915736617459,
-0.725409102281742));
#41053=CARTESIAN_POINT('Ctrl Pts',(0.651928335250053,-0.150143800232939,
-0.714787889961012));
#41054=CARTESIAN_POINT('Ctrl Pts',(0.644242880084047,0.180267689012914,
-0.704166677640277));
#41055=CARTESIAN_POINT('Ctrl Pts',(0.479327999531238,0.466684539337087,
-0.693545465319547));
#41056=CARTESIAN_POINT('Ctrl Pts',(0.197419996334723,0.639197400194773,
-0.682924252998813));
#41057=CARTESIAN_POINT('Ctrl Pts',(-0.13266944809657,0.655703641639384,
-0.672303040678082));
#41058=CARTESIAN_POINT('Ctrl Pts',(-0.430379781004106,0.512173537080057,
-0.661681828357348));
#41059=CARTESIAN_POINT('Ctrl Pts',(-0.623047772943777,0.243638675874784,
-0.651060616036617));
#41060=CARTESIAN_POINT('Ctrl Pts',(-0.663650324809919,-0.0843605725621005,
-0.640439403715884));
#41061=CARTESIAN_POINT('Ctrl Pts',(-0.542277215052327,-0.391770096128179,
-0.629818191395152));
#41062=CARTESIAN_POINT('Ctrl Pts',(-0.288551910996521,-0.603561275664924,
-0.61919697907442));
#41063=CARTESIAN_POINT('Ctrl Pts',(0.0355995897879127,-0.668042721572721,
-0.608575766753687));
#41064=CARTESIAN_POINT('Ctrl Pts',(0.351062366380979,-0.569476623116135,
-0.597954554432955));
#41065=CARTESIAN_POINT('Ctrl Pts',(0.580842221167565,-0.331919757495687,
-0.587333342112222));
#41066=CARTESIAN_POINT('Ctrl Pts',(0.668857333165026,-0.0133520513920273,
-0.57671212979149));
#41067=CARTESIAN_POINT('Ctrl Pts',(0.593626077081373,0.308474457943291,
-0.566090917470758));
#41068=CARTESIAN_POINT('Ctrl Pts',(0.373509957515226,0.555012361719922,
-0.555469705150025));
#41069=CARTESIAN_POINT('Ctrl Pts',(0.0622321783665508,0.666089758367902,
-0.544848492829294));
#41070=CARTESIAN_POINT('Ctrl Pts',(-0.264234456403739,0.614596259540999,
-0.53422728050856));
#41071=CARTESIAN_POINT('Ctrl Pts',(-0.526210034624122,0.413099757483066,
-0.523606068187829));
#41072=CARTESIAN_POINT('Ctrl Pts',(-0.659754819010986,0.110779009702939,
-0.512984855867096));
#41073=CARTESIAN_POINT('Ctrl Pts',(-0.632274861107494,-0.218579299549813,
-0.502363643546364));
#41074=CARTESIAN_POINT('Ctrl Pts',(-0.450477126973457,-0.494589494695984,
-0.491742431225631));
#41075=CARTESIAN_POINT('Ctrl Pts',(-0.158732544136138,-0.64988644363315,
-0.481121218904899));
#41076=CARTESIAN_POINT('Ctrl Pts',(0.171753501841992,-0.646567200522882,
-0.470500006584167));
#41077=CARTESIAN_POINT('Ctrl Pts',(0.460320091431361,-0.48544188489642,
-0.459878794263435));
#41078=CARTESIAN_POINT('Ctrl Pts',(0.636537484106821,-0.205835957776284,
-0.449257581942702));
#41079=CARTESIAN_POINT('Ctrl Pts',(0.657396732580188,0.124007847251966,
-0.43863636962197));
#41080=CARTESIAN_POINT('Ctrl Pts',(0.517806771181053,0.423585360825624,
-0.428015157301238));
#41081=CARTESIAN_POINT('Ctrl Pts',(0.251836979788509,0.619779433184232,
-0.417393944980505));
#41082=CARTESIAN_POINT('Ctrl Pts',(-0.0755980462515238,0.664705457770534,
-0.406772732659774));
#41083=CARTESIAN_POINT('Ctrl Pts',(-0.384582042358491,0.547398449834714,
-0.39615152033904));
#41084=CARTESIAN_POINT('Ctrl Pts',(-0.599702041634294,0.296489243396025,
-0.385530308018309));
#41085=CARTESIAN_POINT('Ctrl Pts',(-0.668454232892285,-0.0267833662666586,
-0.374909095697576));
#41086=CARTESIAN_POINT('Ctrl Pts',(-0.574058437290037,-0.343519025346637,
-0.364287883376844));
#41087=CARTESIAN_POINT('Ctrl Pts',(-0.339553605322675,-0.576412837542728,
-0.353666671056111));
#41088=CARTESIAN_POINT('Ctrl Pts',(-0.0221747569089046,-0.668622980721422,
-0.343045458735379));
#41089=CARTESIAN_POINT('Ctrl Pts',(0.300616230262104,-0.597643951136341,
-0.332424246414647));
#41090=CARTESIAN_POINT('Ctrl Pts',(0.550036550302552,-0.380799426675277,
-0.321803034093914));
#41091=CARTESIAN_POINT('Ctrl Pts',(0.665210797783139,-0.0710141190690022,
-0.311181821773182));
#41092=CARTESIAN_POINT('Ctrl Pts',(0.618028674331743,0.256103430490016,
-0.30056060945245));
#41093=CARTESIAN_POINT('Ctrl Pts',(0.420005809134218,0.520714443433612,
-0.289939397131717));
#41094=CARTESIAN_POINT('Ctrl Pts',(0.119473149966588,0.658235957542453,
-0.279318184810985));
#41095=CARTESIAN_POINT('Ctrl Pts',(-0.210219017943201,0.635103434988625,
-0.268696972490253));
#41096=CARTESIAN_POINT('Ctrl Pts',(-0.488603565549287,0.456962771519233,
-0.25807576016952));
#41097=CARTESIAN_POINT('Ctrl Pts',(-0.647735797590754,0.167292327094403,
-0.247454547848788));
#41098=CARTESIAN_POINT('Ctrl Pts',(-0.648776820735564,-0.163208751908622,
-0.236833335528056));
#41099=CARTESIAN_POINT('Ctrl Pts',(-0.491472315475939,-0.453875858438117,
-0.226212123207324));
#41100=CARTESIAN_POINT('Ctrl Pts',(-0.214215682544731,-0.633766620558494,
-0.215590910886591));
#41101=CARTESIAN_POINT('Ctrl Pts',(0.115324674990204,-0.658975468022751,
-0.204969698565859));
#41102=CARTESIAN_POINT('Ctrl Pts',(0.416716775328578,-0.523349883470236,
-0.194348486245126));
#41103=CARTESIAN_POINT('Ctrl Pts',(0.616404307509721,-0.259991384615625,
-0.183727273924394));
#41104=CARTESIAN_POINT('Ctrl Pts',(0.66564263859121,0.0668221963899351,
-0.173106061603661));
#41105=CARTESIAN_POINT('Ctrl Pts',(0.552428954539379,0.377327397940862,
-0.162484849282929));
#41106=CARTESIAN_POINT('Ctrl Pts',(0.304365909285143,0.595737740289611,
-0.151863636962197));
#41107=CARTESIAN_POINT('Ctrl Pts',(-0.0179442774568819,0.668750733104762,
-0.141242424641465));
#41108=CARTESIAN_POINT('Ctrl Pts',(-0.33595438712131,0.578538159640864,
-0.130621212320732));
#41109=CARTESIAN_POINT('Ctrl Pts',(-0.493165134596604,0.424261513660227,
-0.123540404106911));
#41110=CARTESIAN_POINT('Ctrl Pts',(-0.548572772984126,0.332979158385831,
-0.12));
#41111=CARTESIAN_POINT('Ctrl Pts',(-0.377508796945348,-0.494159567045475,
-0.746931826162627));
#41112=CARTESIAN_POINT('Ctrl Pts',(-0.295280783848913,-0.556976924776374,
-0.743391422055716));
#41113=CARTESIAN_POINT('Ctrl Pts',(-0.0989416217658999,-0.640704093393138,
-0.736310613841894));
#41114=CARTESIAN_POINT('Ctrl Pts',(0.219894627270879,-0.609849714545784,
-0.725689401521162));
#41115=CARTESIAN_POINT('Ctrl Pts',(0.484988113085858,-0.430174184757091,
-0.71506818920043));
#41116=CARTESIAN_POINT('Ctrl Pts',(0.631747687687648,-0.145496051466169,
-0.704446976879697));
#41117=CARTESIAN_POINT('Ctrl Pts',(0.62430013821415,0.174687445752796,-0.693825764558965));
#41118=CARTESIAN_POINT('Ctrl Pts',(0.464490249885608,0.452238171995848,
-0.683204552238233));
#41119=CARTESIAN_POINT('Ctrl Pts',(0.191308797983031,0.619410842748719,
-0.672583339917501));
#41120=CARTESIAN_POINT('Ctrl Pts',(-0.128562623420344,0.635406128275076,
-0.661962127596767));
#41121=CARTESIAN_POINT('Ctrl Pts',(-0.41705723892577,0.49631904344367,-0.651340915276036));
#41122=CARTESIAN_POINT('Ctrl Pts',(-0.603761132310959,0.236096763697407,
-0.640719702955302));
#41123=CARTESIAN_POINT('Ctrl Pts',(-0.643106819357702,-0.0817491643888608,
-0.630098490634572));
#41124=CARTESIAN_POINT('Ctrl Pts',(-0.52549085255453,-0.379642729042011,
-0.619477278313838));
#41125=CARTESIAN_POINT('Ctrl Pts',(-0.279619695437819,-0.584877845711175,
-0.608856065993107));
#41126=CARTESIAN_POINT('Ctrl Pts',(0.0344975932400858,-0.647363248091151,
-0.598234853672374));
#41127=CARTESIAN_POINT('Ctrl Pts',(0.340195119928743,-0.551848294349405,
-0.587613641351642));
#41128=CARTESIAN_POINT('Ctrl Pts',(0.562862066722751,-0.321645076548663,
-0.576992429030909));
#41129=CARTESIAN_POINT('Ctrl Pts',(0.648152643124277,-0.0129387344232621,
-0.566371216710177));
#41130=CARTESIAN_POINT('Ctrl Pts',(0.575250194338317,0.298925533650301,
-0.555750004389445));
#41131=CARTESIAN_POINT('Ctrl Pts',(0.361947838788215,0.537831778733985,
-0.545128792068713));
#41132=CARTESIAN_POINT('Ctrl Pts',(0.0603057616260149,0.645470739479278,
-0.53450757974798));
#41133=CARTESIAN_POINT('Ctrl Pts',(-0.256054995333863,0.595571238175405,
-0.523886367427248));
#41134=CARTESIAN_POINT('Ctrl Pts',(-0.509921036772116,0.400312123991598,
-0.513265155106515));
#41135=CARTESIAN_POINT('Ctrl Pts',(-0.63933190017137,0.107349810462397,
-0.502643942785783));
#41136=CARTESIAN_POINT('Ctrl Pts',(-0.612702593045721,-0.211813108282854,
-0.49202273046505));
#41137=CARTESIAN_POINT('Ctrl Pts',(-0.436532465201871,-0.47927932064641,
-0.481401518144319));
#41138=CARTESIAN_POINT('Ctrl Pts',(-0.153818928088652,-0.629769003470783,
-0.470780305823586));
#41139=CARTESIAN_POINT('Ctrl Pts',(0.16643681793539,-0.626552508579544,
-0.460159093502854));
#41140=CARTESIAN_POINT('Ctrl Pts',(0.446070737585578,-0.47041487799793,
-0.449537881182121));
#41141=CARTESIAN_POINT('Ctrl Pts',(0.61683326520354,-0.199464240679558,
-0.438916668861389));
#41142=CARTESIAN_POINT('Ctrl Pts',(0.637046809050958,0.120169145166092,
-0.428295456540657));
#41143=CARTESIAN_POINT('Ctrl Pts',(0.501777899003527,0.410473142170276,
-0.417674244219924));
#41144=CARTESIAN_POINT('Ctrl Pts',(0.244041286523631,0.600593965041143,
-0.407053031899192));
#41145=CARTESIAN_POINT('Ctrl Pts',(-0.0732578848483181,0.644129290344205,
-0.396431819578459));
#41146=CARTESIAN_POINT('Ctrl Pts',(-0.372677183747475,0.530453557896425,
-0.385810607257728));
#41147=CARTESIAN_POINT('Ctrl Pts',(-0.581138075489099,0.287311325205486,
-0.375189394936995));
#41148=CARTESIAN_POINT('Ctrl Pts',(-0.64776202094782,-0.0259542787029844,
-0.364568182616263));
#41149=CARTESIAN_POINT('Ctrl Pts',(-0.556288277018155,-0.332885285399068,
-0.35394697029553));
#41150=CARTESIAN_POINT('Ctrl Pts',(-0.329042616204627,-0.558569796067267,
-0.343325757974798));
#41151=CARTESIAN_POINT('Ctrl Pts',(-0.0214883303037647,-0.647925545134599,
-0.332704545654066));
#41152=CARTESIAN_POINT('Ctrl Pts',(0.291310559889408,-0.579143693832662,
-0.322083333333334));
#41153=CARTESIAN_POINT('Ctrl Pts',(0.533009995130902,-0.369011660127668,
-0.311462121012601));
#41154=CARTESIAN_POINT('Ctrl Pts',(0.644618987397083,-0.0688158545797981,
-0.300840908691869));
#41155=CARTESIAN_POINT('Ctrl Pts',(0.598897401481997,0.248175667895896,
-0.290219696371136));
#41156=CARTESIAN_POINT('Ctrl Pts',(0.407004396632262,0.504595563342971,
-0.279598484050404));
#41157=CARTESIAN_POINT('Ctrl Pts',(0.115774820867698,0.637860055539404,
-0.268977271729672));
#41158=CARTESIAN_POINT('Ctrl Pts',(-0.203711621834396,0.615443607528816,
-0.258356059408939));
#41159=CARTESIAN_POINT('Ctrl Pts',(-0.473478687827409,0.442817344571911,
-0.247734847088207));
#41160=CARTESIAN_POINT('Ctrl Pts',(-0.62768493135602,0.162113740261402,
-0.237113634767475));
#41161=CARTESIAN_POINT('Ctrl Pts',(-0.628693729300522,-0.158156573435501,
-0.226492422446742));
#41162=CARTESIAN_POINT('Ctrl Pts',(-0.476258634693842,-0.439825987860379,
-0.215871210126011));
#41163=CARTESIAN_POINT('Ctrl Pts',(-0.207584568420635,-0.614148174611669,
-0.205249997805277));
#41164=CARTESIAN_POINT('Ctrl Pts',(0.111754763244715,-0.638576674239172,
-0.194628785484546));
#41165=CARTESIAN_POINT('Ctrl Pts',(0.403817175907084,-0.507149422500723,
-0.184007573163813));
#41166=CARTESIAN_POINT('Ctrl Pts',(0.59732331744809,-0.251943269173339,
-0.173386360843081));
#41167=CARTESIAN_POINT('Ctrl Pts',(0.645037460436522,0.0647536941914932,
-0.162765148522348));
#41168=CARTESIAN_POINT('Ctrl Pts',(0.535328341738816,0.365647109139544,
-0.152143936201616));
#41169=CARTESIAN_POINT('Ctrl Pts',(0.294944166413762,0.577296490344866,
-0.141522723880883));
#41170=CARTESIAN_POINT('Ctrl Pts',(-0.0173888066795909,0.648049342902555,
-0.130901511560152));
#41171=CARTESIAN_POINT('Ctrl Pts',(-0.325554812939681,0.560629328148464,
-0.120280299239419));
#41172=CARTESIAN_POINT('Ctrl Pts',(-0.477899052063863,0.411128364480287,
-0.113199491025598));
#41173=CARTESIAN_POINT('Ctrl Pts',(-0.531591529501778,0.322671683349587,
-0.109659086918687));
#41174=CARTESIAN_POINT('Ctrl Pts',(-0.365449596521923,-0.478374056063018,
-0.736590913081313));
#41175=CARTESIAN_POINT('Ctrl Pts',(-0.285848288017205,-0.539184766232121,
-0.733050508974403));
#41176=CARTESIAN_POINT('Ctrl Pts',(-0.0957810150283928,-0.620237340997284,
-0.72596970076058));
#41177=CARTESIAN_POINT('Ctrl Pts',(0.212870278689466,-0.590368579283812,
-0.715348488439849));
#41178=CARTESIAN_POINT('Ctrl Pts',(0.469495576472127,-0.416432632896724,
-0.704727276119116));
#41179=CARTESIAN_POINT('Ctrl Pts',(0.611567040125244,-0.140848302699399,
-0.694106063798384));
#41180=CARTESIAN_POINT('Ctrl Pts',(0.604357396344252,0.169107202492678,
-0.683484851477651));
#41181=CARTESIAN_POINT('Ctrl Pts',(0.44965250023998,0.437791804654609,-0.67286363915692));
#41182=CARTESIAN_POINT('Ctrl Pts',(0.185197599631338,0.599624285302665,
-0.662242426836187));
#41183=CARTESIAN_POINT('Ctrl Pts',(-0.124455798744119,0.615108614910768,
-0.651621214515455));
#41184=CARTESIAN_POINT('Ctrl Pts',(-0.403734696847433,0.480464549807283,
-0.641000002194722));
#41185=CARTESIAN_POINT('Ctrl Pts',(-0.584474491678141,0.22855485152003,
-0.630378789873991));
#41186=CARTESIAN_POINT('Ctrl Pts',(-0.622563313905486,-0.0791377562156208,
-0.619757577553257));
#41187=CARTESIAN_POINT('Ctrl Pts',(-0.508704490056733,-0.367515361955843,
-0.609136365232526));
#41188=CARTESIAN_POINT('Ctrl Pts',(-0.270687479879118,-0.566194415757424,
-0.598515152911792));
#41189=CARTESIAN_POINT('Ctrl Pts',(0.033395596692259,-0.62668377460958,
-0.587893940591062));
#41190=CARTESIAN_POINT('Ctrl Pts',(0.329327873476507,-0.534219965582675,
-0.577272728270328));
#41191=CARTESIAN_POINT('Ctrl Pts',(0.544881912277937,-0.311370395601639,
-0.566651515949596));
#41192=CARTESIAN_POINT('Ctrl Pts',(0.627447953083531,-0.0125254174544974,
-0.556030303628864));
#41193=CARTESIAN_POINT('Ctrl Pts',(0.556874311595259,0.289376609357312,
-0.545409091308131));
#41194=CARTESIAN_POINT('Ctrl Pts',(0.350385720061206,0.520651195748048,
-0.5347878789874));
#41195=CARTESIAN_POINT('Ctrl Pts',(0.0583793448854777,0.624851720590656,
-0.524166666666666));
#41196=CARTESIAN_POINT('Ctrl Pts',(-0.247875534263986,0.576546216809811,
-0.513545454345935));
#41197=CARTESIAN_POINT('Ctrl Pts',(-0.49363203892011,0.387524490500131,
-0.502924242025201));
#41198=CARTESIAN_POINT('Ctrl Pts',(-0.618908981331752,0.103920611221856,
-0.49230302970447));
#41199=CARTESIAN_POINT('Ctrl Pts',(-0.593130324983951,-0.205046917015896,
-0.481681817383737));
#41200=CARTESIAN_POINT('Ctrl Pts',(-0.422587803430283,-0.463969146596836,
-0.471060605063006));
#41201=CARTESIAN_POINT('Ctrl Pts',(-0.148905312041167,-0.609651563308416,
-0.460439392742272));
#41202=CARTESIAN_POINT('Ctrl Pts',(0.161120134028788,-0.606537816636207,
-0.449818180421541));
#41203=CARTESIAN_POINT('Ctrl Pts',(0.431821383739795,-0.455387871099441,
-0.439196968100808));
#41204=CARTESIAN_POINT('Ctrl Pts',(0.597129046300259,-0.193092523582832,
-0.428575755780076));
#41205=CARTESIAN_POINT('Ctrl Pts',(0.616696885521728,0.116330443080218,
-0.417954543459344));
#41206=CARTESIAN_POINT('Ctrl Pts',(0.485749026826,0.397360923514928,-0.407333331138611));
#41207=CARTESIAN_POINT('Ctrl Pts',(0.236245593258753,0.581408496898052,
-0.396712118817879));
#41208=CARTESIAN_POINT('Ctrl Pts',(-0.0709177234451122,0.623553122917875,
-0.386090906497146));
#41209=CARTESIAN_POINT('Ctrl Pts',(-0.36077232513646,0.513508665958136,
-0.375469694176414));
#41210=CARTESIAN_POINT('Ctrl Pts',(-0.562574109343903,0.278133407014948,
-0.364848481855682));
#41211=CARTESIAN_POINT('Ctrl Pts',(-0.627069809003355,-0.0251251911393111,
-0.35422726953495));
#41212=CARTESIAN_POINT('Ctrl Pts',(-0.538518116746273,-0.322251545451498,
-0.343606057214217));
#41213=CARTESIAN_POINT('Ctrl Pts',(-0.31853162708658,-0.540726754591806,
-0.332984844893485));
#41214=CARTESIAN_POINT('Ctrl Pts',(-0.0208019036986243,-0.627228109547775,
-0.322363632572752));
#41215=CARTESIAN_POINT('Ctrl Pts',(0.28200488951671,-0.560643436528983,
-0.311742420252021));
#41216=CARTESIAN_POINT('Ctrl Pts',(0.515983439959253,-0.357223893580059,
-0.301121207931288));
#41217=CARTESIAN_POINT('Ctrl Pts',(0.624027177011026,-0.0666175900905945,
-0.290499995610556));
#41218=CARTESIAN_POINT('Ctrl Pts',(0.579766128632252,0.240247905301778,
-0.279878783289823));
#41219=CARTESIAN_POINT('Ctrl Pts',(0.394002984130306,0.488476683252329,
-0.269257570969091));
#41220=CARTESIAN_POINT('Ctrl Pts',(0.112076491768808,0.617484153536356,
-0.258636358648359));
#41221=CARTESIAN_POINT('Ctrl Pts',(-0.197204225725589,0.595783780069004,
-0.248015146327626));
#41222=CARTESIAN_POINT('Ctrl Pts',(-0.458353810105532,0.428671917624589,
-0.237393934006894));
#41223=CARTESIAN_POINT('Ctrl Pts',(-0.607634065121286,0.1569351534284,-0.226772721686162));
#41224=CARTESIAN_POINT('Ctrl Pts',(-0.608610637865481,-0.15310439496238,
-0.216151509365429));
#41225=CARTESIAN_POINT('Ctrl Pts',(-0.461044953911745,-0.425776117282641,
-0.205530297044697));
#41226=CARTESIAN_POINT('Ctrl Pts',(-0.200953454296539,-0.594529728664845,
-0.194909084723964));
#41227=CARTESIAN_POINT('Ctrl Pts',(0.108184851499226,-0.618177880455594,
-0.184287872403232));
#41228=CARTESIAN_POINT('Ctrl Pts',(0.390917576485589,-0.490948961531211,
-0.1736666600825));
#41229=CARTESIAN_POINT('Ctrl Pts',(0.57824232738646,-0.243895153731054,
-0.163045447761767));
#41230=CARTESIAN_POINT('Ctrl Pts',(0.624432282281831,0.0626851919930514,
-0.152424235441035));
#41231=CARTESIAN_POINT('Ctrl Pts',(0.518227728938254,0.353966820338225,
-0.141803023120303));
#41232=CARTESIAN_POINT('Ctrl Pts',(0.28552242354238,0.558855240400121,-0.13118181079957));
#41233=CARTESIAN_POINT('Ctrl Pts',(-0.0168333359022998,0.627347952700348,
-0.120560598478838));
#41234=CARTESIAN_POINT('Ctrl Pts',(-0.315155238758052,0.542720496656064,
-0.109939386158106));
#41235=CARTESIAN_POINT('Ctrl Pts',(-0.462632969531122,0.397995215300347,
-0.102858577944284));
#41236=CARTESIAN_POINT('Ctrl Pts',(-0.514610286019429,0.312364208313342,
-0.0993181738373735));
#41237=CARTESIAN_POINT('Ctrl Pts',(-0.353390396098497,-0.462588545080562,
-0.72625));
#41238=CARTESIAN_POINT('Ctrl Pts',(-0.276415792185496,-0.521392607687868,
-0.722709595893089));
#41239=CARTESIAN_POINT('Ctrl Pts',(-0.0926204082908857,-0.59977058860143,
-0.715628787679267));
#41240=CARTESIAN_POINT('Ctrl Pts',(0.205845930108053,-0.57088744402184,
-0.705007575358536));
#41241=CARTESIAN_POINT('Ctrl Pts',(0.454003039858395,-0.402691081036356,
-0.694386363037803));
#41242=CARTESIAN_POINT('Ctrl Pts',(0.59138639256284,-0.136200553932629,
-0.683765150717071));
#41243=CARTESIAN_POINT('Ctrl Pts',(0.584414654474354,0.16352695923256,-0.673143938396339));
#41244=CARTESIAN_POINT('Ctrl Pts',(0.434814750594351,0.42334543731337,-0.662522726075606));
#41245=CARTESIAN_POINT('Ctrl Pts',(0.179086401279645,0.57983772785661,-0.651901513754874));
#41246=CARTESIAN_POINT('Ctrl Pts',(-0.120348974067893,0.59481110154646,
-0.641280301434141));
#41247=CARTESIAN_POINT('Ctrl Pts',(-0.390412154769097,0.464610056170896,
-0.630659089113409));
#41248=CARTESIAN_POINT('Ctrl Pts',(-0.565187851045323,0.221012939342653,
-0.620037876792677));
#41249=CARTESIAN_POINT('Ctrl Pts',(-0.602019808453269,-0.0765263480423816,
-0.609416664471945));
#41250=CARTESIAN_POINT('Ctrl Pts',(-0.491918127558936,-0.355387994869674,
-0.598795452151212));
#41251=CARTESIAN_POINT('Ctrl Pts',(-0.261755264320416,-0.547510985803676,
-0.58817423983048));
#41252=CARTESIAN_POINT('Ctrl Pts',(0.0322936001444312,-0.606004301128008,
-0.577553027509747));
#41253=CARTESIAN_POINT('Ctrl Pts',(0.318460627024272,-0.516591636815947,
-0.566931815189015));
#41254=CARTESIAN_POINT('Ctrl Pts',(0.526901757833122,-0.301095714654614,
-0.556310602868283));
#41255=CARTESIAN_POINT('Ctrl Pts',(0.606743263042784,-0.012112100485733,
-0.545689390547551));
#41256=CARTESIAN_POINT('Ctrl Pts',(0.538498428852201,0.279827685064323,
-0.535068178226818));
#41257=CARTESIAN_POINT('Ctrl Pts',(0.338823601334196,0.50347061276211,-0.524446965906085));
#41258=CARTESIAN_POINT('Ctrl Pts',(0.056452928144941,0.604232701702033,
-0.513825753585354));
#41259=CARTESIAN_POINT('Ctrl Pts',(-0.239696073194109,0.557521195444216,
-0.503204541264621));
#41260=CARTESIAN_POINT('Ctrl Pts',(-0.477343041068104,0.374736857008664,
-0.492583328943889));
#41261=CARTESIAN_POINT('Ctrl Pts',(-0.598486062492136,0.100491411981314,
-0.481962116623157));
#41262=CARTESIAN_POINT('Ctrl Pts',(-0.57355805692218,-0.198280725748937,
-0.471340904302424));
#41263=CARTESIAN_POINT('Ctrl Pts',(-0.408643141658697,-0.448658972547262,
-0.460719691981692));
#41264=CARTESIAN_POINT('Ctrl Pts',(-0.143991695993682,-0.589534123146049,
-0.45009847966096));
#41265=CARTESIAN_POINT('Ctrl Pts',(0.155803450122185,-0.58652312469287,
-0.439477267340227));
#41266=CARTESIAN_POINT('Ctrl Pts',(0.417572029894014,-0.440360864200951,
-0.428856055019495));
#41267=CARTESIAN_POINT('Ctrl Pts',(0.577424827396976,-0.186720806486106,
-0.418234842698762));
#41268=CARTESIAN_POINT('Ctrl Pts',(0.596346961992498,0.112491740994345,
-0.407613630378031));
#41269=CARTESIAN_POINT('Ctrl Pts',(0.469720154648472,0.38424870485958,-0.396992418057298));
#41270=CARTESIAN_POINT('Ctrl Pts',(0.228449899993875,0.562223028754963,
-0.386371205736566));
#41271=CARTESIAN_POINT('Ctrl Pts',(-0.0685775620419064,0.602976955491545,
-0.375749993415833));
#41272=CARTESIAN_POINT('Ctrl Pts',(-0.348867466525445,0.496563774019848,
-0.365128781095101));
#41273=CARTESIAN_POINT('Ctrl Pts',(-0.544010143198707,0.268955488824409,
-0.354507568774369));
#41274=CARTESIAN_POINT('Ctrl Pts',(-0.606377597058891,-0.0242961035756373,
-0.343886356453636));
#41275=CARTESIAN_POINT('Ctrl Pts',(-0.520747956474391,-0.311617805503928,
-0.333265144132904));
#41276=CARTESIAN_POINT('Ctrl Pts',(-0.308020637968532,-0.522883713116344,
-0.322643931812172));
#41277=CARTESIAN_POINT('Ctrl Pts',(-0.0201154770934842,-0.606530673960952,
-0.312022719491439));
#41278=CARTESIAN_POINT('Ctrl Pts',(0.272699219144013,-0.542143179225304,
-0.301401507170707));
#41279=CARTESIAN_POINT('Ctrl Pts',(0.498956884787604,-0.34543612703245,
-0.290780294849974));
#41280=CARTESIAN_POINT('Ctrl Pts',(0.603435366624969,-0.0644193256013902,
-0.280159082529242));
#41281=CARTESIAN_POINT('Ctrl Pts',(0.560634855782508,0.232320142707658,
-0.26953787020851));
#41282=CARTESIAN_POINT('Ctrl Pts',(0.381001571628349,0.472357803161688,
-0.258916657887777));
#41283=CARTESIAN_POINT('Ctrl Pts',(0.108378162669919,0.597108251533307,
-0.248295445567045));
#41284=CARTESIAN_POINT('Ctrl Pts',(-0.190696829616783,0.576123952609194,
-0.237674233246313));
#41285=CARTESIAN_POINT('Ctrl Pts',(-0.443228932383655,0.414526490677267,
-0.227053020925581));
#41286=CARTESIAN_POINT('Ctrl Pts',(-0.587583198886552,0.151756566595399,
-0.216431808604848));
#41287=CARTESIAN_POINT('Ctrl Pts',(-0.588527546430439,-0.148052216489259,
-0.205810596284116));
#41288=CARTESIAN_POINT('Ctrl Pts',(-0.445831273129648,-0.411726246704904,
-0.195189383963384));
#41289=CARTESIAN_POINT('Ctrl Pts',(-0.194322340172443,-0.574911282718019,
-0.184568171642651));
#41290=CARTESIAN_POINT('Ctrl Pts',(0.104614939753737,-0.597779086672016,
-0.173946959321919));
#41291=CARTESIAN_POINT('Ctrl Pts',(0.378017977064095,-0.474748500561697,
-0.163325747001186));
#41292=CARTESIAN_POINT('Ctrl Pts',(0.55916133732483,-0.235847038288769,
-0.152704534680454));
#41293=CARTESIAN_POINT('Ctrl Pts',(0.603827104127141,0.0606166897946097,
-0.142083322359722));
#41294=CARTESIAN_POINT('Ctrl Pts',(0.501127116137692,0.342286531536906,
-0.13146211003899));
#41295=CARTESIAN_POINT('Ctrl Pts',(0.276100680670998,0.540413990455376,
-0.120840897718257));
#41296=CARTESIAN_POINT('Ctrl Pts',(-0.0162778651250086,0.606646562498142,
-0.110219685397525));
#41297=CARTESIAN_POINT('Ctrl Pts',(-0.304755664576424,0.524811665163664,
-0.0995984730767926));
#41298=CARTESIAN_POINT('Ctrl Pts',(-0.447366886998382,0.384862066120406,
-0.092517664862971));
#41299=CARTESIAN_POINT('Ctrl Pts',(-0.49762904253708,0.302056733277098,
-0.0889772607560603));
#41300=CARTESIAN_POINT('',(-0.548572772984126,0.332979158385831,-0.12));
#41301=CARTESIAN_POINT('Ctrl Pts',(0.244188262120089,0.528481699529947,
-0.12));
#41302=CARTESIAN_POINT('Ctrl Pts',(0.218445435093476,0.542622181160769,
-0.12));
#41303=CARTESIAN_POINT('Ctrl Pts',(0.191707940815084,0.554740156615991,
-0.12));
#41304=CARTESIAN_POINT('Ctrl Pts',(0.164242712890297,0.56481938294899,-0.12));
#41305=CARTESIAN_POINT('Ctrl Pts',(0.135399059471504,0.575404465726192,
-0.12));
#41306=CARTESIAN_POINT('Ctrl Pts',(0.105751683718357,0.583741941385187,
-0.12));
#41307=CARTESIAN_POINT('Ctrl Pts',(0.0755747762095856,0.589763858499476,
-0.12));
#41308=CARTESIAN_POINT('Ctrl Pts',(0.0608331404233321,0.592705608206865,
-0.12));
#41309=CARTESIAN_POINT('Ctrl Pts',(0.0459647294330388,0.595093961778282,
-0.12));
#41310=CARTESIAN_POINT('Ctrl Pts',(0.0310000226320474,0.596915993675276,
-0.12));
#41311=CARTESIAN_POINT('Ctrl Pts',(0.0251721580287127,0.597625566895777,
-0.12));
#41312=CARTESIAN_POINT('Ctrl Pts',(0.0193318047130446,0.598248864029065,
-0.12));
#41313=CARTESIAN_POINT('Ctrl Pts',(0.0134897283974255,0.598784612282793,
-0.12));
#41314=CARTESIAN_POINT('Ctrl Pts',(0.00362475613712504,0.599689280653419,
-0.12));
#41315=CARTESIAN_POINT('Ctrl Pts',(-0.00625226620039982,0.600345248614976,
-0.12));
#41316=CARTESIAN_POINT('Ctrl Pts',(-0.0161321161443918,0.600751319652268,
-0.12));
#41317=CARTESIAN_POINT('Ctrl Pts',(-0.0462082784714154,0.60198747794446,
-0.12));
#41318=CARTESIAN_POINT('Ctrl Pts',(-0.0763096986544558,0.600911821118615,
-0.12));
#41319=CARTESIAN_POINT('Ctrl Pts',(-0.10619074537105,0.597625116816541,
-0.12));
#41320=CARTESIAN_POINT('Ctrl Pts',(-0.126342040119356,0.595408616579124,
-0.12));
#41321=CARTESIAN_POINT('Ctrl Pts',(-0.146393540566889,0.592185434384527,
-0.12));
#41322=CARTESIAN_POINT('Ctrl Pts',(-0.166271047885959,0.587973203665797,
-0.12));
#41323=CARTESIAN_POINT('Ctrl Pts',(-0.177982331622319,0.585491472515194,
-0.12));
#41324=CARTESIAN_POINT('Ctrl Pts',(-0.189633215255517,0.582666219304311,
-0.12));
#41325=CARTESIAN_POINT('Ctrl Pts',(-0.201208227469216,0.579499366783346,
-0.12));
#41326=CARTESIAN_POINT('Ctrl Pts',(-0.207704857075218,0.577721928672205,
-0.12));
#41327=CARTESIAN_POINT('Ctrl Pts',(-0.214175648256732,0.575837255539024,
-0.12));
#41328=CARTESIAN_POINT('Ctrl Pts',(-0.220606829957527,0.573849512326344,
-0.12));
#41329=CARTESIAN_POINT('Ctrl Pts',(-0.25015216366532,0.56471767011191,-0.12));
#41330=CARTESIAN_POINT('Ctrl Pts',(-0.278927093165708,0.553397185268195,
-0.12));
#41331=CARTESIAN_POINT('Ctrl Pts',(-0.30667747358036,0.539970478586301,
-0.12));
#41332=CARTESIAN_POINT('Ctrl Pts',(-0.30845905545231,0.53910848041305,-0.12));
#41333=CARTESIAN_POINT('Ctrl Pts',(-0.310236412641107,0.538237783373462,
-0.12));
#41334=CARTESIAN_POINT('Ctrl Pts',(-0.312009476799349,0.537358402041895,
-0.12));
#41335=CARTESIAN_POINT('Ctrl Pts',(-0.335549088486224,0.525683531184262,
-0.12));
#41336=CARTESIAN_POINT('Ctrl Pts',(-0.358332961769366,0.512480115942743,
-0.12));
#41337=CARTESIAN_POINT('Ctrl Pts',(-0.380250615167753,0.497858544366281,
-0.12));
#41338=CARTESIAN_POINT('Ctrl Pts',(-0.386498225486996,0.493690676583894,
-0.12));
#41339=CARTESIAN_POINT('Ctrl Pts',(-0.392677270141369,0.489406051262931,
-0.12));
#41340=CARTESIAN_POINT('Ctrl Pts',(-0.398778867975252,0.485011296272449,
-0.12));
#41341=CARTESIAN_POINT('Ctrl Pts',(-0.424115404323213,0.46676232729937,
-0.12));
#41342=CARTESIAN_POINT('Ctrl Pts',(-0.44802782182311,0.446685130200945,
-0.12));
#41343=CARTESIAN_POINT('Ctrl Pts',(-0.470348776553481,0.424986510597564,
-0.12));
#41344=CARTESIAN_POINT('Ctrl Pts',(-0.492791511018824,0.403169506625034,
-0.12));
#41345=CARTESIAN_POINT('Ctrl Pts',(-0.513626430101255,0.379712592792303,
-0.12));
#41346=CARTESIAN_POINT('Ctrl Pts',(-0.53265652290141,0.354781937742959,
-0.12));
#41347=CARTESIAN_POINT('Ctrl Pts',(-0.538112251162996,0.347634580094158,
-0.12));
#41348=CARTESIAN_POINT('Ctrl Pts',(-0.54341941474828,0.340365857942668,
-0.12));
#41349=CARTESIAN_POINT('Ctrl Pts',(-0.548572772984126,0.332979158385831,
-0.12));
#41350=CARTESIAN_POINT('Ctrl Pts',(0.462926795561193,-0.444481916564912,
-0.72625));
#41351=CARTESIAN_POINT('Ctrl Pts',(0.468784532279406,-0.438389058883916,
-0.725969700760581));
#41352=CARTESIAN_POINT('Ctrl Pts',(0.546966429469725,-0.353744549862236,
-0.722148997414251));
#41353=CARTESIAN_POINT('Ctrl Pts',(0.651928335250053,-0.150143800232939,
-0.714787889961012));
#41354=CARTESIAN_POINT('Ctrl Pts',(0.644242880084047,0.180267689012914,
-0.704166677640277));
#41355=CARTESIAN_POINT('Ctrl Pts',(0.479327999531238,0.466684539337087,
-0.693545465319547));
#41356=CARTESIAN_POINT('Ctrl Pts',(0.197419996334723,0.639197400194773,
-0.682924252998813));
#41357=CARTESIAN_POINT('Ctrl Pts',(-0.13266944809657,0.655703641639384,
-0.672303040678082));
#41358=CARTESIAN_POINT('Ctrl Pts',(-0.430379781004106,0.512173537080057,
-0.661681828357348));
#41359=CARTESIAN_POINT('Ctrl Pts',(-0.623047772943777,0.243638675874784,
-0.651060616036617));
#41360=CARTESIAN_POINT('Ctrl Pts',(-0.663650324809919,-0.0843605725621005,
-0.640439403715884));
#41361=CARTESIAN_POINT('Ctrl Pts',(-0.542277215052327,-0.391770096128179,
-0.629818191395152));
#41362=CARTESIAN_POINT('Ctrl Pts',(-0.288551910996521,-0.603561275664924,
-0.61919697907442));
#41363=CARTESIAN_POINT('Ctrl Pts',(0.0355995897879127,-0.668042721572721,
-0.608575766753687));
#41364=CARTESIAN_POINT('Ctrl Pts',(0.351062366380979,-0.569476623116135,
-0.597954554432955));
#41365=CARTESIAN_POINT('Ctrl Pts',(0.580842221167565,-0.331919757495687,
-0.587333342112222));
#41366=CARTESIAN_POINT('Ctrl Pts',(0.668857333165026,-0.0133520513920273,
-0.57671212979149));
#41367=CARTESIAN_POINT('Ctrl Pts',(0.593626077081373,0.308474457943291,
-0.566090917470758));
#41368=CARTESIAN_POINT('Ctrl Pts',(0.373509957515226,0.555012361719922,
-0.555469705150025));
#41369=CARTESIAN_POINT('Ctrl Pts',(0.0622321783665508,0.666089758367902,
-0.544848492829294));
#41370=CARTESIAN_POINT('Ctrl Pts',(-0.264234456403739,0.614596259540999,
-0.53422728050856));
#41371=CARTESIAN_POINT('Ctrl Pts',(-0.526210034624122,0.413099757483066,
-0.523606068187829));
#41372=CARTESIAN_POINT('Ctrl Pts',(-0.659754819010986,0.110779009702939,
-0.512984855867096));
#41373=CARTESIAN_POINT('Ctrl Pts',(-0.632274861107494,-0.218579299549813,
-0.502363643546364));
#41374=CARTESIAN_POINT('Ctrl Pts',(-0.450477126973457,-0.494589494695984,
-0.491742431225631));
#41375=CARTESIAN_POINT('Ctrl Pts',(-0.158732544136138,-0.64988644363315,
-0.481121218904899));
#41376=CARTESIAN_POINT('Ctrl Pts',(0.171753501841992,-0.646567200522882,
-0.470500006584167));
#41377=CARTESIAN_POINT('Ctrl Pts',(0.460320091431361,-0.48544188489642,
-0.459878794263435));
#41378=CARTESIAN_POINT('Ctrl Pts',(0.636537484106821,-0.205835957776284,
-0.449257581942702));
#41379=CARTESIAN_POINT('Ctrl Pts',(0.657396732580188,0.124007847251966,
-0.43863636962197));
#41380=CARTESIAN_POINT('Ctrl Pts',(0.517806771181053,0.423585360825624,
-0.428015157301238));
#41381=CARTESIAN_POINT('Ctrl Pts',(0.251836979788509,0.619779433184232,
-0.417393944980505));
#41382=CARTESIAN_POINT('Ctrl Pts',(-0.0755980462515238,0.664705457770534,
-0.406772732659774));
#41383=CARTESIAN_POINT('Ctrl Pts',(-0.384582042358491,0.547398449834714,
-0.39615152033904));
#41384=CARTESIAN_POINT('Ctrl Pts',(-0.599702041634294,0.296489243396025,
-0.385530308018309));
#41385=CARTESIAN_POINT('Ctrl Pts',(-0.668454232892285,-0.0267833662666586,
-0.374909095697576));
#41386=CARTESIAN_POINT('Ctrl Pts',(-0.574058437290037,-0.343519025346637,
-0.364287883376844));
#41387=CARTESIAN_POINT('Ctrl Pts',(-0.339553605322675,-0.576412837542728,
-0.353666671056111));
#41388=CARTESIAN_POINT('Ctrl Pts',(-0.0221747569089046,-0.668622980721422,
-0.343045458735379));
#41389=CARTESIAN_POINT('Ctrl Pts',(0.300616230262104,-0.597643951136341,
-0.332424246414647));
#41390=CARTESIAN_POINT('Ctrl Pts',(0.550036550302552,-0.380799426675277,
-0.321803034093914));
#41391=CARTESIAN_POINT('Ctrl Pts',(0.665210797783139,-0.0710141190690022,
-0.311181821773182));
#41392=CARTESIAN_POINT('Ctrl Pts',(0.618028674331743,0.256103430490016,
-0.30056060945245));
#41393=CARTESIAN_POINT('Ctrl Pts',(0.420005809134218,0.520714443433612,
-0.289939397131717));
#41394=CARTESIAN_POINT('Ctrl Pts',(0.119473149966588,0.658235957542453,
-0.279318184810985));
#41395=CARTESIAN_POINT('Ctrl Pts',(-0.210219017943201,0.635103434988625,
-0.268696972490253));
#41396=CARTESIAN_POINT('Ctrl Pts',(-0.488603565549287,0.456962771519233,
-0.25807576016952));
#41397=CARTESIAN_POINT('Ctrl Pts',(-0.647735797590754,0.167292327094403,
-0.247454547848788));
#41398=CARTESIAN_POINT('Ctrl Pts',(-0.648776820735564,-0.163208751908622,
-0.236833335528056));
#41399=CARTESIAN_POINT('Ctrl Pts',(-0.491472315475939,-0.453875858438117,
-0.226212123207324));
#41400=CARTESIAN_POINT('Ctrl Pts',(-0.214215682544731,-0.633766620558494,
-0.215590910886591));
#41401=CARTESIAN_POINT('Ctrl Pts',(0.115324674990204,-0.658975468022751,
-0.204969698565859));
#41402=CARTESIAN_POINT('Ctrl Pts',(0.416716775328578,-0.523349883470236,
-0.194348486245126));
#41403=CARTESIAN_POINT('Ctrl Pts',(0.616404307509721,-0.259991384615625,
-0.183727273924394));
#41404=CARTESIAN_POINT('Ctrl Pts',(0.66564263859121,0.0668221963899351,
-0.173106061603661));
#41405=CARTESIAN_POINT('Ctrl Pts',(0.552428954539379,0.377327397940862,
-0.162484849282929));
#41406=CARTESIAN_POINT('Ctrl Pts',(0.304365909285143,0.595737740289611,
-0.151863636962197));
#41407=CARTESIAN_POINT('Ctrl Pts',(-0.0179442774568819,0.668750733104762,
-0.141242424641465));
#41408=CARTESIAN_POINT('Ctrl Pts',(-0.33595438712131,0.578538159640864,
-0.130621212320732));
#41409=CARTESIAN_POINT('Ctrl Pts',(-0.493165134596604,0.424261513660227,
-0.123540404106911));
#41410=CARTESIAN_POINT('Ctrl Pts',(-0.548572772984126,0.332979158385831,
-0.12));
#41411=CARTESIAN_POINT('Ctrl Pts',(0.462889160393653,-0.444455658495748,
-0.72625));
#41412=CARTESIAN_POINT('Ctrl Pts',(0.535135327429651,-0.369213129884151,
-0.722791509249761));
#41413=CARTESIAN_POINT('Ctrl Pts',(0.642190315853192,-0.182914675178815,
-0.715874527749283));
#41414=CARTESIAN_POINT('Ctrl Pts',(0.653014131807411,0.139347482177261,
-0.705499055498563));
#41415=CARTESIAN_POINT('Ctrl Pts',(0.511617065765403,0.429054145801984,
-0.695123583247846));
#41416=CARTESIAN_POINT('Ctrl Pts',(0.25094192882907,0.618770941114435,-0.684748110997127));
#41417=CARTESIAN_POINT('Ctrl Pts',(-0.0682312037537184,0.664218747915985,
-0.674372638746408));
#41418=CARTESIAN_POINT('Ctrl Pts',(-0.37149945364269,0.554828066014907,
-0.663997166495691));
#41419=CARTESIAN_POINT('Ctrl Pts',(-0.588160489258797,0.316087911596656,
-0.653621694244971));
#41420=CARTESIAN_POINT('Ctrl Pts',(-0.667706091050652,0.00366142581770804,
-0.643246221994255));
#41421=CARTESIAN_POINT('Ctrl Pts',(-0.591591447850655,-0.309619723170008,
-0.632870749743535));
#41422=CARTESIAN_POINT('Ctrl Pts',(-0.377561216430721,-0.550719737673313,
-0.622495277492817));
#41423=CARTESIAN_POINT('Ctrl Pts',(-0.0755113770637089,-0.663432617182758,
-0.612119805242099));
#41424=CARTESIAN_POINT('Ctrl Pts',(0.244142145282362,-0.621481580233081,
-0.601744332991381));
#41425=CARTESIAN_POINT('Ctrl Pts',(0.506879657041181,-0.434646736395633,
-0.591368860740661));
#41426=CARTESIAN_POINT('Ctrl Pts',(0.651450040389794,-0.146484149712398,
-0.580993388489944));
#41427=CARTESIAN_POINT('Ctrl Pts',(0.644150106010189,0.175827768496734,
-0.570617916239225));
#41428=CARTESIAN_POINT('Ctrl Pts',(0.486681657639716,0.457149568902442,
-0.560242443988508));
#41429=CARTESIAN_POINT('Ctrl Pts',(0.215754778891774,0.631897648543906,
-0.549866971737789));
#41430=CARTESIAN_POINT('Ctrl Pts',(-0.105470274367959,0.659333591630754,
-0.53949149948707));
#41431=CARTESIAN_POINT('Ctrl Pts',(-0.402107402880485,0.53306134717955,
-0.529116027236352));
#41432=CARTESIAN_POINT('Ctrl Pts',(-0.605002607191347,0.28251833358982,
-0.518740554985634));
#41433=CARTESIAN_POINT('Ctrl Pts',(-0.666855621715713,-0.0338872136604341,
-0.508365082734916));
#41434=CARTESIAN_POINT('Ctrl Pts',(-0.573246864690785,-0.342392750484064,
-0.497989610484197));
#41435=CARTESIAN_POINT('Ctrl Pts',(-0.345999025618036,-0.571077435861077,
-0.487614138233478));
#41436=CARTESIAN_POINT('Ctrl Pts',(-0.0380896164391166,-0.666628790695116,
-0.477238665982761));
#41437=CARTESIAN_POINT('Ctrl Pts',(0.278699494821865,-0.60677125431137,
-0.466863193732042));
#41438=CARTESIAN_POINT('Ctrl Pts',(0.530516345532464,-0.405459209528553,
-0.456487721481324));
#41439=CARTESIAN_POINT('Ctrl Pts',(0.658655734075261,-0.109623845215152,
-0.446112249230605));
#41440=CARTESIAN_POINT('Ctrl Pts',(0.633244962817189,0.211767751408133,
-0.435736776979887));
#41441=CARTESIAN_POINT('Ctrl Pts',(0.46020795800052,0.483790656030648,-0.425361304729169));
#41442=CARTESIAN_POINT('Ctrl Pts',(0.179884245065169,0.643029098756216,
-0.414985832478451));
#41443=CARTESIAN_POINT('Ctrl Pts',(-0.142375267023613,0.652360365756174,
-0.404610360227732));
#41444=CARTESIAN_POINT('Ctrl Pts',(-0.431443319792535,0.509609090653018,
-0.394234887977014));
#41445=CARTESIAN_POINT('Ctrl Pts',(-0.619930466222754,0.248054390242977,
-0.383859415726295));
#41446=CARTESIAN_POINT('Ctrl Pts',(-0.663895342170731,-0.0713283822377002,
-0.373483943475577));
#41447=CARTESIAN_POINT('Ctrl Pts',(-0.553088566396638,-0.374082612792774,
-0.363108471224859));
#41448=CARTESIAN_POINT('Ctrl Pts',(-0.313342143756286,-0.58962824254807,
-0.35273299897414));
#41449=CARTESIAN_POINT('Ctrl Pts',(-0.000547338252603717,-0.667715855659524,
-0.342357526723423));
#41450=CARTESIAN_POINT('Ctrl Pts',(0.312375066371514,-0.590141153768528,
-0.331982054472704));
#41451=CARTESIAN_POINT('Ctrl Pts',(0.55247453951602,-0.374988862034699,
-0.321606582221986));
#41452=CARTESIAN_POINT('Ctrl Pts',(0.663777511885435,-0.0724166986121209,
-0.311231109971267));
#41453=CARTESIAN_POINT('Ctrl Pts',(0.620336301707957,0.247037722001034,
-0.300855637720549));
#41454=CARTESIAN_POINT('Ctrl Pts',(0.432278210394921,0.508901083360732,
-0.29048016546983));
#41455=CARTESIAN_POINT('Ctrl Pts',(0.14344457678541,0.652126073885111,-0.280104693219112));
#41456=CARTESIAN_POINT('Ctrl Pts',(-0.178829799152076,0.643323143657881,
-0.269729220968394));
#41457=CARTESIAN_POINT('Ctrl Pts',(-0.459414198332819,0.48454448466337,
-0.259353748717676));
#41458=CARTESIAN_POINT('Ctrl Pts',(-0.632896929856003,0.212805632960395,
-0.248978276466957));
#41459=CARTESIAN_POINT('Ctrl Pts',(-0.658834575522026,-0.108543881809492,
-0.238602804216239));
#41460=CARTESIAN_POINT('Ctrl Pts',(-0.531180344891156,-0.404588906018681,
-0.228227331965521));
#41461=CARTESIAN_POINT('Ctrl Pts',(-0.279693903529316,-0.606313554142205,
-0.217851859714802));
#41462=CARTESIAN_POINT('Ctrl Pts',(0.0369967156354772,-0.666690291400585,
-0.207476387464084));
#41463=CARTESIAN_POINT('Ctrl Pts',(0.345062229691949,-0.571644007915702,
-0.197100915213366));
#41464=CARTESIAN_POINT('Ctrl Pts',(0.572684938105708,-0.343331897341362,
-0.186725442962647));
#41465=CARTESIAN_POINT('Ctrl Pts',(0.666798823765209,-0.0349808177150975,
-0.176349970711929));
#41466=CARTESIAN_POINT('Ctrl Pts',(0.605465652234757,0.281526856371821,
-0.165974498461211));
#41467=CARTESIAN_POINT('Ctrl Pts',(0.402979412578655,0.532399882876135,
-0.155599026210492));
#41468=CARTESIAN_POINT('Ctrl Pts',(0.106553789103513,0.659162816942658,
-0.145223553959774));
#41469=CARTESIAN_POINT('Ctrl Pts',(-0.214723962090429,0.632244495520886,
-0.134848081709056));
#41470=CARTESIAN_POINT('Ctrl Pts',(-0.485920592934187,0.457958900439567,
-0.124472609458337));
#41471=CARTESIAN_POINT('Ctrl Pts',(-0.643884510525116,0.176858466795417,
-0.114097137207619));
#41472=CARTESIAN_POINT('Ctrl Pts',(-0.649036352703418,-0.0379468946230774,
-0.10718015570714));
#41473=CARTESIAN_POINT('Ctrl Pts',(-0.626319218357157,-0.139754942292966,
-0.103721664956901));
#41474=CARTESIAN_POINT('Ctrl Pts',(0.464718942461958,-0.44621257367903,
-0.727570523102925));
#41475=CARTESIAN_POINT('Ctrl Pts',(0.537250663424813,-0.37067264798198,
-0.724112032352686));
#41476=CARTESIAN_POINT('Ctrl Pts',(0.644728882109174,-0.183637706565169,
-0.717195050852207));
#41477=CARTESIAN_POINT('Ctrl Pts',(0.655595457840136,0.139898306064466,
-0.706819578601489));
#41478=CARTESIAN_POINT('Ctrl Pts',(0.513639468333482,0.430750181907022,
-0.69644410635077));
#41479=CARTESIAN_POINT('Ctrl Pts',(0.251933888482677,0.621216911245235,
-0.686068634100052));
#41480=CARTESIAN_POINT('Ctrl Pts',(-0.0685009174702088,0.666844374933673,
-0.675693161849334));
#41481=CARTESIAN_POINT('Ctrl Pts',(-0.372967974187952,0.557021274844762,
-0.665317689598615));
#41482=CARTESIAN_POINT('Ctrl Pts',(-0.590485459981355,0.31733739269549,
-0.654942217347898));
#41483=CARTESIAN_POINT('Ctrl Pts',(-0.670345502226871,0.00367589910057958,
-0.644566745097178));
#41484=CARTESIAN_POINT('Ctrl Pts',(-0.593929981190927,-0.310843635416322,
-0.634191272846461));
#41485=CARTESIAN_POINT('Ctrl Pts',(-0.379053698347304,-0.552896707157342,
-0.623815800595742));
#41486=CARTESIAN_POINT('Ctrl Pts',(-0.0758098699991723,-0.666055135361883,
-0.613440328345024));
#41487=CARTESIAN_POINT('Ctrl Pts',(0.245107227789762,-0.623938267950393,
-0.603064856094305));
#41488=CARTESIAN_POINT('Ctrl Pts',(0.508883328693909,-0.436364874671762,
-0.592689383843588));
#41489=CARTESIAN_POINT('Ctrl Pts',(0.654025192020124,-0.147063194728269,
-0.582313911592868));
#41490=CARTESIAN_POINT('Ctrl Pts',(0.646696401343553,0.176522807468057,
-0.571938439342151));
#41491=CARTESIAN_POINT('Ctrl Pts',(0.48860548753781,0.458956659830723,-0.561562967091432));
#41492=CARTESIAN_POINT('Ctrl Pts',(0.216607647472342,0.634395510483487,
-0.551187494840714));
#41493=CARTESIAN_POINT('Ctrl Pts',(-0.105887193444585,0.661939906573517,
-0.540812022589996));
#41494=CARTESIAN_POINT('Ctrl Pts',(-0.403696914693697,0.535168513828335,
-0.530436550339277));
#41495=CARTESIAN_POINT('Ctrl Pts',(-0.607394154286282,0.283635115388603,
-0.520061078088559));
#41496=CARTESIAN_POINT('Ctrl Pts',(-0.669491670892799,-0.0340211682358486,
-0.509685605837841));
#41497=CARTESIAN_POINT('Ctrl Pts',(-0.575512882816362,-0.343746213060933,
-0.499310133587123));
#41498=CARTESIAN_POINT('Ctrl Pts',(-0.347366743632334,-0.573334878335637,
-0.488934661336404));
#41499=CARTESIAN_POINT('Ctrl Pts',(-0.0382401829167803,-0.669263943219774,
-0.478559189085686));
#41500=CARTESIAN_POINT('Ctrl Pts',(0.279801180929114,-0.609169792785862,
-0.468183716834967));
#41501=CARTESIAN_POINT('Ctrl Pts',(0.532613451908327,-0.40706197087722,
-0.457808244584249));
#41502=CARTESIAN_POINT('Ctrl Pts',(0.661259369478884,-0.110057183163517,
-0.44743277233353));
#41503=CARTESIAN_POINT('Ctrl Pts',(0.635748150626934,0.212604859454699,
-0.437057300082813));
#41504=CARTESIAN_POINT('Ctrl Pts',(0.462027138598958,0.485703057934735,
-0.426681827832093));
#41505=CARTESIAN_POINT('Ctrl Pts',(0.180595319097893,0.645570962799093,
-0.416306355581376));
#41506=CARTESIAN_POINT('Ctrl Pts',(-0.142938069815186,0.654939115862385,
-0.405930883330657));
#41507=CARTESIAN_POINT('Ctrl Pts',(-0.433148795117433,0.51162355162525,
-0.395555411079939));
#41508=CARTESIAN_POINT('Ctrl Pts',(-0.622381022448319,0.249034937680809,
-0.385179938829221));
#41509=CARTESIAN_POINT('Ctrl Pts',(-0.666519689500831,-0.0716103400066377,
-0.374804466578503));
#41510=CARTESIAN_POINT('Ctrl Pts',(-0.555274899709033,-0.375561343917636,
-0.364428994327784));
#41511=CARTESIAN_POINT('Ctrl Pts',(-0.314580770639381,-0.591959015496446,
-0.354053522077066));
#41512=CARTESIAN_POINT('Ctrl Pts',(-0.000549501855194795,-0.670355305301288,
-0.343678049826347));
#41513=CARTESIAN_POINT('Ctrl Pts',(0.313609870442805,-0.592473954231052,
-0.333302577575629));
#41514=CARTESIAN_POINT('Ctrl Pts',(0.554658445608785,-0.37647117552053,
-0.32292710532491));
#41515=CARTESIAN_POINT('Ctrl Pts',(0.666401393437919,-0.0727029584449918,
-0.312551633074193));
#41516=CARTESIAN_POINT('Ctrl Pts',(0.622788462182255,0.248014250596821,
-0.302176160823474));
#41517=CARTESIAN_POINT('Ctrl Pts',(0.43398698600347,0.510912745612938,-0.291800688572756));
#41518=CARTESIAN_POINT('Ctrl Pts',(0.144011606508548,0.654703897846908,
-0.281425216322037));
#41519=CARTESIAN_POINT('Ctrl Pts',(-0.179536705009153,0.645866170045693,
-0.271049744071319));
#41520=CARTESIAN_POINT('Ctrl Pts',(-0.461230241236544,0.486459866418583,
-0.260674271820601));
#41521=CARTESIAN_POINT('Ctrl Pts',(-0.635398741907202,0.213646843700976,
-0.250298799569883));
#41522=CARTESIAN_POINT('Ctrl Pts',(-0.661438917878502,-0.108972950706181,
-0.239923327319164));
#41523=CARTESIAN_POINT('Ctrl Pts',(-0.533280076023624,-0.406188227111467,
-0.229547855068446));
#41524=CARTESIAN_POINT('Ctrl Pts',(-0.280799520491592,-0.608710283322796,
-0.219172382817727));
#41525=CARTESIAN_POINT('Ctrl Pts',(0.0371429619347367,-0.669325687087322,
-0.208796910567009));
#41526=CARTESIAN_POINT('Ctrl Pts',(0.346426244580695,-0.573903689918445,
-0.198421438316291));
#41527=CARTESIAN_POINT('Ctrl Pts',(0.574948734991407,-0.344689072530265,
-0.188045966065572));
#41528=CARTESIAN_POINT('Ctrl Pts',(0.669434648363557,-0.035119094842057,
-0.177670493814854));
#41529=CARTESIAN_POINT('Ctrl Pts',(0.607859029842677,0.282639718083408,
-0.167295021564136));
#41530=CARTESIAN_POINT('Ctrl Pts',(0.404572371171796,0.534504436426277,
-0.156919549313418));
#41531=CARTESIAN_POINT('Ctrl Pts',(0.106974991728399,0.661768453560443,
-0.146544077062699));
#41532=CARTESIAN_POINT('Ctrl Pts',(-0.215572756826861,0.634743735027689,
-0.136168604811981));
#41533=CARTESIAN_POINT('Ctrl Pts',(-0.487841412514633,0.459769177540265,
-0.125793132561263));
#41534=CARTESIAN_POINT('Ctrl Pts',(-0.646429759948626,0.17755760797843,
-0.115417660310544));
#41535=CARTESIAN_POINT('Ctrl Pts',(-0.651601956932064,-0.038096942589642,
-0.108500678810065));
#41536=CARTESIAN_POINT('Ctrl Pts',(-0.628795032813062,-0.14030738790899,
-0.105042188059826));
#41537=CARTESIAN_POINT('Ctrl Pts',(0.468463827977225,-0.449808327695529,
-0.732058124057058));
#41538=CARTESIAN_POINT('Ctrl Pts',(0.541579446992128,-0.373660287164295,
-0.728599633306819));
#41539=CARTESIAN_POINT('Ctrl Pts',(0.649924613974643,-0.185117110828464,
-0.721682651806341));
#41540=CARTESIAN_POINT('Ctrl Pts',(0.660878274402623,0.141025458328198,
-0.711307179555621));
#41541=CARTESIAN_POINT('Ctrl Pts',(0.5177785939746,0.434221379345974,-0.700931707304904));
#41542=CARTESIAN_POINT('Ctrl Pts',(0.253964003373025,0.626222802832036,
-0.690556235054185));
#41543=CARTESIAN_POINT('Ctrl Pts',(-0.0690528976258993,0.672218015378987,
-0.680180762803467));
#41544=CARTESIAN_POINT('Ctrl Pts',(-0.375973463283883,0.561509895041683,
-0.66980529055275));
#41545=CARTESIAN_POINT('Ctrl Pts',(-0.595243750791249,0.319894591382352,
-0.659429818302029));
#41546=CARTESIAN_POINT('Ctrl Pts',(-0.67574733472572,0.00370551753535922,
-0.649054346051313));
#41547=CARTESIAN_POINT('Ctrl Pts',(-0.59871603254323,-0.313348498179755,
-0.638678873800593));
#41548=CARTESIAN_POINT('Ctrl Pts',(-0.382108218840265,-0.557352102985363,
-0.628303401549875));
#41549=CARTESIAN_POINT('Ctrl Pts',(-0.0764207666551862,-0.67142239206951,
-0.617927929299157));
#41550=CARTESIAN_POINT('Ctrl Pts',(0.247082369683177,-0.628966135823776,
-0.607552457048439));
#41551=CARTESIAN_POINT('Ctrl Pts',(0.512984051831413,-0.439881223811224,
-0.59717698479772));
#41552=CARTESIAN_POINT('Ctrl Pts',(0.659295508445708,-0.148248270804131,
-0.586801512547002));
#41553=CARTESIAN_POINT('Ctrl Pts',(0.651907660399777,0.177945277253391,
-0.576426040296284));
#41554=CARTESIAN_POINT('Ctrl Pts',(0.49254280611635,0.462655059926965,-0.566050568045565));
#41555=CARTESIAN_POINT('Ctrl Pts',(0.218353132001307,0.639507645534371,
-0.555675095794847));
#41556=CARTESIAN_POINT('Ctrl Pts',(-0.106740461831666,0.667274002001449,
-0.545299623544128));
#41557=CARTESIAN_POINT('Ctrl Pts',(-0.40695001644199,0.539481050203778,
-0.534924151293411));
#41558=CARTESIAN_POINT('Ctrl Pts',(-0.612288704911572,0.28592072584588,
-0.524548679042691));
#41559=CARTESIAN_POINT('Ctrl Pts',(-0.674886620535706,-0.0342953202487183,
-0.514173206791974));
#41560=CARTESIAN_POINT('Ctrl Pts',(-0.580150525309795,-0.346516215422834,
-0.503797734541255));
#41561=CARTESIAN_POINT('Ctrl Pts',(-0.350165921233864,-0.577954969864389,
-0.493422262290537));
#41562=CARTESIAN_POINT('Ctrl Pts',(-0.0385483329210009,-0.674657057770278,
-0.483046790039819));
#41563=CARTESIAN_POINT('Ctrl Pts',(0.282055896479539,-0.614078651998191,
-0.4726713177891));
#41564=CARTESIAN_POINT('Ctrl Pts',(0.536905398884327,-0.410342189183201,
-0.462295845538382));
#41565=CARTESIAN_POINT('Ctrl Pts',(0.666587980953165,-0.11094405448224,
-0.451920373287663));
#41566=CARTESIAN_POINT('Ctrl Pts',(0.64087118562128,0.214318088402166,-0.441544901036946));
#41567=CARTESIAN_POINT('Ctrl Pts',(0.46575028147723,0.489616987940208,-0.431169428786226));
#41568=CARTESIAN_POINT('Ctrl Pts',(0.182050606287704,0.65077315273939,-0.420793956535509));
#41569=CARTESIAN_POINT('Ctrl Pts',(-0.144089904441783,0.660216796979385,
-0.41041848428479));
#41570=CARTESIAN_POINT('Ctrl Pts',(-0.436639228291258,0.515746356160854,
-0.400043012034072));
#41571=CARTESIAN_POINT('Ctrl Pts',(-0.627396341414921,0.251041730306632,
-0.389667539783354));
#41572=CARTESIAN_POINT('Ctrl Pts',(-0.671890690093387,-0.072187395995648,
-0.379292067532636));
#41573=CARTESIAN_POINT('Ctrl Pts',(-0.559749458919139,-0.378587721431273,
-0.368916595281917));
#41574=CARTESIAN_POINT('Ctrl Pts',(-0.317115749773712,-0.596729185490112,
-0.358541123031199));
#41575=CARTESIAN_POINT('Ctrl Pts',(-0.00055392989362848,-0.675757214350081,
-0.348165650780481));
#41576=CARTESIAN_POINT('Ctrl Pts',(0.316137025794007,-0.597248273744105,
-0.337790178529762));
#41577=CARTESIAN_POINT('Ctrl Pts',(0.559128037260631,-0.3795048847092,-0.327414706279044));
#41578=CARTESIAN_POINT('Ctrl Pts',(0.671771440768122,-0.0732888190575194,
-0.317039234028325));
#41579=CARTESIAN_POINT('Ctrl Pts',(0.627807064410998,0.250012818244892,
-0.306663761777607));
#41580=CARTESIAN_POINT('Ctrl Pts',(0.437484173552585,0.515029822272535,
-0.296288289526889));
#41581=CARTESIAN_POINT('Ctrl Pts',(0.145172091990569,0.65997968351971,-0.28591281727617));
#41582=CARTESIAN_POINT('Ctrl Pts',(-0.180983461590688,0.651070738832306,
-0.275537345025452));
#41583=CARTESIAN_POINT('Ctrl Pts',(-0.464946962499182,0.490379895027805,
-0.265161872774734));
#41584=CARTESIAN_POINT('Ctrl Pts',(-0.640518961260343,0.215368469184956,
-0.254786400524015));
#41585=CARTESIAN_POINT('Ctrl Pts',(-0.666768976221095,-0.1098510848563,
-0.244410928273297));
#41586=CARTESIAN_POINT('Ctrl Pts',(-0.537577394806923,-0.409461404791647,
-0.234035456022579));
#41587=CARTESIAN_POINT('Ctrl Pts',(-0.283062281008399,-0.613615439195291,
-0.223659983771861));
#41588=CARTESIAN_POINT('Ctrl Pts',(0.0374422703654468,-0.674719300151826,
-0.213284511521142));
#41589=CARTESIAN_POINT('Ctrl Pts',(0.349217843106239,-0.578528363169896,
-0.202909039270424));
#41590=CARTESIAN_POINT('Ctrl Pts',(0.57958183196945,-0.347466676531802,
-0.192533567019706));
#41591=CARTESIAN_POINT('Ctrl Pts',(0.674829137420516,-0.0354020866616497,
-0.182158094768987));
#41592=CARTESIAN_POINT('Ctrl Pts',(0.612757328717359,0.28491729225613,-0.171782622518269));
#41593=CARTESIAN_POINT('Ctrl Pts',(0.407832523308644,0.538811651509414,
-0.161407150267551));
#41594=CARTESIAN_POINT('Ctrl Pts',(0.10783703441614,0.667101107632415,-0.151031678016832));
#41595=CARTESIAN_POINT('Ctrl Pts',(-0.21730991889707,0.639858795210619,
-0.140656205766114));
#41596=CARTESIAN_POINT('Ctrl Pts',(-0.491772539806295,0.463473885528119,
-0.130280733515396));
#41597=CARTESIAN_POINT('Ctrl Pts',(-0.651638943195009,0.178988927823084,
-0.119905261264677));
#41598=CARTESIAN_POINT('Ctrl Pts',(-0.656852632537107,-0.0384047749254474,
-0.112988279764198));
#41599=CARTESIAN_POINT('Ctrl Pts',(-0.633862107113883,-0.14143803926975,
-0.109529789013959));
#41600=CARTESIAN_POINT('Ctrl Pts',(0.470014347211915,-0.451297101048697,
-0.738715226741092));
#41601=CARTESIAN_POINT('Ctrl Pts',(0.54337417968881,-0.374894718465072,
-0.735256735990852));
#41602=CARTESIAN_POINT('Ctrl Pts',(0.652074769329847,-0.185731384534561,
-0.728339754490373));
#41603=CARTESIAN_POINT('Ctrl Pts',(0.663066493609553,0.141492983497566,
-0.717964282239655));
#41604=CARTESIAN_POINT('Ctrl Pts',(0.519492261637952,0.435658392894028,
-0.707588809988937));
#41605=CARTESIAN_POINT('Ctrl Pts',(0.254804820165469,0.628295904325486,
-0.697213337738218));
#41606=CARTESIAN_POINT('Ctrl Pts',(-0.0692815491306441,0.67444310756472,
-0.6868378654875));
#41607=CARTESIAN_POINT('Ctrl Pts',(-0.377217976623324,0.563368652712182,
-0.676462393236782));
#41608=CARTESIAN_POINT('Ctrl Pts',(-0.597214148502112,0.320953486159955,
-0.666086920986063));
#41609=CARTESIAN_POINT('Ctrl Pts',(-0.677984188465101,0.00371779474059088,
-0.655711448735345));
#41610=CARTESIAN_POINT('Ctrl Pts',(-0.600697910587708,-0.314385751893901,
-0.645335976484627));
#41611=CARTESIAN_POINT('Ctrl Pts',(-0.383373073457732,-0.559197050461262,
-0.634960504233908));
#41612=CARTESIAN_POINT('Ctrl Pts',(-0.076673736305239,-0.673644939952962,
-0.62458503198319));
#41613=CARTESIAN_POINT('Ctrl Pts',(0.247900263823826,-0.631048142615807,
-0.614209559732472));
#41614=CARTESIAN_POINT('Ctrl Pts',(0.514682134447219,-0.441337321657616,
-0.603834087481753));
#41615=CARTESIAN_POINT('Ctrl Pts',(0.661477912573016,-0.148739002946069,
-0.593458615231035));
#41616=CARTESIAN_POINT('Ctrl Pts',(0.654065609005064,0.178534312695462,
-0.583083142980317));
#41617=CARTESIAN_POINT('Ctrl Pts',(0.494173224329236,0.464186543549856,
-0.572707670729598));
#41618=CARTESIAN_POINT('Ctrl Pts',(0.21907592584049,0.641624547587032,-0.56233219847888));
#41619=CARTESIAN_POINT('Ctrl Pts',(-0.107093794744453,0.669482816449697,
-0.551956726228162));
#41620=CARTESIAN_POINT('Ctrl Pts',(-0.408297104852174,0.541266843632825,
-0.541581253977443));
#41621=CARTESIAN_POINT('Ctrl Pts',(-0.614315506682938,0.286867182364573,
-0.531205781726725));
#41622=CARTESIAN_POINT('Ctrl Pts',(-0.677120634309526,-0.0344088448266699,
-0.520830309476007));
#41623=CARTESIAN_POINT('Ctrl Pts',(-0.58207094308648,-0.347663255493916,
-0.510454837225289));
#41624=CARTESIAN_POINT('Ctrl Pts',(-0.351325042584235,-0.579868119901137,
-0.50007936497457));
#41625=CARTESIAN_POINT('Ctrl Pts',(-0.0386759358456004,-0.676890311642653,
-0.489703892723852));
#41626=CARTESIAN_POINT('Ctrl Pts',(0.282989559613697,-0.616111378865716,
-0.479328420473133));
#41627=CARTESIAN_POINT('Ctrl Pts',(0.538682666382641,-0.411700506379297,
-0.468952948222416));
#41628=CARTESIAN_POINT('Ctrl Pts',(0.66879452451883,-0.111311302162335,
-0.458577475971697));
#41629=CARTESIAN_POINT('Ctrl Pts',(0.642992601295546,0.215027525434478,
-0.448202003720979));
#41630=CARTESIAN_POINT('Ctrl Pts',(0.467292010875556,0.491237721054596,
-0.43782653147026));
#41631=CARTESIAN_POINT('Ctrl Pts',(0.182653231305575,0.652927345965089,
-0.427451059219542));
#41632=CARTESIAN_POINT('Ctrl Pts',(-0.144566871714838,0.662402250613341,
-0.417075586968824));
#41633=CARTESIAN_POINT('Ctrl Pts',(-0.438084594105287,0.517453582867965,
-0.406700114718105));
#41634=CARTESIAN_POINT('Ctrl Pts',(-0.629473152578393,0.251872730160416,
-0.396324642467387));
#41635=CARTESIAN_POINT('Ctrl Pts',(-0.674114786718943,-0.0724263511503591,
-0.385949170216669));
#41636=CARTESIAN_POINT('Ctrl Pts',(-0.561602344963072,-0.379840924796351,
-0.375573697965951));
#41637=CARTESIAN_POINT('Ctrl Pts',(-0.318165468246377,-0.59870448204835,
-0.365198225715232));
#41638=CARTESIAN_POINT('Ctrl Pts',(-0.000555763515644371,-0.67799410996808,
-0.354822753464514));
#41639=CARTESIAN_POINT('Ctrl Pts',(0.317183504488467,-0.599225288590716,
-0.344447281213795));
#41640=CARTESIAN_POINT('Ctrl Pts',(0.560978866271118,-0.380761124075465,
-0.334071808963077));
#41641=CARTESIAN_POINT('Ctrl Pts',(0.673995142653298,-0.073531420145835,
-0.323696336712359));
#41642=CARTESIAN_POINT('Ctrl Pts',(0.629885235153281,0.250840412180345,
-0.313320864461641));
#41643=CARTESIAN_POINT('Ctrl Pts',(0.438932336307417,0.5167346771196,-0.302945392210922));
#41644=CARTESIAN_POINT('Ctrl Pts',(0.145652641531586,0.662164352229869,
-0.292569919960204));
#41645=CARTESIAN_POINT('Ctrl Pts',(-0.181582554148068,0.653225917187752,
-0.282194447709485));
#41646=CARTESIAN_POINT('Ctrl Pts',(-0.466486032729584,0.492003153405566,
-0.271818975458767));
#41647=CARTESIAN_POINT('Ctrl Pts',(-0.642639211032385,0.216081383425365,
-0.261443503208049));
#41648=CARTESIAN_POINT('Ctrl Pts',(-0.668976118852786,-0.11021471504172,
-0.251068030957331));
#41649=CARTESIAN_POINT('Ctrl Pts',(-0.539356886880686,-0.410816805495047,
-0.240692558706612));
#41650=CARTESIAN_POINT('Ctrl Pts',(-0.283999275223193,-0.615646634552595,
-0.230317086455894));
#41651=CARTESIAN_POINT('Ctrl Pts',(0.03756621147893,-0.676952756440303,
-0.219941614205175));
#41652=CARTESIAN_POINT('Ctrl Pts',(0.350373827149244,-0.58044341845448,
-0.209566141954457));
#41653=CARTESIAN_POINT('Ctrl Pts',(0.581500365212223,-0.348616848509172,
-0.199190669703739));
#41654=CARTESIAN_POINT('Ctrl Pts',(0.677062964974281,-0.0355193033372838,
-0.18881519745302));
#41655=CARTESIAN_POINT('Ctrl Pts',(0.614785673653287,0.285860483832951,
-0.178439725202302));
#41656=CARTESIAN_POINT('Ctrl Pts',(0.409182549063095,0.540595116453827,
-0.168064252951584));
#41657=CARTESIAN_POINT('Ctrl Pts',(0.108193965249678,0.669309573855992,
-0.157688780700866));
#41658=CARTESIAN_POINT('Ctrl Pts',(-0.218029195802555,0.641976413101301,
-0.147313308450147));
#41659=CARTESIAN_POINT('Ctrl Pts',(-0.493400536410654,0.465008978404062,
-0.136937836199429));
#41660=CARTESIAN_POINT('Ctrl Pts',(-0.653795728983253,0.1795794998349,-0.126562363948711));
#41661=CARTESIAN_POINT('Ctrl Pts',(-0.659027376817395,-0.038528764458213,
-0.119645382448232));
#41662=CARTESIAN_POINT('Ctrl Pts',(-0.635960060745575,-0.141906170184684,
-0.116186891697992));
#41663=CARTESIAN_POINT('Ctrl Pts',(0.470014347211915,-0.451297101048697,
-0.742528335043099));
#41664=CARTESIAN_POINT('Ctrl Pts',(0.543372589191722,-0.374896374926965,
-0.73906984429286));
#41665=CARTESIAN_POINT('Ctrl Pts',(0.652075459781473,-0.185730254682432,
-0.732152862792381));
#41666=CARTESIAN_POINT('Ctrl Pts',(0.66306588519074,0.14149243809354,-0.721777390541662));
#41667=CARTESIAN_POINT('Ctrl Pts',(0.519492314280382,0.435658515066948,
-0.711401918290944));
#41668=CARTESIAN_POINT('Ctrl Pts',(0.254804642144546,0.628295593947961,
-0.701026446040226));
#41669=CARTESIAN_POINT('Ctrl Pts',(-0.0692814769404281,0.674442972356818,
-0.690650973789507));
#41670=CARTESIAN_POINT('Ctrl Pts',(-0.377217891740993,0.563368455293,-0.680275501538789));
#41671=CARTESIAN_POINT('Ctrl Pts',(-0.597213959773261,0.320953407732286,
-0.669900029288071));
#41672=CARTESIAN_POINT('Ctrl Pts',(-0.677983995666914,0.00371778562304485,
-0.659524557037352));
#41673=CARTESIAN_POINT('Ctrl Pts',(-0.600697730621323,-0.314385655403825,
-0.649149084786635));
#41674=CARTESIAN_POINT('Ctrl Pts',(-0.383372962378955,-0.559196888039266,
-0.638773612535916));
#41675=CARTESIAN_POINT('Ctrl Pts',(-0.0766737129197174,-0.67364474082535,
-0.628398140285198));
#41676=CARTESIAN_POINT('Ctrl Pts',(0.247900190499642,-0.631047957547907,
-0.618022668034479));
#41677=CARTESIAN_POINT('Ctrl Pts',(0.514681983299422,-0.441337191609865,
-0.60764719578376));
#41678=CARTESIAN_POINT('Ctrl Pts',(0.661477717937038,-0.148738959334052,
-0.597271723533043));
#41679=CARTESIAN_POINT('Ctrl Pts',(0.654065416708807,0.178534260256687,
-0.586896251282324));
#41680=CARTESIAN_POINT('Ctrl Pts',(0.494173078974265,0.46418640700759,-0.576520779031606));
#41681=CARTESIAN_POINT('Ctrl Pts',(0.219075861427449,0.641624358912467,
-0.566145306780888));
#41682=CARTESIAN_POINT('Ctrl Pts',(-0.107093763256759,0.669482619557719,
-0.555769834530169));
#41683=CARTESIAN_POINT('Ctrl Pts',(-0.408296984775409,0.54126668445947,
-0.545394362279451));
#41684=CARTESIAN_POINT('Ctrl Pts',(-0.614315326024746,0.28686709799964,
-0.535018890028733));
#41685=CARTESIAN_POINT('Ctrl Pts',(-0.677120435178814,-0.0344088347065514,
-0.524643417778014));
#41686=CARTESIAN_POINT('Ctrl Pts',(-0.582070771909591,-0.3476631532525,
-0.514267945527297));
#41687=CARTESIAN_POINT('Ctrl Pts',(-0.351324939265201,-0.579867949371361,
-0.503892473276577));
#41688=CARTESIAN_POINT('Ctrl Pts',(-0.0386759244717649,-0.676890112580673,
-0.49351700102586));
#41689=CARTESIAN_POINT('Ctrl Pts',(0.282989476391259,-0.616111197677603,
-0.483141528775141));
#41690=CARTESIAN_POINT('Ctrl Pts',(0.538682507965055,-0.411700385305101,
-0.472766056524423));
#41691=CARTESIAN_POINT('Ctrl Pts',(0.668794327837566,-0.111311269427527,
-0.462390584273704));
#41692=CARTESIAN_POINT('Ctrl Pts',(0.642992412202175,0.215027462198472,
-0.452015112022986));
#41693=CARTESIAN_POINT('Ctrl Pts',(0.467291873452798,0.491237576589808,
-0.441639639772268));
#41694=CARTESIAN_POINT('Ctrl Pts',(0.182653177590315,0.652927153950078,
-0.431264167521549));
#41695=CARTESIAN_POINT('Ctrl Pts',(-0.14456682920014,0.66240205581193,-0.420888695270831));
#41696=CARTESIAN_POINT('Ctrl Pts',(-0.438084465271938,0.517453430693514,
-0.410513223020113));
#41697=CARTESIAN_POINT('Ctrl Pts',(-0.629472967460876,0.251872656088883,
-0.400137750769395));
#41698=CARTESIAN_POINT('Ctrl Pts',(-0.674114588473059,-0.0724263298510245,
-0.389762278518676));
#41699=CARTESIAN_POINT('Ctrl Pts',(-0.561602179805233,-0.379840813091406,
-0.379386806267958));
#41700=CARTESIAN_POINT('Ctrl Pts',(-0.318165374679212,-0.598704305979552,
-0.369011334017239));
#41701=CARTESIAN_POINT('Ctrl Pts',(-0.000555763352252093,-0.677993910581017,
-0.358635861766521));
#41702=CARTESIAN_POINT('Ctrl Pts',(0.317183411210203,-0.599225112369264,
-0.348260389515803));
#41703=CARTESIAN_POINT('Ctrl Pts',(0.560978701296429,-0.380761012098642,
-0.337884917265085));
#41704=CARTESIAN_POINT('Ctrl Pts',(0.673994944442988,-0.0735313985241569,
-0.327509445014366));
#41705=CARTESIAN_POINT('Ctrl Pts',(0.629885049913813,0.250840338417712,
-0.317133972763648));
#41706=CARTESIAN_POINT('Ctrl Pts',(0.438932207226276,0.516734525145969,
-0.306758500512929));
#41707=CARTESIAN_POINT('Ctrl Pts',(0.145652598694571,0.662164157519516,
-0.296383028262211));
#41708=CARTESIAN_POINT('Ctrl Pts',(-0.18158250074169,0.653225725042971,
-0.286007556011493));
#41709=CARTESIAN_POINT('Ctrl Pts',(-0.466485895555756,0.492003008799146,
-0.275632083760774));
#41710=CARTESIAN_POINT('Ctrl Pts',(-0.642639022019262,0.216081319713422,
-0.265256611510056));
#41711=CARTESIAN_POINT('Ctrl Pts',(-0.66897592216521,-0.110214682299213,
-0.254881139259338));
#41712=CARTESIAN_POINT('Ctrl Pts',(-0.539356728171161,-0.410816685337444,
-0.24450566700862));
#41713=CARTESIAN_POINT('Ctrl Pts',(-0.283999191890099,-0.615646452195022,
-0.234130194757901));
#41714=CARTESIAN_POINT('Ctrl Pts',(0.0375662008019495,-0.67695255995773,
-0.223754722507183));
#41715=CARTESIAN_POINT('Ctrl Pts',(0.350373723373049,-0.580443242588805,
-0.213379250256465));
#41716=CARTESIAN_POINT('Ctrl Pts',(0.581500195668746,-0.34861675626341,
-0.203003778005746));
#41717=CARTESIAN_POINT('Ctrl Pts',(0.67706276294556,-0.0355192724524337,
-0.192628305755028));
#41718=CARTESIAN_POINT('Ctrl Pts',(0.614785498654458,0.285860359114252,
-0.18225283350431));
#41719=CARTESIAN_POINT('Ctrl Pts',(0.409182417194479,0.540595038330385,
-0.171877361253591));
#41720=CARTESIAN_POINT('Ctrl Pts',(0.108193956380082,0.66930921615921,-0.161501889002873));
#41721=CARTESIAN_POINT('Ctrl Pts',(-0.218029177410119,0.641976544855489,
-0.151126416752155));
#41722=CARTESIAN_POINT('Ctrl Pts',(-0.493400299308284,0.46500819646962,
-0.140750944501436));
#41723=CARTESIAN_POINT('Ctrl Pts',(-0.653795732950318,0.17958082394726,
-0.130375472250718));
#41724=CARTESIAN_POINT('Ctrl Pts',(-0.659026876700399,-0.0385310057591697,
-0.123458490750239));
#41725=CARTESIAN_POINT('Ctrl Pts',(-0.635960060745575,-0.141906170184684,
-0.12));
#41726=CARTESIAN_POINT('Ctrl Pts',(-0.548572772984126,0.332979158385831,
-0.12));
#41727=CARTESIAN_POINT('Ctrl Pts',(-0.577197265262902,0.291949500684259,
-0.12));
#41728=CARTESIAN_POINT('Ctrl Pts',(-0.611328090029018,0.228891973083493,
-0.12));
#41729=CARTESIAN_POINT('Ctrl Pts',(-0.643583475482228,0.101487125632845,
-0.12));
#41730=CARTESIAN_POINT('Ctrl Pts',(-0.649841246643075,0.0550307489159153,
-0.12));
#41731=CARTESIAN_POINT('Ctrl Pts',(-0.651978221577845,-0.0421309211851907,
-0.12));
#41732=CARTESIAN_POINT('Ctrl Pts',(-0.646960254890958,-0.0926082141634192,
-0.12));
#41733=CARTESIAN_POINT('Ctrl Pts',(-0.635960060745575,-0.141906170184684,
-0.12));
#41734=CARTESIAN_POINT('Origin',(0.,0.,0.0705711144245887));
#41735=CARTESIAN_POINT('',(-0.9025,-1.10524373623049E-16,-5.55111512312578E-17));
#41736=CARTESIAN_POINT('Origin',(0.,0.,0.));
#41737=CARTESIAN_POINT('',(-0.95,-1.33616303797361E-16,0.0274241377865074));
#41738=CARTESIAN_POINT('',(-1.02473275573014,-1.25493568928637E-16,0.0705711144245887));
#41739=CARTESIAN_POINT('',(-0.95,0.548482755730144,0.112274715389696));
#41740=CARTESIAN_POINT('Ctrl Pts',(-0.95,0.548482755730144,0.112274715389696));
#41741=CARTESIAN_POINT('Ctrl Pts',(-0.95,0.254551732809566,0.0274241377865074));
#41742=CARTESIAN_POINT('Ctrl Pts',(-0.95,-1.50891161675723E-16,0.0274241377865074));
#41743=CARTESIAN_POINT('',(6.71697651192441E-17,1.09696551146029,0.112274715389696));
#41744=CARTESIAN_POINT('Ctrl Pts',(6.71697651192441E-17,1.09696551146029,
0.112274715389696));
#41745=CARTESIAN_POINT('Ctrl Pts',(-0.475000000000001,0.822724133595216,
-0.0460586179436371));
#41746=CARTESIAN_POINT('Ctrl Pts',(-0.95,0.548482755730144,0.112274715389696));
#41747=CARTESIAN_POINT('',(0.95,0.548482755730144,0.112274715389696));
#41748=CARTESIAN_POINT('Ctrl Pts',(0.95,0.548482755730144,0.112274715389696));
#41749=CARTESIAN_POINT('Ctrl Pts',(0.475,0.822724133595217,-0.0460586179436373));
#41750=CARTESIAN_POINT('Ctrl Pts',(6.71697651192441E-17,1.09696551146029,
0.112274715389696));
#41751=CARTESIAN_POINT('',(0.95,-0.548482755730145,0.112274715389696));
#41752=CARTESIAN_POINT('Ctrl Pts',(0.95,-0.548482755730145,0.112274715389696));
#41753=CARTESIAN_POINT('Ctrl Pts',(0.95,-1.11022302462516E-16,-0.0460586179436371));
#41754=CARTESIAN_POINT('Ctrl Pts',(0.95,0.548482755730144,0.112274715389696));
#41755=CARTESIAN_POINT('',(-2.01509295357732E-16,-1.09696551146029,0.112274715389696));
#41756=CARTESIAN_POINT('Ctrl Pts',(-2.01509295357732E-16,-1.09696551146029,
0.112274715389696));
#41757=CARTESIAN_POINT('Ctrl Pts',(0.475,-0.822724133595217,-0.0460586179436371));
#41758=CARTESIAN_POINT('Ctrl Pts',(0.95,-0.548482755730145,0.112274715389696));
#41759=CARTESIAN_POINT('',(-0.95,-0.548482755730145,0.112274715389696));
#41760=CARTESIAN_POINT('Ctrl Pts',(-0.95,-0.548482755730145,0.112274715389696));
#41761=CARTESIAN_POINT('Ctrl Pts',(-0.475,-0.822724133595217,-0.0460586179436367));
#41762=CARTESIAN_POINT('Ctrl Pts',(-2.01509295357732E-16,-1.09696551146029,
0.112274715389696));
#41763=CARTESIAN_POINT('Ctrl Pts',(-0.95,-1.50891161675723E-16,0.0274241377865074));
#41764=CARTESIAN_POINT('Ctrl Pts',(-0.95,-0.254551732809567,0.0274241377865074));
#41765=CARTESIAN_POINT('Ctrl Pts',(-0.95,-0.548482755730145,0.112274715389696));
#41766=CARTESIAN_POINT('Origin',(-2.01509295357732E-16,-1.09696551146029,
0.));
#41767=CARTESIAN_POINT('',(0.95,-0.548482755730145,0.587725284610304));
#41768=CARTESIAN_POINT('',(0.95,-0.548482755730145,0.));
#41769=CARTESIAN_POINT('',(-2.01509295357732E-16,-1.09696551146029,0.587725284610304));
#41770=CARTESIAN_POINT('Ctrl Pts',(0.95,-0.548482755730145,0.587725284610304));
#41771=CARTESIAN_POINT('Ctrl Pts',(0.475,-0.822724133595217,0.746058617943637));
#41772=CARTESIAN_POINT('Ctrl Pts',(-2.01509295357732E-16,-1.09696551146029,
0.587725284610304));
#41773=CARTESIAN_POINT('',(-2.01509295357732E-16,-1.09696551146029,0.));
#41774=CARTESIAN_POINT('Origin',(0.95,-0.548482755730145,0.));
#41775=CARTESIAN_POINT('',(0.95,0.548482755730144,0.587725284610304));
#41776=CARTESIAN_POINT('',(0.95,0.548482755730144,0.));
#41777=CARTESIAN_POINT('Ctrl Pts',(0.95,0.548482755730144,0.587725284610304));
#41778=CARTESIAN_POINT('Ctrl Pts',(0.95,-7.7715611723761E-16,0.746058617943637));
#41779=CARTESIAN_POINT('Ctrl Pts',(0.95,-0.548482755730145,0.587725284610304));
#41780=CARTESIAN_POINT('Origin',(0.95,0.548482755730144,0.));
#41781=CARTESIAN_POINT('',(6.71697651192441E-17,1.09696551146029,0.587725284610304));
#41782=CARTESIAN_POINT('',(6.71697651192441E-17,1.09696551146029,0.));
#41783=CARTESIAN_POINT('Ctrl Pts',(6.71697651192441E-17,1.09696551146029,
0.587725284610304));
#41784=CARTESIAN_POINT('Ctrl Pts',(0.475,0.822724133595216,0.746058617943637));
#41785=CARTESIAN_POINT('Ctrl Pts',(0.95,0.548482755730144,0.587725284610304));
#41786=CARTESIAN_POINT('Origin',(0.,0.,0.629428885575411));
#41787=CARTESIAN_POINT('',(-0.95,0.548482755730144,0.587725284610304));
#41788=CARTESIAN_POINT('Ctrl Pts',(-0.95,0.548482755730144,0.587725284610304));
#41789=CARTESIAN_POINT('Ctrl Pts',(-0.475,0.822724133595217,0.746058617943637));
#41790=CARTESIAN_POINT('Ctrl Pts',(6.71697651192441E-17,1.09696551146029,
0.587725284610304));
#41791=CARTESIAN_POINT('',(-0.95,-7.07449864324762E-17,0.672575862213493));
#41792=CARTESIAN_POINT('Ctrl Pts',(-0.95,-2.51485269459538E-17,0.672575862213493));
#41793=CARTESIAN_POINT('Ctrl Pts',(-0.95,0.254551732809567,0.672575862213493));
#41794=CARTESIAN_POINT('Ctrl Pts',(-0.95,0.548482755730144,0.587725284610304));
#41795=CARTESIAN_POINT('',(-0.9025,-1.10524373623049E-16,0.7));
#41796=CARTESIAN_POINT('',(-1.02473275573014,-1.25493568928637E-16,0.629428885575411));
#41797=CARTESIAN_POINT('Origin',(0.,0.,0.7));
#41798=CARTESIAN_POINT('',(-0.95,-0.548482755730145,0.587725284610304));
#41799=CARTESIAN_POINT('Ctrl Pts',(-0.95,-0.548482755730145,0.587725284610304));
#41800=CARTESIAN_POINT('Ctrl Pts',(-0.95,-0.254551732809567,0.672575862213493));
#41801=CARTESIAN_POINT('Ctrl Pts',(-0.95,-2.51485269459538E-17,0.672575862213493));
#41802=CARTESIAN_POINT('Ctrl Pts',(-2.01509295357732E-16,-1.09696551146029,
0.587725284610304));
#41803=CARTESIAN_POINT('Ctrl Pts',(-0.475,-0.822724133595217,0.746058617943637));
#41804=CARTESIAN_POINT('Ctrl Pts',(-0.95,-0.548482755730145,0.587725284610304));
#41805=CARTESIAN_POINT('Origin',(6.71697651192441E-17,1.09696551146029,
0.));
#41806=CARTESIAN_POINT('',(-0.95,0.548482755730144,0.));
#41807=CARTESIAN_POINT('Origin',(0.,0.,0.7));
#41808=CARTESIAN_POINT('Origin',(0.,0.,0.7));
#41809=CARTESIAN_POINT('',(-0.3,3.67394039744206E-17,0.7));
#41810=CARTESIAN_POINT('Origin',(0.,0.,0.7));
#41811=CARTESIAN_POINT('Origin',(0.,0.,0.));
#41812=CARTESIAN_POINT('',(-0.56785,6.95415684895825E-17,0.));
#41813=CARTESIAN_POINT('Origin',(0.,0.,0.));
#41814=CARTESIAN_POINT('Origin',(0.,0.,0.));
#41815=CARTESIAN_POINT('',(-0.3,-3.67394039744206E-17,0.));
#41816=CARTESIAN_POINT('Origin',(0.,0.,0.));
#41817=CARTESIAN_POINT('Origin',(-0.95,-0.548482755730145,0.));
#41818=CARTESIAN_POINT('',(-0.95,-0.548482755730145,0.));
#41819=CARTESIAN_POINT('Origin',(-0.95,0.548482755730144,0.));
#41820=CARTESIAN_POINT('Origin',(0.,0.,0.0765832901469392));
#41821=CARTESIAN_POINT('',(-0.3,-3.67394039744206E-17,-0.8));
#41822=CARTESIAN_POINT('',(-0.3,-3.67394039744206E-17,0.0765832901469392));
#41823=CARTESIAN_POINT('Origin',(0.,0.,-0.8));
#41824=CARTESIAN_POINT('Origin',(0.,0.,0.0765832901469392));
#41825=CARTESIAN_POINT('',(-0.3,-3.67394039744206E-17,0.953166580293878));
#41826=CARTESIAN_POINT('Origin',(0.,0.,0.953166580293878));
#41827=CARTESIAN_POINT('',(-0.3,-3.67394039744206E-17,0.0765832901469392));
#41828=CARTESIAN_POINT('Origin',(0.57785,0.,-0.8));
#41829=CARTESIAN_POINT('',(-0.57785,-7.07662152887298E-17,-0.8));
#41830=CARTESIAN_POINT('Origin',(0.,0.,-0.8));
#41831=CARTESIAN_POINT('Origin',(0.,0.,-0.76));
#41832=CARTESIAN_POINT('',(-0.61785,-7.56648024853192E-17,-0.76));
#41833=CARTESIAN_POINT('Origin',(0.56785,0.,-0.12));
#41834=CARTESIAN_POINT('',(-0.56785,-6.95415684895825E-17,-0.12));
#41835=CARTESIAN_POINT('Origin',(0.,0.,-0.12));
#41836=CARTESIAN_POINT('Origin',(0.,0.,-0.0349999999999999));
#41837=CARTESIAN_POINT('',(-0.56785,-6.95415684895825E-17,-0.0349999999999999));
#41838=CARTESIAN_POINT('Origin',(0.,0.,1.77));
#41839=CARTESIAN_POINT('',(-0.64,-7.83773951454306E-17,1.8));
#41840=CARTESIAN_POINT('Origin',(0.,0.,1.8));
#41841=CARTESIAN_POINT('',(-0.67,-8.20513355428727E-17,1.77));
#41842=CARTESIAN_POINT('Origin',(0.48,0.,1.8));
#41843=CARTESIAN_POINT('',(-0.48,-5.8783046359073E-17,1.8));
#41844=CARTESIAN_POINT('Origin',(0.,0.,1.8));
#41845=CARTESIAN_POINT('Origin',(0.,0.,1.37658329014694));
#41846=CARTESIAN_POINT('',(-0.39,-4.77612251667468E-17,1.37658329014694));
#59169=UNCERTAINTY_MEASURE_WITH_UNIT(LENGTH_MEASURE(0.001),#59205,
'DISTANCE_ACCURACY_VALUE',
'Maximum model space distance between geometric entities at asserted c
onnectivities');
#59182=UNCERTAINTY_MEASURE_WITH_UNIT(LENGTH_MEASURE(0.001),#59205,
'DISTANCE_ACCURACY_VALUE',
'Maximum model space distance between geometric entities at asserted c
onnectivities');
#59191=(
GEOMETRIC_REPRESENTATION_CONTEXT(3)
GLOBAL_UNCERTAINTY_ASSIGNED_CONTEXT((#59169))
GLOBAL_UNIT_ASSIGNED_CONTEXT((#59205,#59207,#59208))
REPRESENTATION_CONTEXT('','3D')
);
#59204=(
GEOMETRIC_REPRESENTATION_CONTEXT(3)
GLOBAL_UNCERTAINTY_ASSIGNED_CONTEXT((#59182))
GLOBAL_UNIT_ASSIGNED_CONTEXT((#59205,#59207,#59208))
REPRESENTATION_CONTEXT('','3D')
);
#59205=(
LENGTH_UNIT()
NAMED_UNIT(*)
SI_UNIT(.CENTI.,.METRE.)
);
#59207=(
NAMED_UNIT(*)
PLANE_ANGLE_UNIT()
SI_UNIT($,.RADIAN.)
);
#59208=(
NAMED_UNIT(*)
SI_UNIT($,.STERADIAN.)
SOLID_ANGLE_UNIT()
);
#59217=SHAPE_DEFINITION_REPRESENTATION(#59238,#59304);
#59238=PRODUCT_DEFINITION_SHAPE('',$,#59326);
#59304=SHAPE_REPRESENTATION('',(#23491),#59191);
#59317=PRODUCT_DEFINITION_CONTEXT('part definition',#59382,'design');
#59326=PRODUCT_DEFINITION('2026-10-23-00-47-48-451',
'19_Case_Drain_Fitting_DIN_2353_GE08-LR_G1-4',#59347,#59317);
#59347=PRODUCT_DEFINITION_FORMATION('',$,#59392);
#59382=APPLICATION_CONTEXT(
'Core Data for Automotive Mechanical Design Process');
#59383=PRODUCT_CONTEXT('part definition',#59382,'mechanical');
#59392=PRODUCT('2026-10-23-00-47-48-451',
'19_Case_Drain_Fitting_DIN_2353_GE08-LR_G1-4',$,(#59383));
#59566=COLOUR_RGB('Light Blue',0.38,0.62,0.78);
#59567=FILL_AREA_STYLE_COLOUR('',#59566);
#59568=FILL_AREA_STYLE('',(#59567));
#59569=SURFACE_STYLE_FILL_AREA(#59568);
#59570=SURFACE_SIDE_STYLE('',(#59569));
#59571=SURFACE_STYLE_USAGE(.BOTH.,#59570);
#59572=PRESENTATION_STYLE_ASSIGNMENT((#59571));
ENDSEC;
END-ISO-10303-21;
